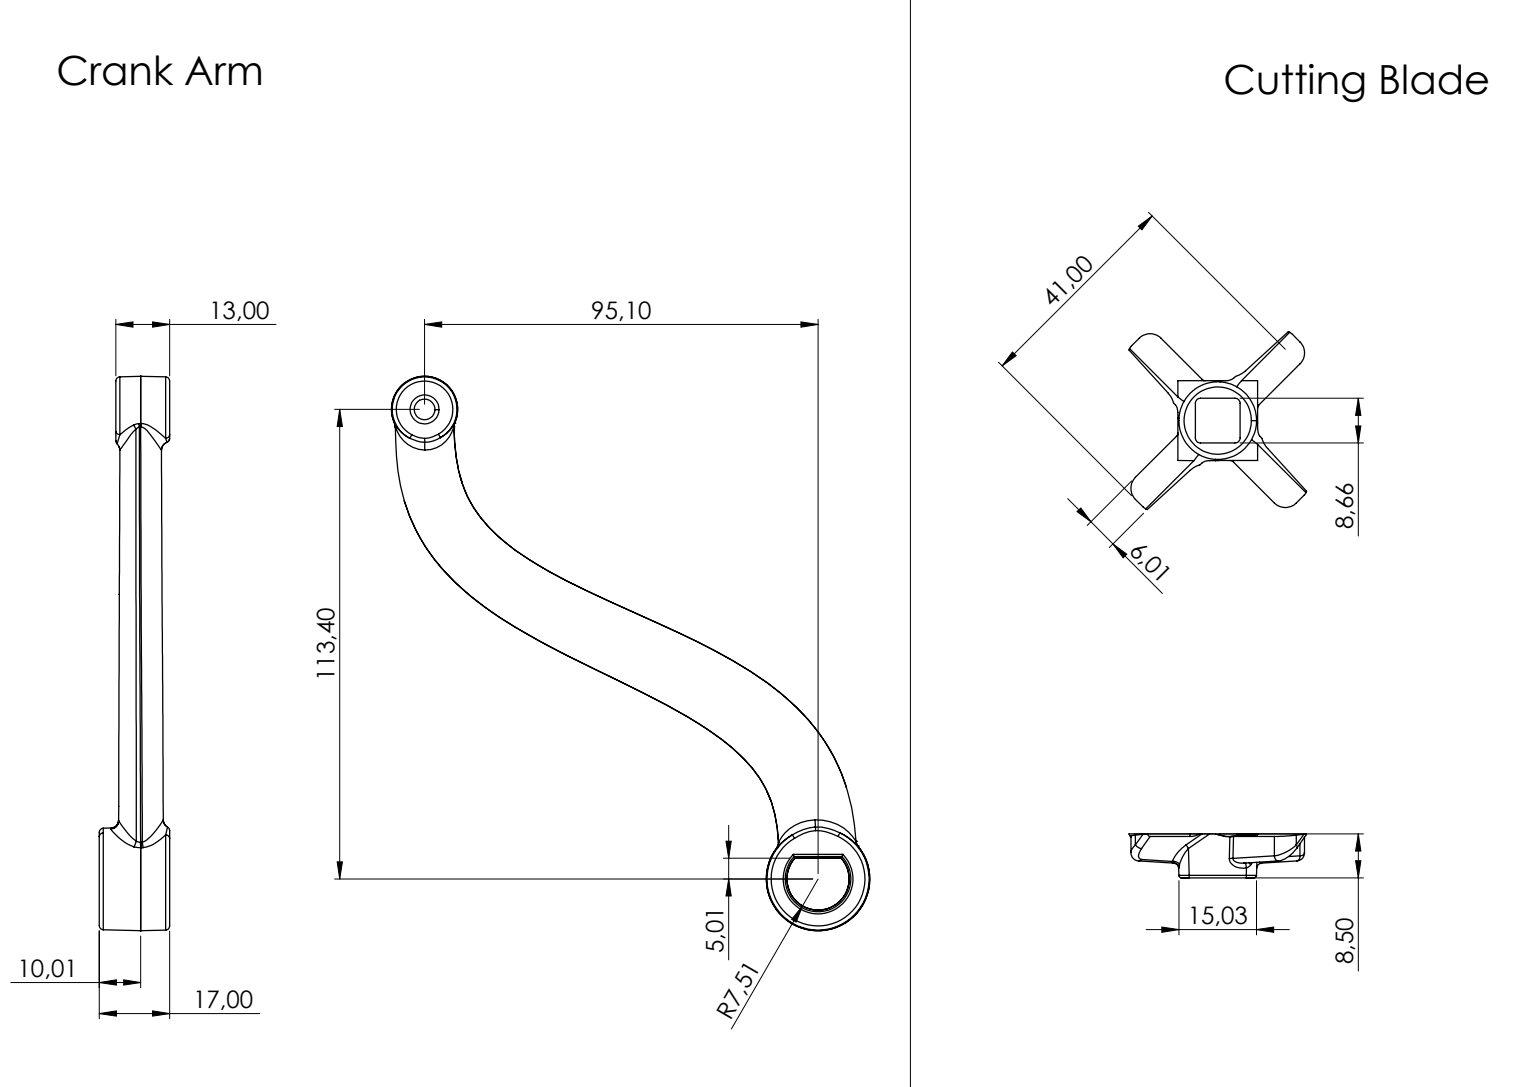
ISO-10303-21;
HEADER;
FILE_DESCRIPTION (('STEP AP214'),
    '1' );
FILE_NAME ('Cutting Blade.step',
    '2026-10-06T09:49:54',
    ( '' ),
    ( '' ),
    'SwSTEP 2.0',
    'SolidWorks 2020',
    '' );
FILE_SCHEMA (( 'AUTOMOTIVE_DESIGN' ));
ENDSEC;

DATA;
#16=CARTESIAN_POINT ( 'NONE',  ( 1.715361092244999996, 1516.743010792419909, 212.5670474586069929 ) ) ;
#21=B_SPLINE_CURVE_WITH_KNOTS ( 'NONE', 3,
 ( #95105, #62085, #88907, #54776, #87831, #29014 ),
 .UNSPECIFIED., .F., .F.,
 ( 4, 2, 4 ),
 ( 0.000000000000000000, 0.5000000000000000000, 1.000000000000000000 ),
 .UNSPECIFIED. ) ;
#54=CARTESIAN_POINT ( 'NONE',  ( -1.906561575282239904E-08, 1509.051704408389924, 204.1347675157070114 ) ) ;
#56=CARTESIAN_POINT ( 'NONE',  ( -6.391938843916317836, 1508.551704408389696, 216.1347674408802106 ) ) ;
#61=CARTESIAN_POINT ( 'NONE',  ( 2.477373605864999995, 1516.891731298979948, 206.2406231745169976 ) ) ;
#69=CARTESIAN_POINT ( 'NONE',  ( -16.59156838405375112, 1513.042027792487033, 221.1339923359998352 ) ) ;
#75=CARTESIAN_POINT ( 'NONE',  ( -5.770883602015000058, 1516.603620185149794, 211.4160555996369908 ) ) ;
#77=EDGE_CURVE ( 'NONE', #86690, #11573, #16701, .T. ) ;
#86=EDGE_CURVE ( 'NONE', #1893, #51148, #21, .T. ) ;
#111=CARTESIAN_POINT ( 'NONE',  ( 6.939219482805000005, 1516.783701990830195, 203.3409846960470020 ) ) ;
#112=CARTESIAN_POINT ( 'NONE',  ( 5.786847739675000213, 1517.104497701820037, 209.8595134730280165 ) ) ;
#115=CARTESIAN_POINT ( 'NONE',  ( 3.849857897463838885, 1511.509056589855390, 217.2694430494650248 ) ) ;
#143=AXIS2_PLACEMENT_3D ( 'NONE', #57309, #48343, #30414 ) ;
#150=CARTESIAN_POINT ( 'NONE',  ( -15.65821252386499829, 1513.518111364920060, 223.8216251916669819 ) ) ;
#156=CARTESIAN_POINT ( 'NONE',  ( -2.881222795715000284, 1516.891731298979948, 206.6444723262370076 ) ) ;
#179=CARTESIAN_POINT ( 'NONE',  ( -13.16128167722848552, 1513.520077403203913, 192.3341213175320092 ) ) ;
#180=EDGE_CURVE ( 'NONE', #17368, #18936, #5451, .T. ) ;
#186=DIRECTION ( 'NONE',  ( -1.000000000000000000, 0.000000000000000000, 0.000000000000000000 ) ) ;
#207=CARTESIAN_POINT ( 'NONE',  ( -5.006329619514999330, 1516.755758396839838, 202.5714564999769891 ) ) ;
#219=EDGE_CURVE ( 'NONE', #44996, #39203, #32843, .T. ) ;
#233=CARTESIAN_POINT ( 'NONE',  ( 7.300066962235000290, 1513.142795523620180, 201.9269575992269949 ) ) ;
#236=ORIENTED_EDGE ( 'NONE', *, *, #47228, .T. ) ;
#243=CARTESIAN_POINT ( 'NONE',  ( -7.886135186697788235, 1512.218159651028827, 212.0631589305448301 ) ) ;
#250=CARTESIAN_POINT ( 'NONE',  ( -4.043990345725000601, 1516.983612918759945, 206.6425990843970055 ) ) ;
#256=CARTESIAN_POINT ( 'NONE',  ( 7.213837368615000578, 1512.784460098860109, 215.9877155789269807 ) ) ;
#266=CARTESIAN_POINT ( 'NONE',  ( 7.720650135305000994, 1516.977993847330026, 214.9014730243169993 ) ) ;
#268=CARTESIAN_POINT ( 'NONE',  ( 6.161099242332739756, 1511.774605969369986, 217.7619246857520068 ) ) ;
#269=CARTESIAN_POINT ( 'NONE',  ( 7.260544162646080046, 1508.878901399440110, 215.8879859943839961 ) ) ;
#270=CARTESIAN_POINT ( 'NONE',  ( 3.268859396054999866, 1516.922519270759949, 211.5998327024669834 ) ) ;
#289=CARTESIAN_POINT ( 'NONE',  ( 2.482067860225000366, 1517.099836525840146, 203.3337487049469985 ) ) ;
#304=LINE ( 'NONE', #17034, #54663 ) ;
#309=CARTESIAN_POINT ( 'NONE',  ( -4.487249408019919450, 1509.038630944639863, 212.6094330731689865 ) ) ;
#315=DIRECTION ( 'NONE',  ( 0.2720708970484284062, 0.6839977328998089190, 0.6768489701308448847 ) ) ;
#316=CARTESIAN_POINT ( 'NONE',  ( -8.788316527315000570, 1511.741868877540128, 215.3741124244170067 ) ) ;
#323=VERTEX_POINT ( 'NONE', #26651 ) ;
#339=CARTESIAN_POINT ( 'NONE',  ( -5.441672317485815036, 1511.126521620285303, 201.4186169187619839 ) ) ;
#370=CARTESIAN_POINT ( 'NONE',  ( -1.703779643355000095, 1517.057265928030120, 213.1670284501570052 ) ) ;
#378=CARTESIAN_POINT ( 'NONE',  ( -3.264778817514999876, 1516.727068157269969, 204.1245957781970048 ) ) ;
#381=CARTESIAN_POINT ( 'NONE',  ( -1.569161292555000031, 1517.051704408389924, 216.8444262845069943 ) ) ;
#393=CARTESIAN_POINT ( 'NONE',  ( 0.7576635334400020350, 1516.855632454399938, 211.9899581013969794 ) ) ;
#398=CARTESIAN_POINT ( 'NONE',  ( -2.881325412095000260, 1517.003078582959688, 208.0029426616869728 ) ) ;
#414=CARTESIAN_POINT ( 'NONE',  ( -7.325541825264999751, 1516.710692850270107, 214.1269169785269924 ) ) ;
#417=CARTESIAN_POINT ( 'NONE',  ( -3.259729335964999919, 1517.119374999550018, 216.4589997383470177 ) ) ;
#444=CARTESIAN_POINT ( 'NONE',  ( -9.638115897704999213, 1520.551704408390151, 203.7504991310570119 ) ) ;
#449=CARTESIAN_POINT ( 'NONE',  ( -2.759740495412019712, 1516.551695078709827, 201.4123589199890034 ) ) ;
#455=ORIENTED_EDGE ( 'NONE', *, *, #105774, .T. ) ;
#493=CARTESIAN_POINT ( 'NONE',  ( 6.949703334655000120, 1517.130100026000036, 209.8609679372960102 ) ) ;
#502=CARTESIAN_POINT ( 'NONE',  ( -14.94819997777649867, 1513.870294663139930, 223.8775307694120045 ) ) ;
#510=CARTESIAN_POINT ( 'NONE',  ( -6.952166420425000659, 1517.213554313520035, 207.4130983078469797 ) ) ;
#525=CARTESIAN_POINT ( 'NONE',  ( -1.715361130375000043, 1516.743010792419909, 205.6766444437269854 ) ) ;
#543=LINE ( 'NONE', #53148, #67817 ) ;
#571=CARTESIAN_POINT ( 'NONE',  ( -3.254401441735000233, 1516.919782530640077, 213.1645757730269963 ) ) ;
#598=VERTEX_POINT ( 'NONE', #85321 ) ;
#605=DIRECTION ( 'NONE',  ( -1.000000000000000000, -6.997424008300000075E-18, -1.832339962680000039E-19 ) ) ;
#607=CARTESIAN_POINT ( 'NONE',  ( -5.385523200472070116, 1511.435001055929888, 200.4690698413500058 ) ) ;
#612=CARTESIAN_POINT ( 'NONE',  ( -3.461995196814999787, 1516.906233342200039, 206.2559344154570056 ) ) ;
#625=CARTESIAN_POINT ( 'NONE',  ( -1.700706814495000163, 1516.923170579120097, 211.4225755968969906 ) ) ;
#632=CARTESIAN_POINT ( 'NONE',  ( 3.052975896485000007, 1516.551704408390151, 217.1245693350269903 ) ) ;
#655=CARTESIAN_POINT ( 'NONE',  ( -4.618119704395000191, 1516.706638732659940, 202.1845071865270143 ) ) ;
#656=CARTESIAN_POINT ( 'NONE',  ( -6.556851034704999748, 1516.939568781210028, 209.1335575761840175 ) ) ;
#659=CARTESIAN_POINT ( 'NONE',  ( 4.264166330254295367, 1511.427938673519748, 217.4025041547218109 ) ) ;
#667=CARTESIAN_POINT ( 'NONE',  ( -0.4363688680027120181, 1517.051704408389924, 216.7663257121729998 ) ) ;
#671=VECTOR ( 'NONE', #63207, 1000.000000000000000 ) ;
#693=CARTESIAN_POINT ( 'NONE',  ( -15.60002308836500085, 1512.080583811389943, 221.9287863060669963 ) ) ;
#698=CARTESIAN_POINT ( 'NONE',  ( 7.708770007014999592, 1516.524310051880093, 206.8307984429870032 ) ) ;
#715=CARTESIAN_POINT ( 'NONE',  ( -2.385772222184999958, 1512.160709093490141, 201.5273412906769863 ) ) ;
#720=CARTESIAN_POINT ( 'NONE',  ( -7.500000019065006462, 1516.813460996586855, 209.5490843734590385 ) ) ;
#748=CARTESIAN_POINT ( 'NONE',  ( 4.031142351675000235, 1516.929569650079884, 204.1114229688670036 ) ) ;
#750=CARTESIAN_POINT ( 'NONE',  ( 15.09629032713499974, 1514.287526756679881, 193.8365223143670164 ) ) ;
#757=ORIENTED_EDGE ( 'NONE', *, *, #107789, .F. ) ;
#773=CARTESIAN_POINT ( 'NONE',  ( -4.027051443935000030, 1516.733363207009916, 211.6130343286269806 ) ) ;
#776=CARTESIAN_POINT ( 'NONE',  ( 7.248946776565000860, 1514.005261957179982, 201.2133402509770121 ) ) ;
#782=CARTESIAN_POINT ( 'NONE',  ( -8.664447134935000960, 1512.053281741910041, 215.6822705669570155 ) ) ;
#785=CARTESIAN_POINT ( 'NONE',  ( 7.717505752974999744, 1516.857914730730045, 216.8393517232070167 ) ) ;
#792=CARTESIAN_POINT ( 'NONE',  ( 3.446329775655000205, 1516.812046502680005, 206.2422037788969931 ) ) ;
#798=CARTESIAN_POINT ( 'NONE',  ( 7.665825164484999732, 1514.407352313670117, 214.8849219750870247 ) ) ;
#804=CARTESIAN_POINT ( 'NONE',  ( 7.487063056100070391, 1517.051702153270071, 209.5621714086410066 ) ) ;
#805=EDGE_CURVE ( 'NONE', #71147, #96332, #85826, .T. ) ;
#809=CARTESIAN_POINT ( 'NONE',  ( 0.7560907277860019482, 1516.770163853809890, 214.1221759657669850 ) ) ;
#814=CARTESIAN_POINT ( 'NONE',  ( 4.625359524845000792, 1517.025470194390209, 211.6020329869469947 ) ) ;
#824=TOROIDAL_SURFACE ( 'NONE', #91997, 6.500000000000000000, 1.000000000000000000 ) ;
#831=CARTESIAN_POINT ( 'NONE',  ( -4.039897316195000698, 1516.787536375099990, 204.1233307748069876 ) ) ;
#878=EDGE_CURVE ( 'NONE', #23166, #598, #93399, .T. ) ;
#892=ORIENTED_EDGE ( 'NONE', *, *, #53861, .T. ) ;
#899=DIRECTION ( 'NONE',  ( 0.9980966414074828874, 0.06164810140419229451, 0.001614312349211199796 ) ) ;
#915=CARTESIAN_POINT ( 'NONE',  ( -4.029572678834999699, 1516.858649670339901, 213.1633184439769764 ) ) ;
#918=EDGE_CURVE ( 'NONE', #68939, #6679, #17776, .T. ) ;
#923=CARTESIAN_POINT ( 'NONE',  ( 2.868433798504999910, 1517.020727862619879, 204.1095288638669842 ) ) ;
#926=CARTESIAN_POINT ( 'NONE',  ( -7.644479542047480258, 1517.051704408389924, 208.6854770967850072 ) ) ;
#938=CARTESIAN_POINT ( 'NONE',  ( 4.042729802795000715, 1516.919782530640077, 212.3762473738369749 ) ) ;
#943=CARTESIAN_POINT ( 'NONE',  ( 2.480427254505000345, 1516.872851364150165, 208.3639601402670110 ) ) ;
#960=CARTESIAN_POINT ( 'NONE',  ( 1.712644716155000024, 1516.636036526019780, 214.1174694231270053 ) ) ;
#963=CARTESIAN_POINT ( 'NONE',  ( -7.716878941104999612, 1516.833976295079992, 216.4517711926369827 ) ) ;
#990=EDGE_CURVE ( 'NONE', #18936, #89283, #17213, .T. ) ;
#997=CARTESIAN_POINT ( 'NONE',  ( -1.079555022276609932, 1516.642200982659915, 201.4099888424200060 ) ) ;
#1038=CARTESIAN_POINT ( 'NONE',  ( -7.601092437462869889, 1510.855104182140167, 214.7738715786570083 ) ) ;
#1045=CARTESIAN_POINT ( 'NONE',  ( -3.255809902135000211, 1516.837969789639828, 209.8792719553279937 ) ) ;
#1059=CARTESIAN_POINT ( 'NONE',  ( -0.7533003905399979772, 1516.992029636990083, 208.3816250717139837 ) ) ;
#1076=CARTESIAN_POINT ( 'NONE',  ( 2.477986732234999767, 1516.922519270759949, 205.8529865360470126 ) ) ;
#1123=CARTESIAN_POINT ( 'NONE',  ( -2.865911554774999814, 1516.906233342200039, 212.5838411289170153 ) ) ;
#1138=DIRECTION ( 'NONE',  ( -0.9147450530333530727, 0.03449475076686789321, 0.4025563316115395862 ) ) ;
#1154=EDGE_CURVE ( 'NONE', #30294, #42497, #37115, .T. ) ;
#1166=CARTESIAN_POINT ( 'NONE',  ( -6.563254928984999736, 1517.139039350860003, 206.6385234782069915 ) ) ;
#1173=CARTESIAN_POINT ( 'NONE',  ( 13.08147543293499915, 1513.492015765619954, 222.9104281842669764 ) ) ;
#1174=ORIENTED_EDGE ( 'NONE', *, *, #86900, .F. ) ;
#1179=CARTESIAN_POINT ( 'NONE',  ( -4.027697264044999947, 1516.766397346390022, 212.0005392193770035 ) ) ;
#1205=CARTESIAN_POINT ( 'NONE',  ( -4.037378294184999383, 1516.688761843659904, 202.5730239910470232 ) ) ;
#1206=CARTESIAN_POINT ( 'NONE',  ( 4.618583391875000110, 1516.939762005280045, 209.1087859301640322 ) ) ;
#1217=CARTESIAN_POINT ( 'NONE',  ( -0.4354997994421860308, 1517.051704408389924, 216.8053818660609977 ) ) ;
#1241=CARTESIAN_POINT ( 'NONE',  ( -15.56957305056499941, 1512.571022561239943, 222.6873122058669878 ) ) ;
#1245=CARTESIAN_POINT ( 'NONE',  ( -1.136004312195000088, 1516.815173273089840, 206.2562091229970065 ) ) ;
#1251=CARTESIAN_POINT ( 'NONE',  ( -10.25304834626500039, 1513.301704408390151, 214.4251468100669911 ) ) ;
#1262=CARTESIAN_POINT ( 'NONE',  ( -2.564633821555000193, 1511.308638870219966, 201.5496530815769916 ) ) ;
#1284=B_SPLINE_CURVE_WITH_KNOTS ( 'NONE', 3,
 ( #68712, #35081, #51899, #102816, #69263, #9338 ),
 .UNSPECIFIED., .F., .F.,
 ( 4, 2, 4 ),
 ( 1.219745810294720132E-06, 0.01184121947742510124, 0.02355703793478339941 ),
 .UNSPECIFIED. ) ;
#1293=FACE_OUTER_BOUND ( 'NONE', #104183, .T. ) ;
#1294=CARTESIAN_POINT ( 'NONE',  ( 2.480813884984999884, 1517.051603658920158, 204.1089070683270279 ) ) ;
#1296=CARTESIAN_POINT ( 'NONE',  ( 16.21240999383499570, 1514.452905717119847, 194.1945360481670093 ) ) ;
#1317=CARTESIAN_POINT ( 'NONE',  ( 6.950214933285000285, 1517.129577905929864, 211.9934263588270085 ) ) ;
#1320=CARTESIAN_POINT ( 'NONE',  ( 6.781132878754999815, 1512.686126173230150, 201.8548505242569888 ) ) ;
#1326=CARTESIAN_POINT ( 'NONE',  ( -7.084879081845000037, 1512.024017243139951, 216.0683601470269934 ) ) ;
#1327=CARTESIAN_POINT ( 'NONE',  ( 16.67556690833916022, 1513.118420042606658, 196.8779830456916216 ) ) ;
#1330=CARTESIAN_POINT ( 'NONE',  ( -6.554778571775000451, 1516.929962200689943, 216.8412383526069789 ) ) ;
#1337=EDGE_LOOP ( 'NONE', ( #26400, #72792, #8720, #28875, #102883, #62231 ) ) ;
#1338=CARTESIAN_POINT ( 'NONE',  ( -2.881222795715000284, 1516.891731298979948, 206.6444723262370076 ) ) ;
#1343=CARTESIAN_POINT ( 'NONE',  ( -7.203718089889590281, 1508.728103933889997, 202.3962606498199932 ) ) ;
#1353=AXIS2_PLACEMENT_3D ( 'NONE', #75150, #16294, #109298 ) ;
#1354=CARTESIAN_POINT ( 'NONE',  ( 7.719392382375000139, 1516.929962200689943, 215.6766245038770080 ) ) ;
#1358=CARTESIAN_POINT ( 'NONE',  ( -7.321193745875000047, 1516.534976163889951, 211.4135222436570132 ) ) ;
#1365=DIRECTION ( 'NONE',  ( -0.7384854939282339270, 4.128709092058512866E-17, 0.6742693640212139572 ) ) ;
#1374=CARTESIAN_POINT ( 'NONE',  ( -5.007588685045000432, 1516.804776704140068, 203.3466091393569855 ) ) ;
#1427=CARTESIAN_POINT ( 'NONE',  ( 7.522201442634911750, 1510.631883379783403, 203.2096215414982510 ) ) ;
#1448=CARTESIAN_POINT ( 'NONE',  ( 0.7564342142240020328, 1516.783665406140017, 213.7345173100169973 ) ) ;
#1449=CARTESIAN_POINT ( 'NONE',  ( 3.276907026574999993, 1511.440441732939917, 216.8388625892569905 ) ) ;
#1461=CARTESIAN_POINT ( 'NONE',  ( 2.288357407604999949, 1517.116049120239950, 203.3334095979369920 ) ) ;
#1479=CARTESIAN_POINT ( 'NONE',  ( -3.446329813785000251, 1516.812046502680005, 212.0014881234369852 ) ) ;
#1484=CARTESIAN_POINT ( 'NONE',  ( 3.255809864005000165, 1516.837969789639828, 208.3644199470059846 ) ) ;
#1494=B_SPLINE_CURVE_WITH_KNOTS ( 'NONE', 5,
 ( #71750, #95254, #20722, #61140, #62230, #54918 ),
 .UNSPECIFIED., .F., .F.,
 ( 6, 6 ),
 ( 0.000000000000000000, 1.000000000000000000 ),
 .UNSPECIFIED. ) ;
#1502=CARTESIAN_POINT ( 'NONE',  ( 3.262264650305000124, 1516.633288330999903, 215.6694029015669969 ) ) ;
#1514=CARTESIAN_POINT ( 'NONE',  ( 7.518184181947409783, 1510.874996213040049, 203.1087175251330166 ) ) ;
#1558=ADVANCED_FACE ( 'NONE', ( #55461 ), #67926, .T. ) ;
#1588=CARTESIAN_POINT ( 'NONE',  ( -7.713648872314999849, 1516.710624944440042, 209.8745175203999906 ) ) ;
#1606=CARTESIAN_POINT ( 'NONE',  ( -5.013429394184999666, 1517.123342927159911, 207.9998951881570122 ) ) ;
#1612=DIRECTION ( 'NONE',  ( -1.000000000000000000, 0.000000000000000000, 0.000000000000000000 ) ) ;
#1625=CARTESIAN_POINT ( 'NONE',  ( -6.949574985774999547, 1517.102359858469754, 205.8627441332170065 ) ) ;
#1628=CARTESIAN_POINT ( 'NONE',  ( -5.018135829431690453, 1516.818301249122669, 203.5289603568284065 ) ) ;
#1646=CARTESIAN_POINT ( 'NONE',  ( 6.946748518954999341, 1516.983995446890049, 214.1250666973070054 ) ) ;
#1673=CARTESIAN_POINT ( 'NONE',  ( 4.041472473744999405, 1516.858649670339901, 213.1514186109370144 ) ) ;
#1721=CARTESIAN_POINT ( 'NONE',  ( 2.282622912365000367, 1516.861367446839949, 206.8218623544969716 ) ) ;
#1735=CARTESIAN_POINT ( 'NONE',  ( 1.716392741775000008, 1516.788317650260069, 211.9856338259669997 ) ) ;
#1760=CARTESIAN_POINT ( 'NONE',  ( 5.513240533218949579, 1508.551563895499839, 201.9548267187850001 ) ) ;
#1764=CARTESIAN_POINT ( 'NONE',  ( -7.719392420504999741, 1516.929962200689943, 202.5670673984569703 ) ) ;
#1765=CARTESIAN_POINT ( 'NONE',  ( 0.01012488564660149991, 1516.989863902050047, 210.2497743036369968 ) ) ;
#1771=LINE ( 'NONE', #96358, #74990 ) ;
#1802=CARTESIAN_POINT ( 'NONE',  ( 11.25155670613500014, 1512.842772631639946, 225.3231501446670109 ) ) ;
#1806=CARTESIAN_POINT ( 'NONE',  ( -16.38335856736500062, 1512.258183966690012, 220.9924808180670084 ) ) ;
#1811=CARTESIAN_POINT ( 'NONE',  ( -5.012317106364999830, 1517.020727862619879, 206.2534121335969814 ) ) ;
#1816=DIRECTION ( 'NONE',  ( 0.000000000000000000, -1.000000000000000000, 3.531714064933559186E-16 ) ) ;
#1828=CARTESIAN_POINT ( 'NONE',  ( -2.229731647334999955, 1512.142919181319940, 201.5278066827870020 ) ) ;
#1831=CARTESIAN_POINT ( 'NONE',  ( 17.14950075666149587, 1517.051704408389924, 222.8506259189660170 ) ) ;
#1864=CARTESIAN_POINT ( 'NONE',  ( 7.324914918154999732, 1516.685667699390024, 204.5043554653269950 ) ) ;
#1886=CARTESIAN_POINT ( 'NONE',  ( -0.7355686809059980291, 1517.012231669750008, 212.3888856620870058 ) ) ;
#1893=VERTEX_POINT ( 'NONE', #110668 ) ;
#1894=VERTEX_POINT ( 'NONE', #27773 ) ;
#1900=CARTESIAN_POINT ( 'NONE',  ( 7.550503318189189628, 1510.480349263560129, 203.5706572562480119 ) ) ;
#1908=CARTESIAN_POINT ( 'NONE',  ( 5.771797426184999580, 1516.647618671360078, 206.2459958378869942 ) ) ;
#1911=AXIS2_PLACEMENT_3D ( 'NONE', #63244, #45873, #62132 ) ;
#1914=CARTESIAN_POINT ( 'NONE',  ( -6.766176630772359424, 1508.878902422570036, 201.8612697231370134 ) ) ;
#1920=CARTESIAN_POINT ( 'NONE',  ( -14.49568595290499928, 1514.921196705999819, 193.9190483465280010 ) ) ;
#1921=CARTESIAN_POINT ( 'NONE',  ( 17.05226155321927095, 1516.729020916208583, 222.6134475786040525 ) ) ;
#1925=CARTESIAN_POINT ( 'NONE',  ( 0.01289778877310149806, 1516.939723362869927, 214.1281058189269970 ) ) ;
#1927=CARTESIAN_POINT ( 'NONE',  ( 6.247704779676360509, 1510.876154134890157, 216.5661308656380015 ) ) ;
#1929=CARTESIAN_POINT ( 'NONE',  ( 2.493073829755000137, 1516.826109302209943, 211.9861720575370043 ) ) ;
#1938=PLANE ( 'NONE',  #73670 ) ;
#1946=CARTESIAN_POINT ( 'NONE',  ( 5.000083827734999709, 1516.858456333729919, 204.1129977322069919 ) ) ;
#1948=VECTOR ( 'NONE', #101539, 1000.000000000000114 ) ;
#1991=CARTESIAN_POINT ( 'NONE',  ( -5.004442077115000664, 1516.690345681169902, 201.4087281291169802 ) ) ;
#1995=CARTESIAN_POINT ( 'NONE',  ( 8.126234247455000670, 1514.923664147150021, 215.2485921136969864 ) ) ;
#2004=CARTESIAN_POINT ( 'NONE',  ( -8.463742342545000241, 1511.382391139620040, 213.9463409611770146 ) ) ;
#2018=ORIENTED_EDGE ( 'NONE', *, *, #878, .T. ) ;
#2023=CARTESIAN_POINT ( 'NONE',  ( 2.490245914424999985, 1516.691389976299888, 213.7302634767470124 ) ) ;
#2024=CARTESIAN_POINT ( 'NONE',  ( 4.036380747524999535, 1511.355055856609852, 217.1076883285369945 ) ) ;
#2025=AXIS2_PLACEMENT_3D ( 'NONE', #103889, #7617, #68656 ) ;
#2031=CARTESIAN_POINT ( 'NONE',  ( 5.000083827734999709, 1516.858456333729919, 204.1129977322069919 ) ) ;
#2046=CARTESIAN_POINT ( 'NONE',  ( 0.7574259850960020080, 1516.837969789639828, 212.3776558342370038 ) ) ;
#2051=CARTESIAN_POINT ( 'NONE',  ( 4.623892060624999800, 1517.066898074209803, 209.8584071487349831 ) ) ;
#2067=CARTESIAN_POINT ( 'NONE',  ( 2.487103419534999915, 1516.577434278289957, 215.6681487122470173 ) ) ;
#2078=CARTESIAN_POINT ( 'NONE',  ( 7.658720530103260593, 1511.445028088800200, 203.0218979614350019 ) ) ;
#2079=PRODUCT_DEFINITION_CONTEXT ( 'detailed design', #26278, 'design' ) ;
#2081=DIRECTION ( 'NONE',  ( 0.6742693640208961003, 0.000000000000000000, 0.7384854939285241393 ) ) ;
#2090=CARTESIAN_POINT ( 'NONE',  ( 6.520293444144174444, 1509.032998982614345, 201.8615402263750127 ) ) ;
#2105=EDGE_CURVE ( 'NONE', #33006, #74270, #109360, .T. ) ;
#2108=CARTESIAN_POINT ( 'NONE',  ( -1.951485868198830076, 1516.530904812869949, 201.4129032351939657 ) ) ;
#2156=ORIENTED_EDGE ( 'NONE', *, *, #106868, .F. ) ;
#2157=CARTESIAN_POINT ( 'NONE',  ( -1.122033430074999893, 1516.972341476009888, 209.8777854684929878 ) ) ;
#2161=VECTOR ( 'NONE', #110428, 1000.000000000000114 ) ;
#2174=CARTESIAN_POINT ( 'NONE',  ( 6.938478784765000462, 1516.719999691880048, 208.3679751968140010 ) ) ;
#2178=ORIENTED_EDGE ( 'NONE', *, *, #38568, .F. ) ;
#2184=CARTESIAN_POINT ( 'NONE',  ( 6.541070334811199594, 1517.051704644130041, 212.7912326336579838 ) ) ;
#2191=CARTESIAN_POINT ( 'NONE',  ( -7.336844680545000053, 1517.106845464700200, 205.6683011064770312 ) ) ;
#2210=CARTESIAN_POINT ( 'NONE',  ( -6.549762485114999144, 1516.729202374750002, 213.7405950387170037 ) ) ;
#2211=CARTESIAN_POINT ( 'NONE',  ( -4.329791528864999961, 1515.051704408389924, 212.4519801359869859 ) ) ;
#2228=CARTESIAN_POINT ( 'NONE',  ( 6.499999980935001531, 1516.051704408390151, 209.1218459511669892 ) ) ;
#2270=FACE_OUTER_BOUND ( 'NONE', #4358, .T. ) ;
#2285=CARTESIAN_POINT ( 'NONE',  ( -5.013274999515000552, 1517.068517094990057, 206.8347616620369820 ) ) ;
#2297=CARTESIAN_POINT ( 'NONE',  ( -3.445685115514999897, 1516.778761582560037, 211.6139765934069885 ) ) ;
#2307=CARTESIAN_POINT ( 'NONE',  ( 14.86633461655332233, 1514.624327954312776, 225.3233414037949842 ) ) ;
#2324=CARTESIAN_POINT ( 'NONE',  ( -1.130607502004999931, 1516.632821972880038, 202.5736453444569918 ) ) ;
#2325=CARTESIAN_POINT ( 'NONE',  ( -3.253301419385000504, 1516.790374942449944, 210.2573062871869922 ) ) ;
#2329=ORIENTED_EDGE ( 'NONE', *, *, #108317, .F. ) ;
#2346=CARTESIAN_POINT ( 'NONE',  ( -7.779264728704999854, 1514.199187793449937, 202.4059200890270063 ) ) ;
#2359=EDGE_CURVE ( 'NONE', #5115, #10547, #107935, .T. ) ;
#2371=CARTESIAN_POINT ( 'NONE',  ( -0.7576635715699989726, 1516.855632454399938, 206.2537338009369989 ) ) ;
#2373=DIRECTION ( 'NONE',  ( 0.000000000000000000, -1.000000000000000000, 6.123233995736769734E-17 ) ) ;
#2390=CARTESIAN_POINT ( 'NONE',  ( 5.857434645806802287, 1510.600498174433824, 216.6525474564166416 ) ) ;
#2404=EDGE_CURVE ( 'NONE', #19958, #1894, #81618, .T. ) ;
#2424=CARTESIAN_POINT ( 'NONE',  ( 7.323974606304999746, 1516.647924054489977, 205.0857262875869935 ) ) ;
#2446=CARTESIAN_POINT ( 'NONE',  ( 6.561995960394999550, 1517.083030555940013, 212.3803205491769859 ) ) ;
#2467=CARTESIAN_POINT ( 'NONE',  ( -7.338411997524999286, 1517.170512887980067, 206.6372682748769876 ) ) ;
#2473=CARTESIAN_POINT ( 'NONE',  ( -6.961854465055609786, 1508.551568319609714, 202.5699773954310103 ) ) ;
#2485=CARTESIAN_POINT ( 'NONE',  ( -6.552897405075000847, 1516.858146885269889, 215.6784973415170157 ) ) ;
#2489=CARTESIAN_POINT ( 'NONE',  ( -1.118903308544999975, 1517.003078582959688, 212.0031713441969998 ) ) ;
#2505=CARTESIAN_POINT ( 'NONE',  ( 4.612507273904999039, 1516.886345593249871, 204.1123678647870179 ) ) ;
#2521=CARTESIAN_POINT ( 'NONE',  ( -5.513435911474870110, 1508.551704408389924, 202.1089243664339961 ) ) ;
#2522=CIRCLE ( 'NONE', #40049, 5.000000000000000888 ) ;
#2545=DIRECTION ( 'NONE',  ( 0.000000000000000000, 1.000000000000000000, -6.123233995736769734E-17 ) ) ;
#2547=CARTESIAN_POINT ( 'NONE',  ( 3.259729297834999873, 1517.119374999550018, 201.7846921639870175 ) ) ;
#2562=CARTESIAN_POINT ( 'NONE',  ( -7.548380910495000151, 1510.399296111369949, 213.9269235281369959 ) ) ;
#2581=CARTESIAN_POINT ( 'NONE',  ( 0.01289778877310149806, 1516.939723362869927, 214.1281058189269970 ) ) ;
#2582=CARTESIAN_POINT ( 'NONE',  ( 2.933667421895000516, 1512.215430505229961, 217.0052628094269949 ) ) ;
#2587=CARTESIAN_POINT ( 'NONE',  ( 4.998515157294999511, 1516.787536375099990, 205.0819486540370065 ) ) ;
#2589=CARTESIAN_POINT ( 'NONE',  ( -3.415238448984999842, 1511.775527460079957, 205.7066075212470082 ) ) ;
#2590=CARTESIAN_POINT ( 'NONE',  ( 5.004475574535000248, 1517.026025493960105, 201.3999380438669959 ) ) ;
#2601=CARTESIAN_POINT ( 'NONE',  ( 4.043366220174999803, 1516.951766529250108, 211.9887038632370206 ) ) ;
#2607=CARTESIAN_POINT ( 'NONE',  ( 7.724874613184999461, 1517.139320148880188, 209.8621665372610039 ) ) ;
#2621=CARTESIAN_POINT ( 'NONE',  ( 0.01244693565920149993, 1516.939646076049939, 214.9034317483770167 ) ) ;
#2631=CARTESIAN_POINT ( 'NONE',  ( 7.899080318006880930, 1511.275365984429982, 203.5511717028010139 ) ) ;
#2639=DIRECTION ( 'NONE',  ( -0.6742693640212139572, -4.521919481779819710E-17, -0.7384854939282339270 ) ) ;
#2645=DIRECTION ( 'NONE',  ( -0.7071067811865492381, 0.000000000000000000, -0.7071067811865457964 ) ) ;
#2662=CARTESIAN_POINT ( 'NONE',  ( -2.000106894569579907, 1516.529320347400244, 201.4129447258819994 ) ) ;
#2706=CARTESIAN_POINT ( 'NONE',  ( 0.01012488564660149991, 1516.989863902050047, 210.2497743036369968 ) ) ;
#2708=B_SPLINE_CURVE_WITH_KNOTS ( 'NONE', 3,
 ( #29885, #55678, #22008, #65718, #23130, #6348, #29339, #63540, #97656, #20926, #49469, #60081, #25881, #23687, #57872, #109375, #68482, #179, #109911, #100404, #58416, #17468, #92002, #7447, #42158, #51118, #41045, #101480, #51669, #94197, #24231, #85805, #8538, #93634, #66287, #85242, #32652, #16369, #75223, #102583, #92542, #9103, #76310, #15276, #24768, #43270, #110460, #108807, #50567, #83589 ),
 .UNSPECIFIED., .F., .F.,
 ( 4, 2, 2, 1, 1, 2, 2, 2, 2, 1, 1, 1, 2, 2, 2, 2, 1, 1, 1, 2, 2, 2, 2, 1, 1, 1, 1, 2, 2, 2, 4 ),
 ( 0.000000000000000000, 0.1249999999987768118, 0.1874999999981652177, 0.2187499999978483323, 0.2343749999976874887, 0.2421874999976066367, 0.2499999999975258125, 0.3749999999967162934, 0.4374999999962853603, 0.4687499999960699770, 0.4843749999959355845, 0.4921874999958685826, 0.4960937499958351093, 0.4999999999958015806, 0.6249999999951432184, 0.6874999999948141483, 0.7187499999946499463, 0.7343749999945659024, 0.7421874999945267115, 0.7460937499945041740, 0.7499999999944817475, 0.8124999999947372098, 0.8437499999948295804, 0.8593749999948757656, 0.8671874999948987472, 0.8710937499949140683, 0.8730468749949186202, 0.8740234374949206186, 0.8749999999949225060, 0.9374999999974612530, 1.000000000000000000 ),
 .UNSPECIFIED. ) ;
#2712=EDGE_LOOP ( 'NONE', ( #76998, #67436, #41942, #17145, #20832, #42478, #88108, #19322, #74311 ) ) ;
#2720=VERTEX_POINT ( 'NONE', #85468 ) ;
#2722=CARTESIAN_POINT ( 'NONE',  ( 3.255809864005000165, 1516.837969789639828, 208.3644199470059846 ) ) ;
#2739=CARTESIAN_POINT ( 'NONE',  ( -2.493699806765000027, 1516.858326417339867, 206.6451124560869914 ) ) ;
#2749=CARTESIAN_POINT ( 'NONE',  ( -7.821732098484999618, 1513.613303996360173, 201.3872288444869980 ) ) ;
#2756=CARTESIAN_POINT ( 'NONE',  ( 3.456007385174999946, 1516.647534046129977, 215.6697273451470096 ) ) ;
#2758=ORIENTED_EDGE ( 'NONE', *, *, #78090, .T. ) ;
#2802=CARTESIAN_POINT ( 'NONE',  ( 7.599227146675000100, 1512.341036988540054, 206.8869224911269953 ) ) ;
#2820=CARTESIAN_POINT ( 'NONE',  ( -5.783578535681273003, 1516.788854543809975, 213.9010045776934419 ) ) ;
#2823=DIRECTION ( 'NONE',  ( -0.4770263929453174567, 0.7067418228236591604, -0.5224574779878943254 ) ) ;
#2825=CARTESIAN_POINT ( 'NONE',  ( 2.864326087304999824, 1516.826109302209943, 206.6287721023469999 ) ) ;
#2829=CARTESIAN_POINT ( 'NONE',  ( 15.20279577643499991, 1516.814170398969964, 225.0317485278669949 ) ) ;
#2836=CARTESIAN_POINT ( 'NONE',  ( 1.136004274065000041, 1516.815173273089840, 211.9874827793370287 ) ) ;
#2845=CARTESIAN_POINT ( 'NONE',  ( 11.97297233184965570, 1513.029502680773930, 225.6983645998317058 ) ) ;
#2847=ORIENTED_EDGE ( 'NONE', *, *, #49017, .T. ) ;
#2848=ORIENTED_EDGE ( 'NONE', *, *, #54124, .T. ) ;
#2856=CARTESIAN_POINT ( 'NONE',  ( 6.455447949027460552, 1508.551704612109916, 202.2941920603649919 ) ) ;
#2861=EDGE_CURVE ( 'NONE', #93671, #44996, #6366, .T. ) ;
#2864=VERTEX_POINT ( 'NONE', #72042 ) ;
#2865=CARTESIAN_POINT ( 'NONE',  ( 7.324914918154999732, 1516.685667699390024, 204.5043554653269950 ) ) ;
#2870=ORIENTED_EDGE ( 'NONE', *, *, #97880, .F. ) ;
#2891=CARTESIAN_POINT ( 'NONE',  ( -7.573276867445001059, 1513.355826799089755, 201.2778793177070042 ) ) ;
#2901=VERTEX_POINT ( 'NONE', #12649 ) ;
#2916=CARTESIAN_POINT ( 'NONE',  ( 2.863787855735000054, 1516.788317650260069, 207.4054531903269947 ) ) ;
#2935=CARTESIAN_POINT ( 'NONE',  ( 5.963459866581566793, 1510.663752950224307, 216.6350338863308309 ) ) ;
#2938=CARTESIAN_POINT ( 'NONE',  ( 17.10989499766859367, 1517.051704408389924, 222.9504516956734506 ) ) ;
#2956=ADVANCED_FACE ( 'NONE', ( #92651 ), #32751, .F. ) ;
#2972=CARTESIAN_POINT ( 'NONE',  ( 7.712490952985000980, 1516.666407245520077, 204.5049844236870058 ) ) ;
#2992=CARTESIAN_POINT ( 'NONE',  ( 6.561686423234999843, 1517.069378699710114, 212.5741351528070027 ) ) ;
#3003=CARTESIAN_POINT ( 'NONE',  ( -7.316722043595000002, 1511.382498894329956, 215.7022088808070066 ) ) ;
#3012=CARTESIAN_POINT ( 'NONE',  ( -4.811461170099283535, 1516.551188146009054, 218.2487618711105313 ) ) ;
#3014=CARTESIAN_POINT ( 'NONE',  ( 0.7350231981660010350, 1516.970035769810011, 206.8242163110469960 ) ) ;
#3025=CARTESIAN_POINT ( 'NONE',  ( 7.717505752974999744, 1516.857914730730045, 201.4043401791270185 ) ) ;
#3033=CARTESIAN_POINT ( 'NONE',  ( -3.259101837015000225, 1517.102359858469754, 216.0714209178769920 ) ) ;
#3037=CARTESIAN_POINT ( 'NONE',  ( 5.949235695344720298, 1511.655824793919919, 217.4114490419000276 ) ) ;
#3039=CARTESIAN_POINT ( 'NONE',  ( 2.492443650904999863, 1516.793978928989873, 212.3737347995770222 ) ) ;
#3040=CARTESIAN_POINT ( 'NONE',  ( 3.330134165755000097, 1515.051704408389924, 213.4516374609670208 ) ) ;
#3043=ORIENTED_EDGE ( 'NONE', *, *, #45218, .T. ) ;
#3055=ORIENTED_EDGE ( 'NONE', *, *, #108341, .F. ) ;
#3056=CARTESIAN_POINT ( 'NONE',  ( -2.877113108595000135, 1516.697242742309982, 204.1252037719370094 ) ) ;
#3069=AXIS2_PLACEMENT_3D ( 'NONE', #84795, #58524, #49027 ) ;
#3094=CARTESIAN_POINT ( 'NONE',  ( -12.61087486066499785, 1512.195694528090144, 194.0417079242670013 ) ) ;
#3097=CARTESIAN_POINT ( 'NONE',  ( -2.872700555325000238, 1516.559109716219837, 201.4121646638069763 ) ) ;
#3102=CARTESIAN_POINT ( 'NONE',  ( 7.575166919095000395, 1511.422242621320265, 206.4203055568870013 ) ) ;
#3106=ORIENTED_EDGE ( 'NONE', *, *, #105951, .T. ) ;
#3111=CARTESIAN_POINT ( 'NONE',  ( -7.848179713114999956, 1511.193640125469983, 213.6447370295169890 ) ) ;
#3132=CARTESIAN_POINT ( 'NONE',  ( -7.325541825264999751, 1516.710692850270107, 214.1269169785269924 ) ) ;
#3133=CARTESIAN_POINT ( 'NONE',  ( 4.813011385984999890, 1510.693074690949970, 216.6779200322870054 ) ) ;
#3138=CARTESIAN_POINT ( 'NONE',  ( -0.01322039564809850132, 1516.939819969850078, 205.0847949345169923 ) ) ;
#3141=CARTESIAN_POINT ( 'NONE',  ( 0.7403205670290020635, 1517.139320148880188, 201.3969713189170250 ) ) ;
#3153=CARTESIAN_POINT ( 'NONE',  ( -4.609996619675000851, 1516.769879638719885, 212.5810025483170023 ) ) ;
#3160=CARTESIAN_POINT ( 'NONE',  ( 0.7533003524100010395, 1516.992029636990083, 209.8620668306199946 ) ) ;
#3173=CARTESIAN_POINT ( 'NONE',  ( -5.777745433405000242, 1516.908489800550115, 215.6797558528670038 ) ) ;
#3179=CARTESIAN_POINT ( 'NONE',  ( 0.7403205670290020635, 1517.139320148880188, 201.3969713189170250 ) ) ;
#3188=CARTESIAN_POINT ( 'NONE',  ( 7.946349138541700441, 1511.532396045849964, 203.1959877047910084 ) ) ;
#3201=DIRECTION ( 'NONE',  ( 0.02616798426500965835, 0.9993150019883683122, -0.02616798426500970692 ) ) ;
#3202=CARTESIAN_POINT ( 'NONE',  ( 4.987078416414999715, 1508.551704408389924, 212.6094384009469707 ) ) ;
#3246=CARTESIAN_POINT ( 'NONE',  ( -7.500000019064998469, 1516.801704408389924, 209.1218459511669892 ) ) ;
#3258=CARTESIAN_POINT ( 'NONE',  ( 1.137296650804999976, 1516.908147884120126, 210.8236964273370120 ) ) ;
#3266=CARTESIAN_POINT ( 'NONE',  ( 5.778999773775000293, 1516.955859323880077, 201.7887757972170277 ) ) ;
#3272=CARTESIAN_POINT ( 'NONE',  ( 1.715109447055000125, 1516.963431999339946, 209.8570730874349977 ) ) ;
#3289=CARTESIAN_POINT ( 'NONE',  ( -2.299656354225000143, 1516.843453247299749, 206.6453952679669896 ) ) ;
#3290=VERTEX_POINT ( 'NONE', #37586 ) ;
#3306=DIRECTION ( 'NONE',  ( -1.000000000000000000, 0.000000000000000000, 0.000000000000000000 ) ) ;
#3308=CARTESIAN_POINT ( 'NONE',  ( 2.874588922665000545, 1516.606339319019980, 215.6687976528169770 ) ) ;
#3331=CYLINDRICAL_SURFACE ( 'NONE', #1911, 0.4999999999999909517 ) ;
#3350=ORIENTED_EDGE ( 'NONE', *, *, #99298, .F. ) ;
#3376=CARTESIAN_POINT ( 'NONE',  ( -0.01323705180209850014, 1516.939658295650133, 206.6356258303270010 ) ) ;
#3386=CARTESIAN_POINT ( 'NONE',  ( 8.753854055680109880, 1516.720891557477444, 213.2732902691849972 ) ) ;
#3397=CARTESIAN_POINT ( 'NONE',  ( 14.31751620109325174, 1514.209381233404883, 225.6439688837686504 ) ) ;
#3407=FACE_BOUND ( 'NONE', #58671, .T. ) ;
#3416=CARTESIAN_POINT ( 'NONE',  ( -3.264778817514999876, 1516.727068157269969, 204.1245957781970048 ) ) ;
#3436=CARTESIAN_POINT ( 'NONE',  ( -6.742834623714999864, 1512.383155430620036, 200.7463434866369880 ) ) ;
#3452=CARTESIAN_POINT ( 'NONE',  ( 14.12475443283500098, 1513.169116394660023, 224.4178625549669732 ) ) ;
#3461=CARTESIAN_POINT ( 'NONE',  ( 1.117840086735000016, 1516.949031626070109, 207.4047068479870006 ) ) ;
#3495=DIRECTION ( 'NONE',  ( -0.5224574779883525144, -0.7067418228232951183, 0.4770263929453549823 ) ) ;
#3502=EDGE_CURVE ( 'NONE', #33889, #21042, #75482, .T. ) ;
#3519=CARTESIAN_POINT ( 'NONE',  ( -2.490245952555000031, 1516.691389976299888, 204.5134284255869943 ) ) ;
#3541=CARTESIAN_POINT ( 'NONE',  ( 2.879956924955000108, 1516.827328999679821, 212.3743765858270081 ) ) ;
#3550=ORIENTED_EDGE ( 'NONE', *, *, #91361, .T. ) ;
#3564=CARTESIAN_POINT ( 'NONE',  ( 3.445201488374999954, 1516.743010792419909, 207.4064848398570291 ) ) ;
#3576=CYLINDRICAL_SURFACE ( 'NONE', #58477, 0.9999999999999522604 ) ;
#3583=CARTESIAN_POINT ( 'NONE',  ( -6.940473372275000052, 1516.833525648419936, 215.6778681647369922 ) ) ;
#3585=CARTESIAN_POINT ( 'NONE',  ( 6.048292005814400518, 1511.681069547209972, 217.7611486164249754 ) ) ;
#3587=CARTESIAN_POINT ( 'NONE',  ( -4.996642198295000448, 1516.697242742309982, 211.9989590406970024 ) ) ;
#3588=CARTESIAN_POINT ( 'NONE',  ( 3.915803383833039941, 1515.051704408389924, 213.4516362061017674 ) ) ;
#3605=CARTESIAN_POINT ( 'NONE',  ( -7.723480117524999855, 1517.086065052259983, 205.0863097070169943 ) ) ;
#3629=VECTOR ( 'NONE', #88330, 1000.000000000000227 ) ;
#3634=( BOUNDED_CURVE ( )  B_SPLINE_CURVE ( 3, ( #36275, #78848, #61504, #11632 ),
 .UNSPECIFIED., .F., .F. ) 
 B_SPLINE_CURVE_WITH_KNOTS ( ( 4, 4 ),
 ( 5.498282993746389735, 7.068394191937580118 ),
 .UNSPECIFIED. ) 
 CURVE ( )  GEOMETRIC_REPRESENTATION_ITEM ( )  RATIONAL_B_SPLINE_CURVE ( ( 1.000000000000000000, 0.8048993128220308657, 0.8048993128220308657, 1.000000000000000000 ) ) 
 REPRESENTATION_ITEM ( '' )  );
#3645=CARTESIAN_POINT ( 'NONE',  ( -14.49215846226499949, 1514.088841912139969, 192.6059998857670053 ) ) ;
#3650=CARTESIAN_POINT ( 'NONE',  ( 1.710012720495000194, 1517.232977404109988, 201.3945188173769907 ) ) ;
#3664=CARTESIAN_POINT ( 'NONE',  ( -7.556166249915000854, 1510.696675236759802, 213.5834717662970093 ) ) ;
#3667=AXIS2_PLACEMENT_3D ( 'NONE', #4462, #79519, #2823 ) ;
#3675=CARTESIAN_POINT ( 'NONE',  ( 15.90990255763500016, 1512.830284628050094, 198.1616908427670296 ) ) ;
#3685=CARTESIAN_POINT ( 'NONE',  ( 3.263521904354999670, 1516.676340709600026, 214.8942497445370066 ) ) ;
#3686=CARTESIAN_POINT ( 'NONE',  ( 3.165841356415000085, 1511.802450769970164, 217.0590624235869939 ) ) ;
#3691=CARTESIAN_POINT ( 'NONE',  ( -2.878693287274999957, 1516.766397346390022, 205.0941487061870134 ) ) ;
#3694=B_SPLINE_SURFACE_WITH_KNOTS ( 'NONE', 5, 5, ( 
 ( #309, #110587, #33873, #74800, #42284, #15953 ),
 ( #17600, #76434, #75890, #50686, #51800, #68609 ),
 ( #85939, #9242, #59652, #66412, #108943, #58000 ),
 ( #68064, #17038, #7027, #24898, #100529, #60203 ),
 ( #102177, #110040, #93760, #23808, #102712, #59105 ),
 ( #92134, #51235, #15409, #83732, #41184, #84283 ) ),
 .UNSPECIFIED., .F., .F., .F.,
 ( 6, 6 ),
 ( 6, 6 ),
 ( 4.250940516431700011, 7.082035122218299783 ),
 ( -9.670478295891639110E-06, 0.5000000000000000000 ),
 .UNSPECIFIED. ) ;
#3698=ORIENTED_EDGE ( 'NONE', *, *, #45621, .F. ) ;
#3704=CARTESIAN_POINT ( 'NONE',  ( 6.560742225334999844, 1517.028034847769959, 213.1554992345569701 ) ) ;
#3710=CARTESIAN_POINT ( 'NONE',  ( -1.709766532154999963, 1516.959716008189844, 209.1345041580460133 ) ) ;
#3719=CARTESIAN_POINT ( 'NONE',  ( 7.499999980935000643, 1516.801704408389924, 209.1218459511669892 ) ) ;
#3725=CARTESIAN_POINT ( 'NONE',  ( 2.488360629304999794, 1516.616791731099966, 214.8929950451170043 ) ) ;
#3729=VERTEX_POINT ( 'NONE', #70805 ) ;
#3730=CARTESIAN_POINT ( 'NONE',  ( -0.01126495432349849946, 1516.939530130779985, 202.1773791897269916 ) ) ;
#3735=CARTESIAN_POINT ( 'NONE',  ( 8.788267567532809466, 1511.742575854359984, 202.8686686809350022 ) ) ;
#3758=CARTESIAN_POINT ( 'NONE',  ( -7.495712400002839004, 1517.016242308364099, 208.8285887136074450 ) ) ;
#3764=CARTESIAN_POINT ( 'NONE',  ( -0.7983437007204670088, 1516.708834472140097, 201.4082439830900171 ) ) ;
#3769=CARTESIAN_POINT ( 'NONE',  ( 12.22498599127479935, 1512.125809830880144, 223.8828819965079902 ) ) ;
#3814=CARTESIAN_POINT ( 'NONE',  ( -5.770820179264999794, 1516.591755933730155, 210.8331571987770019 ) ) ;
#3822=EDGE_CURVE ( 'NONE', #89306, #3290, #97423, .T. ) ;
#3823=CARTESIAN_POINT ( 'NONE',  ( 3.259729297834999873, 1517.119374999550018, 201.7846921639870175 ) ) ;
#3838=AXIS2_PLACEMENT_3D ( 'NONE', #66963, #14317, #56898 ) ;
#3844=CARTESIAN_POINT ( 'NONE',  ( -1.136004312195000088, 1516.815173273089840, 206.2562091229970065 ) ) ;
#3852=CARTESIAN_POINT ( 'NONE',  ( 6.372167600494999640, 1511.069621805459974, 216.5183910133270047 ) ) ;
#3860=CARTESIAN_POINT ( 'NONE',  ( -4.612507312034999529, 1516.886345593249871, 214.1313240375470173 ) ) ;
#3862=ORIENTED_EDGE ( 'NONE', *, *, #70755, .F. ) ;
#3879=DIRECTION ( 'NONE',  ( 0.7063774289747313251, 0.04540766091858271930, -0.7063774289747313251 ) ) ;
#3881=CARTESIAN_POINT ( 'NONE',  ( -5.513435705061030312, 1509.038615938849944, 201.6090957135359929 ) ) ;
#3890=CARTESIAN_POINT ( 'NONE',  ( -4.554962026871971048, 1508.731359868796062, 212.6094325583298712 ) ) ;
#3928=CARTESIAN_POINT ( 'NONE',  ( -0.7579263249019989601, 1516.927039499179955, 207.4176752179770347 ) ) ;
#3949=CARTESIAN_POINT ( 'NONE',  ( 14.77683004841523307, 1514.552098284236536, 225.3854720466699462 ) ) ;
#3967=CARTESIAN_POINT ( 'NONE',  ( 1.121383591734999907, 1517.104192383289956, 204.4960559556369901 ) ) ;
#3987=CARTESIAN_POINT ( 'NONE',  ( -6.658917469454999960, 1512.371207877090001, 200.8892782097470047 ) ) ;
#4000=CARTESIAN_POINT ( 'NONE',  ( 13.86270800413499948, 1513.875858217480072, 225.8871191791669730 ) ) ;
#4008=CARTESIAN_POINT ( 'NONE',  ( -2.494758036134999912, 1516.937508036699910, 207.4208181092269854 ) ) ;
#4019=CYLINDRICAL_SURFACE ( 'NONE', #68164, 0.9999999999999985567 ) ;
#4026=CARTESIAN_POINT ( 'NONE',  ( 6.288919081391354027, 1510.947107034761302, 216.5507387054137496 ) ) ;
#4063=CARTESIAN_POINT ( 'NONE',  ( 4.028630584655000568, 1516.812923327049930, 205.6617440802170051 ) ) ;
#4070=ORIENTED_EDGE ( 'NONE', *, *, #85135, .F. ) ;
#4091=ORIENTED_EDGE ( 'NONE', *, *, #25305, .T. ) ;
#4092=CARTESIAN_POINT ( 'NONE',  ( -6.715925881185000001, 1514.199187793469946, 216.9011106608170110 ) ) ;
#4093=CARTESIAN_POINT ( 'NONE',  ( 16.20149547506775534, 1514.624327907797579, 194.2555113716582582 ) ) ;
#4104=CARTESIAN_POINT ( 'NONE',  ( 7.321193707744999557, 1516.534976163889951, 206.8301696586770220 ) ) ;
#4121=CARTESIAN_POINT ( 'NONE',  ( 0.7538707352880020807, 1516.719999691880048, 216.0603247549969979 ) ) ;
#4123=DIRECTION ( 'NONE',  ( 0.8236474686107853049, -0.5669078173018522460, 0.01484500364079644613 ) ) ;
#4125=CARTESIAN_POINT ( 'NONE',  ( 6.561995960394999550, 1517.083030555940013, 212.3803205491769859 ) ) ;
#4143=CARTESIAN_POINT ( 'NONE',  ( -6.559798094425000059, 1516.987478262539980, 204.5068286042669854 ) ) ;
#4165=CARTESIAN_POINT ( 'NONE',  ( 8.389588760568322812, 1511.399594748087793, 204.5238464867746302 ) ) ;
#4170=ADVANCED_FACE ( 'NONE', ( #109599 ), #49705, .T. ) ;
#4175=CARTESIAN_POINT ( 'NONE',  ( -12.07722023366500075, 1511.957228877180114, 194.2728863314669923 ) ) ;
#4177=CARTESIAN_POINT ( 'NONE',  ( 2.872208710164999790, 1517.145312756229941, 201.7840522196070197 ) ) ;
#4181=CARTESIAN_POINT ( 'NONE',  ( 7.684243075114999932, 1511.930588878439949, 206.3551010095970071 ) ) ;
#4188=CARTESIAN_POINT ( 'NONE',  ( -4.487249791936469556, 1509.038615938009798, 212.6094384014929801 ) ) ;
#4189=CARTESIAN_POINT ( 'NONE',  ( -4.616861546623686863, 1516.666407247929328, 201.4093550276068072 ) ) ;
#4206=VERTEX_POINT ( 'NONE', #57562 ) ;
#4214=CARTESIAN_POINT ( 'NONE',  ( -5.775236830874999505, 1516.804776704140068, 214.1294346171470124 ) ) ;
#4221=CARTESIAN_POINT ( 'NONE',  ( -1.713317447804999949, 1516.660388280709867, 204.5138242629670060 ) ) ;
#4234=CARTESIAN_POINT ( 'NONE',  ( -6.935457963315000640, 1516.627618683580067, 212.5772239474869991 ) ) ;
#4239=CARTESIAN_POINT ( 'NONE',  ( -7.714148301377419692, 1516.729697371079965, 209.8385372711610160 ) ) ;
#4240=EDGE_CURVE ( 'NONE', #49508, #63015, #65316, .T. ) ;
#4241=CARTESIAN_POINT ( 'NONE',  ( 5.786847739675000213, 1517.104497701820037, 209.8595134730280165 ) ) ;
#4257=CARTESIAN_POINT ( 'NONE',  ( 3.261635932824999973, 1516.613881697390070, 216.0569793506570022 ) ) ;
#4262=CARTESIAN_POINT ( 'NONE',  ( 7.716878902974999122, 1516.833976295079992, 201.7919207096969672 ) ) ;
#4263=CARTESIAN_POINT ( 'NONE',  ( -14.84895963876499891, 1511.957228877180114, 221.1990661657670216 ) ) ;
#4265=CARTESIAN_POINT ( 'NONE',  ( -15.91746622356501462, 1512.594959757389915, 220.0895646873669875 ) ) ;
#4288=EDGE_CURVE ( 'NONE', #37685, #65412, #87722, .T. ) ;
#4300=CARTESIAN_POINT ( 'NONE',  ( 0.04106552329005089957, 1516.946282269519997, 201.4020272027410101 ) ) ;
#4302=ORIENTED_EDGE ( 'NONE', *, *, #103432, .F. ) ;
#4304=CARTESIAN_POINT ( 'NONE',  ( 13.70533112961760125, 1512.850289816029772, 224.4308539454270033 ) ) ;
#4306=ORIENTED_EDGE ( 'NONE', *, *, #42966, .T. ) ;
#4345=CARTESIAN_POINT ( 'NONE',  ( 3.462948796544999652, 1516.956048353049937, 211.4063724288770061 ) ) ;
#4354=CARTESIAN_POINT ( 'NONE',  ( 2.291514297774999598, 1517.194972660189933, 201.3955140066269962 ) ) ;
#4358=EDGE_LOOP ( 'NONE', ( #50228, #35588, #67697, #74405 ) ) ;
#4370=CARTESIAN_POINT ( 'NONE',  ( 0.7559394982620020187, 1516.972341476009888, 210.2438793621770117 ) ) ;
#4375=CARTESIAN_POINT ( 'NONE',  ( 7.717016619025000246, 1511.440441732939917, 205.8449389055269876 ) ) ;
#4377=CARTESIAN_POINT ( 'NONE',  ( 4.995994787574999485, 1516.665179208830068, 206.6322283937570035 ) ) ;
#4378=ORIENTED_EDGE ( 'NONE', *, *, #31531, .F. ) ;
#4379=LINE ( 'NONE', #98415, #97351 ) ;
#4396=CARTESIAN_POINT ( 'NONE',  ( -6.939219520934999608, 1516.783701990830195, 214.9027072062869763 ) ) ;
#4397=ORIENTED_EDGE ( 'NONE', *, *, #51664, .F. ) ;
#4398=CARTESIAN_POINT ( 'NONE',  ( 7.708877363402839578, 1516.528409826940106, 206.8600011716279994 ) ) ;
#4428=CARTESIAN_POINT ( 'NONE',  ( -4.487249791936469556, 1509.038615938009798, 212.6094384014929801 ) ) ;
#4440=CARTESIAN_POINT ( 'NONE',  ( 3.487585849186794817, 1508.611350403810775, 213.8000011204408963 ) ) ;
#4453=CARTESIAN_POINT ( 'NONE',  ( -7.507423057800870048, 1508.880864719049896, 215.2619752906269923 ) ) ;
#4462=CARTESIAN_POINT ( 'NONE',  ( -5.242935297045000276, 1514.496907775670024, 217.7778693727470056 ) ) ;
#4464=CARTESIAN_POINT ( 'NONE',  ( 4.026614479655000522, 1516.699825673279975, 207.4075116849170115 ) ) ;
#4485=CARTESIAN_POINT ( 'NONE',  ( 14.16490606602967084, 1514.105081316843780, 225.7087563701193460 ) ) ;
#4493=CARTESIAN_POINT ( 'NONE',  ( 4.369728359379250193, 1508.879004046169939, 205.0024669094390219 ) ) ;
#4501=CARTESIAN_POINT ( 'NONE',  ( 4.612507273904999039, 1516.886345593249871, 204.1123678647870179 ) ) ;
#4507=ORIENTED_EDGE ( 'NONE', *, *, #75832, .F. ) ;
#4512=CARTESIAN_POINT ( 'NONE',  ( -14.35493914170010044, 1513.426431439620046, 193.9549492499340033 ) ) ;
#4523=CARTESIAN_POINT ( 'NONE',  ( -7.466890204824999877, 1513.600111798330090, 202.4729951676269764 ) ) ;
#4537=CARTESIAN_POINT ( 'NONE',  ( 11.87063484783499945, 1512.258183966700017, 225.5052044994669700 ) ) ;
#4543=CARTESIAN_POINT ( 'NONE',  ( 2.282622912365000367, 1516.861367446839949, 206.8218623544969716 ) ) ;
#4584=CARTESIAN_POINT ( 'NONE',  ( 3.487592431604999987, 1508.551704408389924, 204.1347675156769981 ) ) ;
#4591=CARTESIAN_POINT ( 'NONE',  ( -3.385932610363147077, 1511.683921178999071, 201.1181467729594203 ) ) ;
#4598=CARTESIAN_POINT ( 'NONE',  ( -4.041472511874999896, 1516.858649670339901, 205.0922732913970208 ) ) ;
#4612=CARTESIAN_POINT ( 'NONE',  ( -4.612671377915000370, 1516.783665406140017, 209.8782801844560026 ) ) ;
#4627=CARTESIAN_POINT ( 'NONE',  ( -6.390054486374999954, 1513.333000339850059, 216.6179291409569885 ) ) ;
#4637=CARTESIAN_POINT ( 'NONE',  ( 7.708770007014999592, 1516.524310051880093, 206.8307984429870032 ) ) ;
#4642=ORIENTED_EDGE ( 'NONE', *, *, #48019, .F. ) ;
#4648=CARTESIAN_POINT ( 'NONE',  ( -5.910253173700709795, 1511.600194708689969, 200.4926261112069881 ) ) ;
#4654=CARTESIAN_POINT ( 'NONE',  ( 5.005700201405000271, 1516.732530461250008, 216.0598116305469887 ) ) ;
#4658=CARTESIAN_POINT ( 'NONE',  ( 2.419940912470191829, 1516.533504771425442, 216.8308567494544832 ) ) ;
#4659=CARTESIAN_POINT ( 'NONE',  ( 3.266349474065000091, 1516.797038924770050, 213.1501537103870021 ) ) ;
#4667=EDGE_CURVE ( 'NONE', #106739, #71879, #51778, .T. ) ;
#4677=CARTESIAN_POINT ( 'NONE',  ( 6.547881374914999775, 1516.647534046129977, 205.6658385469270058 ) ) ;
#4700=CARTESIAN_POINT ( 'NONE',  ( 7.924501696547047835, 1511.889619706852500, 206.0091653069858069 ) ) ;
#4706=CARTESIAN_POINT ( 'NONE',  ( -7.513187957268617545, 1510.663752939659162, 215.0853058208080313 ) ) ;
#4709=CARTESIAN_POINT ( 'NONE',  ( -11.59188839696499862, 1512.902436350919970, 192.6803903701670038 ) ) ;
#4712=CARTESIAN_POINT ( 'NONE',  ( -1.708721022705000037, 1516.531533746980131, 201.8006767011069940 ) ) ;
#4746=CARTESIAN_POINT ( 'NONE',  ( -5.001338666445000136, 1516.911981270829983, 214.9058546054269812 ) ) ;
#4754=CARTESIAN_POINT ( 'NONE',  ( 0.7360974386200019870, 1517.045004075700035, 205.0794574309270217 ) ) ;
#4767=CARTESIAN_POINT ( 'NONE',  ( -7.323034312095000331, 1516.609912606490070, 212.5765947784269940 ) ) ;
#4772=CARTESIAN_POINT ( 'NONE',  ( 4.625789976465000564, 1517.104192383289956, 210.2432295619669844 ) ) ;
#4785=CARTESIAN_POINT ( 'NONE',  ( -2.484577695354999616, 1517.170512887980067, 216.4602579296269766 ) ) ;
#4790=CARTESIAN_POINT ( 'NONE',  ( -3.261007169695000041, 1516.596789218710001, 201.7991362452670216 ) ) ;
#4797=CARTESIAN_POINT ( 'NONE',  ( 8.488400859335269999, 1511.451532973539770, 203.7397716954870077 ) ) ;
#4811=FACE_OUTER_BOUND ( 'NONE', #61858, .T. ) ;
#4824=CARTESIAN_POINT ( 'NONE',  ( 0.02465969127001850156, 1516.941612417570013, 201.4021494659330074 ) ) ;
#4829=CARTESIAN_POINT ( 'NONE',  ( 13.03156809012940087, 1512.406412987999829, 224.3505518485380037 ) ) ;
#4873=CARTESIAN_POINT ( 'NONE',  ( 7.339749335215000059, 1517.224900789629828, 210.8312305431869902 ) ) ;
#4875=CARTESIAN_POINT ( 'NONE',  ( 3.461360093275000160, 1516.874084700499907, 212.3753080308970311 ) ) ;
#4883=CARTESIAN_POINT ( 'NONE',  ( -3.261007169695000041, 1516.596789218710001, 201.7991362452670216 ) ) ;
#4884=DIRECTION ( 'NONE',  ( 0.6742693640212154005, 0.000000000000000000, 0.7384854939282328168 ) ) ;
#4898=CARTESIAN_POINT ( 'NONE',  ( -5.775625115495000017, 1516.745833913490060, 209.8771724060850090 ) ) ;
#4904=CARTESIAN_POINT ( 'NONE',  ( 7.548872300095000654, 1510.418062979259958, 203.9404357814470075 ) ) ;
#4906=( BOUNDED_CURVE ( )  B_SPLINE_CURVE ( 3, ( #98180, #56187, #20910, #55115 ),
 .UNSPECIFIED., .F., .F. ) 
 B_SPLINE_CURVE_WITH_KNOTS ( ( 4, 4 ),
 ( 4.424142070125560267, 5.579787944456629845 ),
 .UNSPECIFIED. ) 
 CURVE ( )  GEOMETRIC_REPRESENTATION_ITEM ( )  RATIONAL_B_SPLINE_CURVE ( ( 1.000000000000000000, 0.8917691661789544089, 0.8917691661789544089, 1.000000000000000000 ) ) 
 REPRESENTATION_ITEM ( '' )  );
#4907=CARTESIAN_POINT ( 'NONE',  ( -4.625359562974999506, 1517.025470194390209, 206.6416589153869836 ) ) ;
#4922=CARTESIAN_POINT ( 'NONE',  ( 5.006329581384999727, 1516.755758396839838, 215.6722354023569892 ) ) ;
#4924=CARTESIAN_POINT ( 'NONE',  ( 7.710967333700570414, 1516.608222572569957, 207.8710650191239893 ) ) ;
#4925=CARTESIAN_POINT ( 'NONE',  ( -7.889297536996000559, 1517.051704408390378, 206.4074150262267722 ) ) ;
#4933=CARTESIAN_POINT ( 'NONE',  ( 2.234923440975000286, 1512.341036988540054, 216.7210731169070073 ) ) ;
#4946=VECTOR ( 'NONE', #52550, 1000.000000000000114 ) ;
#4951=CARTESIAN_POINT ( 'NONE',  ( -4.538868782924999401, 1511.336728379370243, 201.0216414995070124 ) ) ;
#4967=DIRECTION ( 'NONE',  ( 0.02616798426500960631, -0.9993150019883682011, -0.02616798426500960631 ) ) ;
#4995=CARTESIAN_POINT ( 'NONE',  ( -7.727327152855000492, 1517.232977404109988, 207.4118332116069894 ) ) ;
#5011=CARTESIAN_POINT ( 'NONE',  ( 7.565983030562289713, 1517.051704408389924, 209.5600921240870207 ) ) ;
#5036=CARTESIAN_POINT ( 'NONE',  ( -6.557909920764999789, 1516.908489800550115, 203.3441005368270282 ) ) ;
#5043=CARTESIAN_POINT ( 'NONE',  ( 4.554961988741982992, 1508.731359868795835, 205.6342593440040503 ) ) ;
#5045=CARTESIAN_POINT ( 'NONE',  ( -14.75568483658040009, 1513.870294662259994, 194.1736459919410152 ) ) ;
#5057=CARTESIAN_POINT ( 'NONE',  ( -7.743766119884999632, 1514.370494773840164, 202.8627129457869955 ) ) ;
#5070=CARTESIAN_POINT ( 'NONE',  ( 14.37690900153499918, 1514.216506490359961, 225.6932579665669891 ) ) ;
#5110=CIRCLE ( 'NONE', #99897, 1.000000000000059064 ) ;
#5115=VERTEX_POINT ( 'NONE', #95839 ) ;
#5118=DIRECTION ( 'NONE',  ( -0.8236474686107847498, 0.5669078173018529121, -0.01484500364079613562 ) ) ;
#5127=CARTESIAN_POINT ( 'NONE',  ( -2.957486053519140956, 1512.146863357693292, 201.2343373090091347 ) ) ;
#5136=CARTESIAN_POINT ( 'NONE',  ( 2.285487581364999965, 1517.001127920769704, 205.0775242521070254 ) ) ;
#5151=CARTESIAN_POINT ( 'NONE',  ( 2.881325373965000214, 1517.003078582959688, 210.2407492406470055 ) ) ;
#5164=CARTESIAN_POINT ( 'NONE',  ( -5.706397885535000825, 1514.325389163589989, 216.7730352073269842 ) ) ;
#5165=CARTESIAN_POINT ( 'NONE',  ( 16.31974134803240872, 1514.485057798524167, 194.4298416830750682 ) ) ;
#5171=CARTESIAN_POINT ( 'NONE',  ( -3.487592469391230132, 1509.038615938009798, 204.6345961782960217 ) ) ;
#5174=CARTESIAN_POINT ( 'NONE',  ( -2.258825589925000266, 1511.942942747529969, 201.5330432499970073 ) ) ;
#5180=CARTESIAN_POINT ( 'NONE',  ( 3.255809864005000165, 1516.837969789639828, 208.3644199470059846 ) ) ;
#5191=CARTESIAN_POINT ( 'NONE',  ( -5.652025646554889704, 1510.855104182140167, 201.5207535327680262 ) ) ;
#5193=CARTESIAN_POINT ( 'NONE',  ( -6.178095865712184498, 1510.835436358435118, 201.6599032209836082 ) ) ;
#5199=VECTOR ( 'NONE', #47929, 1000.000000000000000 ) ;
#5200=CARTESIAN_POINT ( 'NONE',  ( -5.778999811904999895, 1516.955859323880077, 216.4549161051170074 ) ) ;
#5206=CARTESIAN_POINT ( 'NONE',  ( -5.772727946874999461, 1516.691414181030041, 212.5791125756269935 ) ) ;
#5218=B_SPLINE_CURVE_WITH_KNOTS ( 'NONE', 5,
 ( #98225, #73606, #22587, #29913, #39979, #56237 ),
 .UNSPECIFIED., .F., .F.,
 ( 6, 6 ),
 ( 4.250950522270000143, 7.082025451739999866 ),
 .UNSPECIFIED. ) ;
#5225=CARTESIAN_POINT ( 'NONE',  ( -1.714334285315000095, 1516.699825673279975, 205.0952314524469955 ) ) ;
#5254=( BOUNDED_CURVE ( )  B_SPLINE_CURVE ( 3, ( #58994, #16391, #50586, #84716 ),
 .UNSPECIFIED., .F., .T. ) 
 B_SPLINE_CURVE_WITH_KNOTS ( ( 4, 4 ),
 ( 0.5395807524025459934, 1.539014399144550405 ),
 .UNSPECIFIED. ) 
 CURVE ( )  GEOMETRIC_REPRESENTATION_ITEM ( )  RATIONAL_B_SPLINE_CURVE ( ( 1.000000000000000000, 0.9184788592068002799, 0.9184788592068002799, 1.000000000000000000 ) ) 
 REPRESENTATION_ITEM ( '' )  );
#5261=CARTESIAN_POINT ( 'NONE',  ( -7.550503362009299835, 1510.480349264700180, 214.6730346447039892 ) ) ;
#5264=CARTESIAN_POINT ( 'NONE',  ( -11.75640701316500092, 1511.791180387469922, 193.9413991097669907 ) ) ;
#5266=CARTESIAN_POINT ( 'NONE',  ( -6.942973667334999988, 1516.833844030519913, 201.7931697622170191 ) ) ;
#5269=CARTESIAN_POINT ( 'NONE',  ( 15.90990255763500016, 1512.830284628050094, 198.1616908427670296 ) ) ;
#5293=CARTESIAN_POINT ( 'NONE',  ( 7.380526832584999752, 1511.503799556579906, 202.6426608137470282 ) ) ;
#5303=CARTESIAN_POINT ( 'NONE',  ( 0.7538707352880020807, 1516.719999691880048, 216.0603247549969979 ) ) ;
#5311=CARTESIAN_POINT ( 'NONE',  ( 4.997573787194999895, 1516.742629295279812, 205.6633194342169872 ) ) ;
#5313=CARTESIAN_POINT ( 'NONE',  ( 4.037050997585000189, 1516.939819969850078, 209.1086255745840106 ) ) ;
#5317=CARTESIAN_POINT ( 'NONE',  ( 6.527830543224999893, 1512.220794350770120, 216.8989209840169963 ) ) ;
#5325=CARTESIAN_POINT ( 'NONE',  ( 5.785582913545000316, 1516.981965530290154, 213.1542438721070027 ) ) ;
#5330=CARTESIAN_POINT ( 'NONE',  ( -7.708877905894440552, 1516.528429087750055, 211.1705659669590034 ) ) ;
#5331=CARTESIAN_POINT ( 'NONE',  ( 4.045182479925000685, 1517.057265928030120, 210.8256255754569963 ) ) ;
#5343=CARTESIAN_POINT ( 'NONE',  ( 7.550503318189189628, 1510.480349263560129, 203.5706572562480119 ) ) ;
#5346=CARTESIAN_POINT ( 'NONE',  ( -1.125509888415000104, 1517.203017563489766, 216.4609531728469847 ) ) ;
#5351=CARTESIAN_POINT ( 'NONE',  ( -6.942344729965000738, 1516.810037859429940, 201.4055938791270250 ) ) ;
#5353=VERTEX_POINT ( 'NONE', #67760 ) ;
#5358=CARTESIAN_POINT ( 'NONE',  ( 7.551708674585110082, 1510.523965798400013, 203.3918062713489974 ) ) ;
#5375=AXIS2_PLACEMENT_3D ( 'NONE', #34462, #94922, #43974 ) ;
#5380=CARTESIAN_POINT ( 'NONE',  ( -13.72878287234173555, 1517.051704408389924, 226.2713469440930112 ) ) ;
#5386=CARTESIAN_POINT ( 'NONE',  ( -0.4165852338731970139, 1516.813354641049955, 201.4055070984510110 ) ) ;
#5390=CARTESIAN_POINT ( 'NONE',  ( 14.92122229814569856, 1514.080593477150160, 223.9397791912049911 ) ) ;
#5410=ADVANCED_FACE ( 'NONE', ( #101873 ), #50955, .F. ) ;
#5431=CARTESIAN_POINT ( 'NONE',  ( 2.494757998004999866, 1516.937508036699910, 210.8228737931069929 ) ) ;
#5434=CARTESIAN_POINT ( 'NONE',  ( -7.323034312095000331, 1516.609912606490070, 212.5765947784269940 ) ) ;
#5440=CARTESIAN_POINT ( 'NONE',  ( 5.778372563615000068, 1516.932669162149978, 202.1763558832970205 ) ) ;
#5451=LINE ( 'NONE', #23883, #107492 ) ;
#5452=CARTESIAN_POINT ( 'NONE',  ( -3.669386717783980068, 1517.051704642929963, 215.6629163041010031 ) ) ;
#5455=CARTESIAN_POINT ( 'NONE',  ( 2.493697040924999886, 1516.977201124959947, 210.2401991861970032 ) ) ;
#5460=CARTESIAN_POINT ( 'NONE',  ( 8.558300736974999268, 1511.397837225850026, 204.0148718853070022 ) ) ;
#5461=CARTESIAN_POINT ( 'NONE',  ( 5.770820141135000192, 1516.591755933730155, 207.4105347035570048 ) ) ;
#5473=CARTESIAN_POINT ( 'NONE',  ( 7.627638999635267147, 1513.425324099864838, 215.5670651928058703 ) ) ;
#5477=CARTESIAN_POINT ( 'NONE',  ( 4.987078416394999714, 1508.551704408389924, 209.1218459511669892 ) ) ;
#5479=CARTESIAN_POINT ( 'NONE',  ( -7.715625241105000143, 1516.786099423779888, 215.6766101314970001 ) ) ;
#5481=CARTESIAN_POINT ( 'NONE',  ( 7.709070221419720426, 1516.535774777470124, 206.6432696383980101 ) ) ;
#5494=B_SPLINE_SURFACE_WITH_KNOTS ( 'NONE', 5, 5, ( 
 ( #3735, #88267, #86601, #12101, #44063, #2078, #36758, #45737, #35646 ),
 ( #46295, #80422, #18829, #37867, #3188, #11560, #78201, #37316, #27252 ),
 ( #61434, #97205, #53024, #103382, #61990, #54139, #10449, #1514, #44622 ),
 ( #71511, #53585, #105630, #28915, #78763, #104511, #105067, #96106, #19381 ),
 ( #26687, #36208, #27806, #87731, #2631, #11009, #45180, #73122, #5358 ),
 ( #99399, #4797, #22124, #65286, #5917, #107819, #99953, #89907, #38942 ) ),
 .UNSPECIFIED., .F., .F., .F.,
 ( 6, 6 ),
 ( 6, 3, 6 ),
 ( 4.238752792101340816, 5.659133035208659734 ),
 ( 0.000000000000000000, 0.5000000000000000000, 1.002061266618659907 ),
 .UNSPECIFIED. ) ;
#5507=AXIS2_PLACEMENT_3D ( 'NONE', #74613, #107651, #66229 ) ;
#5525=ORIENTED_EDGE ( 'NONE', *, *, #219, .F. ) ;
#5526=EDGE_CURVE ( 'NONE', #51148, #42643, #78925, .T. ) ;
#5529=FACE_OUTER_BOUND ( 'NONE', #43506, .T. ) ;
#5545=CARTESIAN_POINT ( 'NONE',  ( -7.512750272569109988, 1509.038617475950105, 214.6350457578409987 ) ) ;
#5560=CARTESIAN_POINT ( 'NONE',  ( 2.477975315464999717, 1516.839862955080207, 207.9852983471170091 ) ) ;
#5588=ORIENTED_EDGE ( 'NONE', *, *, #102639, .F. ) ;
#5594=ORIENTED_EDGE ( 'NONE', *, *, #22009, .T. ) ;
#5598=CARTESIAN_POINT ( 'NONE',  ( 2.866857893004999713, 1516.951766529250108, 205.0784797119270024 ) ) ;
#5603=ORIENTED_EDGE ( 'NONE', *, *, #74145, .F. ) ;
#5606=CYLINDRICAL_SURFACE ( 'NONE', #96725, 2.999999999999995115 ) ;
#5607=CARTESIAN_POINT ( 'NONE',  ( -13.18795888012849993, 1512.495155157840145, 193.8533315336999863 ) ) ;
#5623=CARTESIAN_POINT ( 'NONE',  ( -5.614653854145000622, 1512.956339156650074, 214.7364997862470091 ) ) ;
#5633=CARTESIAN_POINT ( 'NONE',  ( 14.45097768893499968, 1514.857962383129916, 224.3693530530669875 ) ) ;
#5647=VECTOR ( 'NONE', #2639, 1000.000000000000114 ) ;
#5687=PLANE ( 'NONE',  #110541 ) ;
#5688=SURFACE_SIDE_STYLE ('',( #90215 ) ) ;
#5702=CARTESIAN_POINT ( 'NONE',  ( -2.879642191334999879, 1516.812046502680005, 205.6755161564470313 ) ) ;
#5716=CARTESIAN_POINT ( 'NONE',  ( 7.339749335215000059, 1517.224900789629828, 210.8312305431869902 ) ) ;
#5730=CARTESIAN_POINT ( 'NONE',  ( -5.986375141904999531, 1514.050458741980037, 216.7582919984769774 ) ) ;
#5744=CARTESIAN_POINT ( 'NONE',  ( 7.716878902974999122, 1516.833976295079992, 201.7919207096969672 ) ) ;
#5745=CARTESIAN_POINT ( 'NONE',  ( 0.7402208603880020554, 1516.992029636990083, 208.3685455796920110 ) ) ;
#5759=CARTESIAN_POINT ( 'NONE',  ( -5.912224502460420084, 1510.631883423287263, 201.5996445015462371 ) ) ;
#5764=CARTESIAN_POINT ( 'NONE',  ( 2.291676273424999799, 1516.534976163889951, 216.4430396779769978 ) ) ;
#5769=CARTESIAN_POINT ( 'NONE',  ( 1.135185044044999980, 1516.778853242349896, 212.5689744308569971 ) ) ;
#5790=CARTESIAN_POINT ( 'NONE',  ( -6.948321743994999800, 1517.049325831759916, 205.0875650164470017 ) ) ;
#5818=CARTESIAN_POINT ( 'NONE',  ( 7.508706873624496403, 1508.884207225577484, 203.6084103738515978 ) ) ;
#5831=CARTESIAN_POINT ( 'NONE',  ( 1.125509850285000280, 1517.203017563489766, 201.7827387294869936 ) ) ;
#5835=CARTESIAN_POINT ( 'NONE',  ( 15.19327421213499996, 1512.300546902530186, 196.2658363013669884 ) ) ;
#5847=CARTESIAN_POINT ( 'NONE',  ( -7.618904794935000169, 1511.873873588870083, 211.7469127400270281 ) ) ;
#5860=ORIENTED_EDGE ( 'NONE', *, *, #36766, .F. ) ;
#5865=CARTESIAN_POINT ( 'NONE',  ( -6.553524415734999664, 1516.882690742909972, 216.0660777183969969 ) ) ;
#5871=CARTESIAN_POINT ( 'NONE',  ( 7.710610402995000001, 1516.594591938570147, 205.6677260153969939 ) ) ;
#5873=CARTESIAN_POINT ( 'NONE',  ( -3.255809902135000211, 1516.837969789639828, 209.8792719553279937 ) ) ;
#5884=CARTESIAN_POINT ( 'NONE',  ( -5.774609660074999873, 1516.777260590120022, 213.7418541773069762 ) ) ;
#5888=CARTESIAN_POINT ( 'NONE',  ( -7.714725160980429486, 1516.751726750540229, 209.7571990288649886 ) ) ;
#5889=CARTESIAN_POINT ( 'NONE',  ( 4.626591867355000609, 1517.096587378560116, 210.8266407735670214 ) ) ;
#5904=CARTESIAN_POINT ( 'NONE',  ( 6.555393117025000826, 1516.809497469189864, 216.4498952504870033 ) ) ;
#5909=CARTESIAN_POINT ( 'NONE',  ( 4.615644804385000022, 1517.009964551830080, 202.1744681489270192 ) ) ;
#5917=CARTESIAN_POINT ( 'NONE',  ( 7.866724121416869941, 1511.219705715099963, 203.6977230978289981 ) ) ;
#5946=CARTESIAN_POINT ( 'NONE',  ( 14.56186259785490122, 1513.645442088340133, 224.1908963721469945 ) ) ;
#5956=CARTESIAN_POINT ( 'NONE',  ( 13.82860585633196848, 1517.051704408389924, 192.0119494921260639 ) ) ;
#5982=CARTESIAN_POINT ( 'NONE',  ( -4.995994825704999975, 1516.665179208830068, 211.6114635085770033 ) ) ;
#5985=CARTESIAN_POINT ( 'NONE',  ( 6.949265646015000186, 1517.089216728169959, 212.5747629931370000 ) ) ;
#5991=CARTESIAN_POINT ( 'NONE',  ( 6.552897366944999469, 1516.858146885269889, 202.5651945608169910 ) ) ;
#6006=CARTESIAN_POINT ( 'NONE',  ( 1.136814033864999907, 1516.854133554269993, 211.4058994415870245 ) ) ;
#6011=CARTESIAN_POINT ( 'NONE',  ( 7.556074062054999985, 1510.693074690949970, 204.3088345461070219 ) ) ;
#6012=CARTESIAN_POINT ( 'NONE',  ( 2.282622912365000367, 1516.861367446839949, 206.8218623544969716 ) ) ;
#6030=CARTESIAN_POINT ( 'NONE',  ( -7.328676208015000526, 1516.833844030519913, 216.0648195994369871 ) ) ;
#6034=CARTESIAN_POINT ( 'NONE',  ( -7.722580352398438208, 1517.051704408390378, 206.9393828551336583 ) ) ;
#6061=CARTESIAN_POINT ( 'NONE',  ( -3.991161821394999976, 1511.207707629420156, 201.3372867307170111 ) ) ;
#6063=CARTESIAN_POINT ( 'NONE',  ( -5.556349349672759175, 1511.457792576462907, 200.4111309786675577 ) ) ;
#6085=DIRECTION ( 'NONE',  ( 1.000000000000000000, 0.000000000000000000, 0.000000000000000000 ) ) ;
#6095=CARTESIAN_POINT ( 'NONE',  ( -7.395102162025949610, 1511.068351247050032, 215.4971964518929894 ) ) ;
#6100=CARTESIAN_POINT ( 'NONE',  ( 3.447128460625000113, 1516.778853242349896, 207.9866608880570027 ) ) ;
#6124=CARTESIAN_POINT ( 'NONE',  ( 4.364199090702369332, 1509.032029411810072, 205.0059829744700153 ) ) ;
#6133=CARTESIAN_POINT ( 'NONE',  ( -6.947377821305000367, 1517.009964551830080, 204.5062011277169916 ) ) ;
#6136=CARTESIAN_POINT ( 'NONE',  ( 15.05672294932299948, 1512.222316757829958, 196.4963374934199862 ) ) ;
#6142=CARTESIAN_POINT ( 'NONE',  ( -12.89209534591269879, 1512.335564144490036, 193.9409293534239964 ) ) ;
#6157=EDGE_LOOP ( 'NONE', ( #35933, #103858, #3055, #67312 ) ) ;
#6219=( BOUNDED_CURVE ( )  B_SPLINE_CURVE ( 3, ( #76193, #110340, #33612, #67809 ),
 .UNSPECIFIED., .F., .F. ) 
 B_SPLINE_CURVE_WITH_KNOTS ( ( 4, 4 ),
 ( 0.5395807523979880838, 1.539014399141934941 ),
 .UNSPECIFIED. ) 
 CURVE ( )  GEOMETRIC_REPRESENTATION_ITEM ( )  RATIONAL_B_SPLINE_CURVE ( ( 1.000000000000000000, 0.9184788592064899726, 0.9184788592064899726, 1.000000000000000000 ) ) 
 REPRESENTATION_ITEM ( '' )  );
#6226=CARTESIAN_POINT ( 'NONE',  ( -2.994327866758245804, 1512.053565093312500, 201.2273685530865919 ) ) ;
#6233=CARTESIAN_POINT ( 'NONE',  ( 4.610938211375000151, 1516.815231249920089, 205.0813186281270077 ) ) ;
#6251=CARTESIAN_POINT ( 'NONE',  ( 4.626591867355000609, 1517.096587378560116, 210.8266407735670214 ) ) ;
#6280=ORIENTED_EDGE ( 'NONE', *, *, #25623, .T. ) ;
#6281=CARTESIAN_POINT ( 'NONE',  ( 3.259101798884999734, 1517.102359858469754, 202.1722709844570147 ) ) ;
#6282=CARTESIAN_POINT ( 'NONE',  ( -0.01012492377659850000, 1516.989863902050047, 207.9939175986969815 ) ) ;
#6294=CARTESIAN_POINT ( 'NONE',  ( -6.092700172539130321, 1510.714321716110135, 201.6274141883939990 ) ) ;
#6297=CARTESIAN_POINT ( 'NONE',  ( -6.054581406427221424, 1510.727597940411670, 201.6275102438071372 ) ) ;
#6302=CARTESIAN_POINT ( 'NONE',  ( 1.128757561074999805, 1516.608208975040043, 216.8328129478670121 ) ) ;
#6308=CARTESIAN_POINT ( 'NONE',  ( -0.7360974767499980365, 1517.045004075700035, 213.1642344714070134 ) ) ;
#6316=CARTESIAN_POINT ( 'NONE',  ( -3.330134203884999700, 1515.051704408389924, 204.7920544413669859 ) ) ;
#6325=CARTESIAN_POINT ( 'NONE',  ( -1.135460355084999762, 1516.790374942449944, 205.8685445508469911 ) ) ;
#6348=CARTESIAN_POINT ( 'NONE',  ( -11.80664835635214516, 1512.979863700403257, 192.6170353444451564 ) ) ;
#6355=CARTESIAN_POINT ( 'NONE',  ( 7.512750207965000371, 1509.038615934239942, 203.6084103740869864 ) ) ;
#6366=( BOUNDED_CURVE ( )  B_SPLINE_CURVE ( 3, ( #28347, #71501, #28904, #29436 ),
 .UNSPECIFIED., .F., .F. ) 
 B_SPLINE_CURVE_WITH_KNOTS ( ( 4, 4 ),
 ( 1.971460695176299183, 2.757092281751130525 ),
 .UNSPECIFIED. ) 
 CURVE ( )  GEOMETRIC_REPRESENTATION_ITEM ( )  RATIONAL_B_SPLINE_CURVE ( ( 1.000000000000000000, 0.9492232417517829646, 0.9492232417517829646, 1.000000000000000000 ) ) 
 REPRESENTATION_ITEM ( '' )  );
#6373=CARTESIAN_POINT ( 'NONE',  ( -0.01126495432349849946, 1516.939530130779985, 202.1773791897269916 ) ) ;
#6374=CARTESIAN_POINT ( 'NONE',  ( -8.704319915738482294, 1511.459876705991064, 214.6724670380187945 ) ) ;
#6376=CARTESIAN_POINT ( 'NONE',  ( 15.16677552193500134, 1513.509764667529907, 194.6542904276670072 ) ) ;
#6381=ORIENTED_EDGE ( 'NONE', *, *, #92600, .F. ) ;
#6402=CARTESIAN_POINT ( 'NONE',  ( 8.297002879045001222, 1511.752511073100095, 203.0778258940270007 ) ) ;
#6411=CARTESIAN_POINT ( 'NONE',  ( 2.292940169014999974, 1516.565291103010168, 215.6678853655270132 ) ) ;
#6417=CARTESIAN_POINT ( 'NONE',  ( 6.445219222570445439, 1513.425324099854834, 201.4942069324724514 ) ) ;
#6421=CARTESIAN_POINT ( 'NONE',  ( 4.028630584655000568, 1516.812923327049930, 205.6617440802170051 ) ) ;
#6423=CARTESIAN_POINT ( 'NONE',  ( 7.719640903004999721, 1516.939452820819952, 209.1117431028050078 ) ) ;
#6426=CARTESIAN_POINT ( 'NONE',  ( 6.658917431355000360, 1512.371207877119787, 217.3544136925769976 ) ) ;
#6435=CARTESIAN_POINT ( 'NONE',  ( 7.334328272665000092, 1517.005755693489846, 214.1256940922069987 ) ) ;
#6440=CARTESIAN_POINT ( 'NONE',  ( -7.709297277558810890, 1516.544444245480008, 210.8523772776020166 ) ) ;
#6441=CARTESIAN_POINT ( 'NONE',  ( -0.7352271553329990939, 1516.963431999339946, 210.8369554172870153 ) ) ;
#6454=CARTESIAN_POINT ( 'NONE',  ( 2.292307230374999616, 1516.548716157039962, 216.0554627912370051 ) ) ;
#6459=CARTESIAN_POINT ( 'NONE',  ( 7.715625202974999652, 1516.786099423779888, 202.5670817708370066 ) ) ;
#6460=CARTESIAN_POINT ( 'NONE',  ( -16.76527324706500011, 1513.875858217480072, 222.9845539743670031 ) ) ;
#6461=CARTESIAN_POINT ( 'NONE',  ( 5.513435558014999849, 1509.038615934239942, 216.6345961781970288 ) ) ;
#6532=CARTESIAN_POINT ( 'NONE',  ( 7.725990161824999980, 1517.181921232829836, 211.6070516194370157 ) ) ;
#6536=CARTESIAN_POINT ( 'NONE',  ( 1.135185044044999980, 1516.778853242349896, 212.5689744308569971 ) ) ;
#6545=CARTESIAN_POINT ( 'NONE',  ( -6.556022232634999725, 1516.833525648419936, 202.1813725979570222 ) ) ;
#6560=CARTESIAN_POINT ( 'NONE',  ( -6.546001388695000145, 1516.557392317769882, 210.8318505190270002 ) ) ;
#6566=CARTESIAN_POINT ( 'NONE',  ( 7.321169230994999388, 1516.531533746980131, 207.4131249475269954 ) ) ;
#6573=ORIENTED_EDGE ( 'NONE', *, *, #60296, .T. ) ;
#6585=CARTESIAN_POINT ( 'NONE',  ( -2.483949978725000118, 1517.156142772249950, 216.0726795003369887 ) ) ;
#6587=CARTESIAN_POINT ( 'NONE',  ( 7.718696897759629749, 1516.903402714960066, 209.0140334714870107 ) ) ;
#6612=CARTESIAN_POINT ( 'NONE',  ( -3.853756162035000266, 1510.775363762149937, 201.5636160667770014 ) ) ;
#6616=CARTESIAN_POINT ( 'NONE',  ( -14.11150871393421724, 1517.034034075904401, 226.0802419627609368 ) ) ;
#6640=LINE ( 'NONE', #91743, #85039 ) ;
#6649=CARTESIAN_POINT ( 'NONE',  ( -8.298113379911610465, 1511.753545947210114, 215.1666516095260135 ) ) ;
#6654=CARTESIAN_POINT ( 'NONE',  ( -7.337297350114999617, 1517.135701590510052, 208.3821536943570152 ) ) ;
#6667=EDGE_CURVE ( 'NONE', #51820, #65412, #80948, .T. ) ;
#6679=VERTEX_POINT ( 'NONE', #110000 ) ;
#6687=CARTESIAN_POINT ( 'NONE',  ( -3.802992233161490265, 1508.880967439349888, 204.6292016850710240 ) ) ;
#6689=CARTESIAN_POINT ( 'NONE',  ( 5.772727908745000747, 1516.691414181030041, 205.6645793267070133 ) ) ;
#6693=CARTESIAN_POINT ( 'NONE',  ( 15.13723819610809862, 1513.497693042470019, 194.6975888916769861 ) ) ;
#6698=CARTESIAN_POINT ( 'NONE',  ( -14.21962194668809865, 1513.293387711960122, 193.9060419221420091 ) ) ;
#6745=FACE_OUTER_BOUND ( 'NONE', #93919, .T. ) ;
#6770=CARTESIAN_POINT ( 'NONE',  ( -4.982688954091917921, 1511.399508273119864, 200.6046720606312306 ) ) ;
#6776=CARTESIAN_POINT ( 'NONE',  ( -2.879956963085000154, 1516.827328999679821, 205.8693153165069702 ) ) ;
#6780=ORIENTED_EDGE ( 'NONE', *, *, #73025, .F. ) ;
#6788=CARTESIAN_POINT ( 'NONE',  ( -16.01537990865516292, 1514.821748405528524, 224.2191644384507754 ) ) ;
#6792=CARTESIAN_POINT ( 'NONE',  ( -1.117840124865000062, 1516.949031626070109, 210.8389850543470061 ) ) ;
#6813=CARTESIAN_POINT ( 'NONE',  ( -3.487586626227472841, 1508.731359868795380, 204.5668839433602386 ) ) ;
#6820=CARTESIAN_POINT ( 'NONE',  ( -0.01126495432349849946, 1516.939530130779985, 202.1773791897269916 ) ) ;
#6821=CARTESIAN_POINT ( 'NONE',  ( 7.713648834184999359, 1516.710624944440042, 208.3691743819339877 ) ) ;
#6843=CARTESIAN_POINT ( 'NONE',  ( 1.220352910582999995, 1516.613788747029275, 216.8329590593428975 ) ) ;
#6844=CARTESIAN_POINT ( 'NONE',  ( 1.715361092244999996, 1516.743010792419909, 212.5670474586069929 ) ) ;
#6862=CARTESIAN_POINT ( 'NONE',  ( 6.547556931335000385, 1516.633288330999903, 205.8595812817970057 ) ) ;
#6869=ADVANCED_FACE ( 'NONE', ( #93185 ), #60826, .F. ) ;
#6903=ORIENTED_EDGE ( 'NONE', *, *, #97405, .F. ) ;
#6906=CARTESIAN_POINT ( 'NONE',  ( -7.550614507920475837, 1510.484595328588057, 214.6890571836817969 ) ) ;
#6910=CARTESIAN_POINT ( 'NONE',  ( -15.20279857216500119, 1514.921193539169963, 193.2119409213669883 ) ) ;
#6913=EDGE_CURVE ( 'NONE', #72650, #43618, #16563, .T. ) ;
#6916=CARTESIAN_POINT ( 'NONE',  ( -2.873329398885000163, 1516.572193931679976, 201.7997408644770019 ) ) ;
#6919=CARTESIAN_POINT ( 'NONE',  ( 16.88678280943500098, 1513.362623229679912, 196.1895945485670154 ) ) ;
#6943=CARTESIAN_POINT ( 'NONE',  ( 8.207084954655000431, 1512.038636172079805, 202.7922115676269925 ) ) ;
#6952=CARTESIAN_POINT ( 'NONE',  ( 6.943602653455000606, 1516.858069504249897, 216.0629462479770098 ) ) ;
#6953=CARTESIAN_POINT ( 'NONE',  ( -7.943222529415674416, 1511.827399570821171, 212.3015523490330452 ) ) ;
#6962=CARTESIAN_POINT ( 'NONE',  ( -3.461360131404999763, 1516.874084700499907, 205.8683838714370040 ) ) ;
#6964=CARTESIAN_POINT ( 'NONE',  ( 4.618583391875000110, 1516.939762005280045, 209.1087859301640322 ) ) ;
#6978=CARTESIAN_POINT ( 'NONE',  ( -6.549762485114999144, 1516.729202374750002, 213.7405950387170037 ) ) ;
#6982=CARTESIAN_POINT ( 'NONE',  ( 7.167019213315450443, 1508.551563895499839, 214.6350865034499691 ) ) ;
#6983=CARTESIAN_POINT ( 'NONE',  ( 1.718203463455000080, 1516.898441858519845, 210.8221056461869978 ) ) ;
#7002=CARTESIAN_POINT ( 'NONE',  ( -2.873958889724999910, 1516.588006113850042, 202.1873174023370154 ) ) ;
#7006=EDGE_CURVE ( 'NONE', #21616, #44160, #62344, .T. ) ;
#7027=CARTESIAN_POINT ( 'NONE',  ( -4.159863671365049420, 1508.728286123109910, 213.5483371690740171 ) ) ;
#7084=CARTESIAN_POINT ( 'NONE',  ( -1.701729858475000023, 1516.969638403840008, 212.0041719496170174 ) ) ;
#7087=CARTESIAN_POINT ( 'NONE',  ( -7.710285875814999912, 1516.582197289609894, 212.3822242253069987 ) ) ;
#7094=CARTESIAN_POINT ( 'NONE',  ( 2.290256263724999908, 1517.170721208160103, 202.1706708033170230 ) ) ;
#7104=ORIENTED_EDGE ( 'NONE', *, *, #62690, .F. ) ;
#7105=ORIENTED_EDGE ( 'NONE', *, *, #75513, .F. ) ;
#7112=CARTESIAN_POINT ( 'NONE',  ( -2.282622950494999969, 1516.861367446839949, 211.4218295478370067 ) ) ;
#7117=CARTESIAN_POINT ( 'NONE',  ( 1.700706776364999895, 1516.923170579120097, 206.8211163054370161 ) ) ;
#7119=DIRECTION ( 'NONE',  ( 0.000000000000000000, -1.000000000000000000, 6.123233995736769734E-17 ) ) ;
#7134=CARTESIAN_POINT ( 'NONE',  ( -6.937338783705000012, 1516.706638732659940, 213.7399656364970042 ) ) ;
#7137=CARTESIAN_POINT ( 'NONE',  ( 6.555393117025000826, 1516.809497469189864, 216.4498952504870033 ) ) ;
#7215=CARTESIAN_POINT ( 'NONE',  ( -7.726684725664999753, 1517.208444099459939, 207.9957078235169945 ) ) ;
#7227=CARTESIAN_POINT ( 'NONE',  ( 7.526515472008799890, 1517.051704408389924, 209.5611024095850041 ) ) ;
#7235=EDGE_LOOP ( 'NONE', ( #2156, #21366, #70373, #71162, #9440, #30933, #91937, #29011, #55062 ) ) ;
#7247=CARTESIAN_POINT ( 'NONE',  ( 7.710610402995000001, 1516.594591938570147, 205.6677260153969939 ) ) ;
#7309=B_SPLINE_CURVE_WITH_KNOTS ( 'NONE', 3,
 ( #58479, #17535, #243, #67998, #76373, #34371, #75826, #68545, #109977, #16431, #24833, #85872, #6953, #110522, #41110, #75287, #92606, #85303, #25389, #109433, #9173, #102644, #50623, #33254, #51736, #84756, #25944, #60140, #43338, #33804, #77486, #93695, #32159, #66346, #102110, #100462, #59582, #23745, #32710, #50082, #16975, #101000, #51174, #24296, #84211, #7507, #8053, #59038, #67445 ),
 .UNSPECIFIED., .F., .F.,
 ( 4, 2, 1, 2, 2, 2, 1, 1, 2, 2, 2, 2, 1, 1, 1, 2, 2, 2, 2, 1, 1, 1, 2, 2, 2, 1, 1, 2, 2, 4 ),
 ( 0.000000000000000000, 0.06249999999961332320, 0.09374999999955876961, 0.1093749999996599526, 0.1249999999997611078, 0.1875000000001662837, 0.2187500000003581302, 0.2343750000004542200, 0.2421875000005638823, 0.2500000000006735723, 0.3750000000012407853, 0.4375000000015574209, 0.4687500000017156832, 0.4843750000018106627, 0.4921875000018929858, 0.4960937500019232393, 0.5000000000019535484, 0.6250000000019894086, 0.6875000000019952928, 0.7187500000020067281, 0.7343750000020016211, 0.7421875000020143887, 0.7460937500020170532, 0.7500000000020197177, 0.8125000000015978330, 0.8437500000013867796, 0.8593750000012922996, 0.8671875000012422285, 0.8750000000011921575, 1.000000000000000000 ),
 .UNSPECIFIED. ) ;
#7339=CARTESIAN_POINT ( 'NONE',  ( -0.01327257453019850021, 1516.940252185109784, 206.2479269295770052 ) ) ;
#7349=CARTESIAN_POINT ( 'NONE',  ( -16.09179319795009633, 1514.742486295231856, 224.1276633295240117 ) ) ;
#7353=CARTESIAN_POINT ( 'NONE',  ( 4.044321679994999919, 1517.001127920769704, 211.4073335515969916 ) ) ;
#7381=CARTESIAN_POINT ( 'NONE',  ( -5.004442077115000664, 1516.690345681169902, 201.4087281291169802 ) ) ;
#7382=CARTESIAN_POINT ( 'NONE',  ( -2.297629659184999618, 1516.970035769810011, 208.3868227339359862 ) ) ;
#7386=CARTESIAN_POINT ( 'NONE',  ( 4.076676381798102433, 1511.455724275399234, 217.3418713267658973 ) ) ;
#7402=CARTESIAN_POINT ( 'NONE',  ( 0.7533001353030019942, 1516.714320817460020, 216.4479181143769893 ) ) ;
#7407=CARTESIAN_POINT ( 'NONE',  ( -1.704794841465000044, 1517.096587378560116, 213.7484378375869767 ) ) ;
#7410=CARTESIAN_POINT ( 'NONE',  ( 4.119379022663339995, 1508.879004046169939, 213.4915743296109838 ) ) ;
#7424=CARTESIAN_POINT ( 'NONE',  ( 0.7356989345870019736, 1517.020847257979995, 205.6609797614169963 ) ) ;
#7447=CARTESIAN_POINT ( 'NONE',  ( -13.59245260875518113, 1513.749539319655923, 192.3712733982298744 ) ) ;
#7471=CARTESIAN_POINT ( 'NONE',  ( 6.551643386774999023, 1516.807958722750072, 203.3403553877570005 ) ) ;
#7474=CARTESIAN_POINT ( 'NONE',  ( 16.85261132413500107, 1513.023086264660151, 195.9232021551670186 ) ) ;
#7506=CARTESIAN_POINT ( 'NONE',  ( 4.036119644515000715, 1516.647924054489977, 216.4458205765370167 ) ) ;
#7507=CARTESIAN_POINT ( 'NONE',  ( -8.520858377768730563, 1511.400001115551277, 214.1155622411217507 ) ) ;
#7513=EDGE_CURVE ( 'NONE', #11042, #20112, #71758, .T. ) ;
#7515=CARTESIAN_POINT ( 'NONE',  ( 2.477986732234999767, 1516.922519270759949, 205.8529865360470126 ) ) ;
#7522=CARTESIAN_POINT ( 'NONE',  ( 7.645478567275000081, 1514.134513140269974, 215.1770428866170164 ) ) ;
#7531=CARTESIAN_POINT ( 'NONE',  ( 0.7564342142240020328, 1516.783665406140017, 213.7345173100169973 ) ) ;
#7534=FACE_OUTER_BOUND ( 'NONE', #24165, .T. ) ;
#7535=CARTESIAN_POINT ( 'NONE',  ( 7.321627509198920691, 1508.611138448520023, 214.6350682835270050 ) ) ;
#7536=CARTESIAN_POINT ( 'NONE',  ( -2.476733514145000203, 1516.858326417339867, 211.6155457388669845 ) ) ;
#7550=CARTESIAN_POINT ( 'NONE',  ( 11.74136607283499956, 1511.863761374039996, 224.9732485802669828 ) ) ;
#7551=CARTESIAN_POINT ( 'NONE',  ( -2.485205687335000135, 1517.181921232829836, 216.8478361320569832 ) ) ;
#7555=VERTEX_POINT ( 'NONE', #50920 ) ;
#7556=CARTESIAN_POINT ( 'NONE',  ( 5.001338628314999646, 1516.911981270829983, 203.3378372969070256 ) ) ;
#7567=DIRECTION ( 'NONE',  ( -0.7063774289747313251, 0.04540766091858282338, 0.7063774289747313251 ) ) ;
#7593=CARTESIAN_POINT ( 'NONE',  ( 3.669386717837979983, 1517.051704638620095, 202.5807756278150009 ) ) ;
#7617=DIRECTION ( 'NONE',  ( 0.000000000000000000, -1.000000000000000000, 6.123233995736769734E-17 ) ) ;
#7627=CARTESIAN_POINT ( 'NONE',  ( 8.002723364794999128, 1516.551704408390151, 206.0688700356170102 ) ) ;
#7629=CARTESIAN_POINT ( 'NONE',  ( -2.477986770365000257, 1516.922519270759949, 212.3907053662870226 ) ) ;
#7631=CARTESIAN_POINT ( 'NONE',  ( 5.441672368615000366, 1511.126521646420088, 216.8250749888169935 ) ) ;
#7638=CARTESIAN_POINT ( 'NONE',  ( -5.781490582474999584, 1516.807958722750072, 202.5702025453269925 ) ) ;
#7639=ADVANCED_FACE ( 'NONE', ( #65132 ), #57934, .T. ) ;
#7654=CARTESIAN_POINT ( 'NONE',  ( -1.118104767724999782, 1516.965971551240045, 211.4215139361070044 ) ) ;
#7659=CARTESIAN_POINT ( 'NONE',  ( -7.339107240745000205, 1517.203017563489766, 207.9963360818169917 ) ) ;
#7676=CARTESIAN_POINT ( 'NONE',  ( 0.01289778877310149806, 1516.939723362869927, 214.1281058189269970 ) ) ;
#7679=CARTESIAN_POINT ( 'NONE',  ( -7.716252091104999877, 1516.810037859429940, 216.0641906620670056 ) ) ;
#7695=CARTESIAN_POINT ( 'NONE',  ( -14.77048072796499945, 1514.151220560310094, 224.0952811371670066 ) ) ;
#7756=CARTESIAN_POINT ( 'NONE',  ( -4.037051035714999792, 1516.939819969850078, 209.1350663277499962 ) ) ;
#7757=DIRECTION ( 'NONE',  ( -0.02616798426433289068, 0.9993150019884036173, 0.02616798426433289068 ) ) ;
#7764=CARTESIAN_POINT ( 'NONE',  ( -15.22870591643729909, 1512.406412987999829, 222.1534140603669698 ) ) ;
#7782=DIRECTION ( 'NONE',  ( -1.000000000000000000, 0.000000000000000000, 0.000000000000000000 ) ) ;
#7789=CARTESIAN_POINT ( 'NONE',  ( -0.7568987378019988999, 1516.805675336850072, 205.0906771642370074 ) ) ;
#7792=CARTESIAN_POINT ( 'NONE',  ( 14.77306016951930090, 1514.147575501539905, 194.1509863539160108 ) ) ;
#7815=CARTESIAN_POINT ( 'NONE',  ( 15.20279842864010078, 1514.921193439799936, 225.0317510863630162 ) ) ;
#7838=CARTESIAN_POINT ( 'NONE',  ( -7.710610441124999603, 1516.594591938570147, 212.5759658869370128 ) ) ;
#7842=ORIENTED_EDGE ( 'NONE', *, *, #22655, .T. ) ;
#7848=ORIENTED_EDGE ( 'NONE', *, *, #51201, .T. ) ;
#7880=CARTESIAN_POINT ( 'NONE',  ( -2.492443689034999910, 1516.793978928989873, 205.8699571027569846 ) ) ;
#7889=CARTESIAN_POINT ( 'NONE',  ( -16.68633777358233061, 1513.912053498707792, 222.9853921125541376 ) ) ;
#7893=CARTESIAN_POINT ( 'NONE',  ( 2.299983577604999940, 1516.861367446839949, 211.4044688825970013 ) ) ;
#7908=ORIENTED_EDGE ( 'NONE', *, *, #77071, .F. ) ;
#7919=CARTESIAN_POINT ( 'NONE',  ( -0.08509234499448949107, 1516.966051576868949, 216.6298010462417665 ) ) ;
#7925=CARTESIAN_POINT ( 'NONE',  ( -3.454119954834999895, 1516.594591938570147, 201.4112355291069889 ) ) ;
#7926=CARTESIAN_POINT ( 'NONE',  ( -4.623892098755000291, 1517.066898074209803, 208.3852847535989952 ) ) ;
#7951=CARTESIAN_POINT ( 'NONE',  ( -1.121950782074999875, 1517.123342927159911, 214.1352753262870010 ) ) ;
#7956=CARTESIAN_POINT ( 'NONE',  ( 4.333361510917200121, 1508.551704406479985, 213.7899733016769801 ) ) ;
#7957=ORIENTED_EDGE ( 'NONE', *, *, #100216, .F. ) ;
#7970=CARTESIAN_POINT ( 'NONE',  ( -2.492443689034999910, 1516.793978928989873, 205.8699571027569846 ) ) ;
#8018=CARTESIAN_POINT ( 'NONE',  ( -6.556651409415000131, 1516.858146885269889, 202.5689485651570010 ) ) ;
#8039=PLANE ( 'NONE',  #33939 ) ;
#8044=CARTESIAN_POINT ( 'NONE',  ( 6.017564063794999640, 1514.771170611759999, 201.2298835190769921 ) ) ;
#8052=CARTESIAN_POINT ( 'NONE',  ( 2.291047489114999891, 1516.524310051880093, 216.8306159772470210 ) ) ;
#8053=CARTESIAN_POINT ( 'NONE',  ( -8.566427451443020757, 1511.406470015435389, 214.2518601733771675 ) ) ;
#8059=CARTESIAN_POINT ( 'NONE',  ( -2.299014068865000038, 1516.811292230880099, 206.2578025137869986 ) ) ;
#8065=CARTESIAN_POINT ( 'NONE',  ( 7.943523441464999557, 1514.557408760809949, 215.5609834051570033 ) ) ;
#8073=CARTESIAN_POINT ( 'NONE',  ( 4.621897824414999967, 1516.858533673840157, 213.7337256555570093 ) ) ;
#8076=CARTESIAN_POINT ( 'NONE',  ( 5.984345938447710012, 1508.551704613440052, 216.1343701986449730 ) ) ;
#8077=CARTESIAN_POINT ( 'NONE',  ( -4.027051443935000030, 1516.733363207009916, 211.6130343286269806 ) ) ;
#8092=CARTESIAN_POINT ( 'NONE',  ( 2.485217193935000068, 1516.534320418310244, 216.8308781079170160 ) ) ;
#8097=CARTESIAN_POINT ( 'NONE',  ( -5.006329619514999330, 1516.755758396839838, 202.5714564999769891 ) ) ;
#8117=FACE_OUTER_BOUND ( 'NONE', #53866, .T. ) ;
#8172=CARTESIAN_POINT ( 'NONE',  ( 7.721907888235000073, 1517.026025493960105, 214.1263215447669950 ) ) ;
#8179=CARTESIAN_POINT ( 'NONE',  ( -1.130002532395000037, 1516.621991115350056, 202.1860446705670142 ) ) ;
#8193=CARTESIAN_POINT ( 'NONE',  ( -7.708745685915000756, 1516.523379810429788, 210.8299382363969983 ) ) ;
#8197=CARTESIAN_POINT ( 'NONE',  ( -1.133653179125000188, 1516.978425811520083, 208.3843950493249793 ) ) ;
#8214=CARTESIAN_POINT ( 'NONE',  ( -6.937965698444999774, 1516.732530461250008, 214.1275461716370216 ) ) ;
#8217=CARTESIAN_POINT ( 'NONE',  ( -4.034908597844999889, 1517.068717944079935, 216.4577469658269990 ) ) ;
#8219=CARTESIAN_POINT ( 'NONE',  ( 7.720548113794640344, 1516.974097803170025, 209.2608539945439929 ) ) ;
#8263=DIRECTION ( 'NONE',  ( 0.000000000000000000, -1.000000000000000000, 6.123233995736769734E-17 ) ) ;
#8282=DIRECTION ( 'NONE',  ( 0.000000000000000000, -1.000000000000000000, 6.123233995736769734E-17 ) ) ;
#8294=CARTESIAN_POINT ( 'NONE',  ( -7.663889450468710507, 1510.954290761809943, 214.5915452069070000 ) ) ;
#8299=EDGE_CURVE ( 'NONE', #100973, #100009, #29763, .T. ) ;
#8301=CARTESIAN_POINT ( 'NONE',  ( 0.7402208603880020554, 1516.992029636990083, 208.3685455796920110 ) ) ;
#8307=ORIENTED_EDGE ( 'NONE', *, *, #96093, .T. ) ;
#8310=CARTESIAN_POINT ( 'NONE',  ( -15.29008555799489955, 1513.004579589639889, 223.0186118662149966 ) ) ;
#8330=CARTESIAN_POINT ( 'NONE',  ( -4.492644309999670682, 1508.880967335730247, 205.3188433609270191 ) ) ;
#8332=CARTESIAN_POINT ( 'NONE',  ( 0.7355686427760019797, 1517.012231669750008, 205.8548062402470009 ) ) ;
#8383=CARTESIAN_POINT ( 'NONE',  ( -4.609996619675000851, 1516.769879638719885, 212.5810025483170023 ) ) ;
#8394=CARTESIAN_POINT ( 'NONE',  ( 15.84449002363500014, 1515.383078152259941, 223.0212718033670001 ) ) ;
#8425=CARTESIAN_POINT ( 'NONE',  ( -7.337793750624999944, 1517.145312756229941, 206.2496372219370073 ) ) ;
#8432=VERTEX_POINT ( 'NONE', #23716 ) ;
#8435=CARTESIAN_POINT ( 'NONE',  ( -16.43125158753896287, 1512.939392324912433, 220.7790245402972289 ) ) ;
#8439=CARTESIAN_POINT ( 'NONE',  ( -4.608021707265000266, 1516.660388280709867, 210.8351633799069873 ) ) ;
#8468=CARTESIAN_POINT ( 'NONE',  ( -6.944231786295000042, 1516.882690742909972, 202.5683215544970039 ) ) ;
#8469=CARTESIAN_POINT ( 'NONE',  ( 0.007128837152181529378, 1517.006509894990131, 209.8686634857439799 ) ) ;
#8488=ADVANCED_FACE ( 'NONE', ( #87512 ), #26474, .T. ) ;
#8491=CARTESIAN_POINT ( 'NONE',  ( 16.82650268237432201, 1517.015067831505576, 223.4080418569560322 ) ) ;
#8497=CARTESIAN_POINT ( 'NONE',  ( 4.491288139582719552, 1508.884219106000046, 212.6094330128009915 ) ) ;
#8513=CARTESIAN_POINT ( 'NONE',  ( 4.609064303374999838, 1516.723920667490120, 206.2441009858569885 ) ) ;
#8528=ORIENTED_EDGE ( 'NONE', *, *, #27617, .T. ) ;
#8533=CARTESIAN_POINT ( 'NONE',  ( 3.487592431261229642, 1509.038615938009798, 213.6090957240379851 ) ) ;
#8538=CARTESIAN_POINT ( 'NONE',  ( -14.32480461217465262, 1514.214463197139139, 192.6030336675313777 ) ) ;
#8539=LINE ( 'NONE', #78525, #109372 ) ;
#8556=CARTESIAN_POINT ( 'NONE',  ( -5.513222351421919853, 1508.611138448520023, 216.4434734794269843 ) ) ;
#8565=CARTESIAN_POINT ( 'NONE',  ( -3.456007423304999993, 1516.647534046129977, 202.5739645571870255 ) ) ;
#8566=VECTOR ( 'NONE', #97905, 1000.000000000000114 ) ;
#8584=EDGE_CURVE ( 'NONE', #11042, #10258, #20278, .T. ) ;
#8592=CARTESIAN_POINT ( 'NONE',  ( 7.211759810944999849, 1511.702066573629963, 202.3497083402869805 ) ) ;
#8599=AXIS2_PLACEMENT_3D ( 'NONE', #38062, #20144, #106367 ) ;
#8600=CARTESIAN_POINT ( 'NONE',  ( -2.290886304614999869, 1517.184383877180153, 216.4605998004670084 ) ) ;
#8605=CARTESIAN_POINT ( 'NONE',  ( 1.701027822874999984, 1516.937508036699910, 206.6270879340970055 ) ) ;
#8610=CARTESIAN_POINT ( 'NONE',  ( 7.458171671575000161, 1513.513616978040091, 215.6792808263570009 ) ) ;
#8620=CARTESIAN_POINT ( 'NONE',  ( -6.550389470255000290, 1516.755758396839838, 214.1281755516169767 ) ) ;
#8625=CARTESIAN_POINT ( 'NONE',  ( 6.769623004886519801, 1509.032014039220030, 216.3879256010220047 ) ) ;
#8626=CARTESIAN_POINT ( 'NONE',  ( -5.770883602015000058, 1516.603620185149794, 211.4160555996369908 ) ) ;
#8638=CARTESIAN_POINT ( 'NONE',  ( 10.96771871713499813, 1512.594959757389915, 225.0393121556670053 ) ) ;
#8645=CARTESIAN_POINT ( 'NONE',  ( 3.257220602695000355, 1517.040132827679827, 203.3350082531769942 ) ) ;
#8667=PLANE ( 'NONE',  #94587 ) ;
#8680=EDGE_CURVE ( 'NONE', #17382, #54193, #56412, .T. ) ;
#8703=AXIS2_PLACEMENT_3D ( 'NONE', #5623, #31913, #90714 ) ;
#8704=CARTESIAN_POINT ( 'NONE',  ( 7.540337753453409064, 1510.559702729411583, 203.3485307114503655 ) ) ;
#8720=ORIENTED_EDGE ( 'NONE', *, *, #81624, .F. ) ;
#8725=CARTESIAN_POINT ( 'NONE',  ( -3.449149233875000053, 1516.947419719950176, 213.7456339395970133 ) ) ;
#8731=CARTESIAN_POINT ( 'NONE',  ( -5.008848238024999233, 1516.858456333729919, 204.1217621043670079 ) ) ;
#8743=CARTESIAN_POINT ( 'NONE',  ( -4.802229637768189896, 1508.551704408389924, 204.6920723467030143 ) ) ;
#8744=CARTESIAN_POINT ( 'NONE',  ( -5.771149113014999443, 1516.616791731099966, 211.6102065995370083 ) ) ;
#8749=CARTESIAN_POINT ( 'NONE',  ( 6.944466742375000834, 1516.939530130779985, 209.1105810159089913 ) ) ;
#8750=VERTEX_POINT ( 'NONE', #32552 ) ;
#8766=CARTESIAN_POINT ( 'NONE',  ( 4.620008207075000151, 1516.777260590120022, 214.8964555921769772 ) ) ;
#8769=CARTESIAN_POINT ( 'NONE',  ( -5.003848160104999998, 1517.005755693489846, 216.4561742428970206 ) ) ;
#8843=CARTESIAN_POINT ( 'NONE',  ( -8.248023465271721477, 1511.495156305270029, 214.8261723429600067 ) ) ;
#8849=ORIENTED_EDGE ( 'NONE', *, *, #2404, .F. ) ;
#8850=CARTESIAN_POINT ( 'NONE',  ( -2.297629659184999618, 1516.970035769810011, 208.3868227339359862 ) ) ;
#8859=CARTESIAN_POINT ( 'NONE',  ( -14.90569725764700060, 1513.941944659479987, 223.9356467521019738 ) ) ;
#8860=CARTESIAN_POINT ( 'NONE',  ( 4.616899834755000320, 1517.050041317280147, 201.3993091674070115 ) ) ;
#8883=CARTESIAN_POINT ( 'NONE',  ( 1.702754371344999962, 1517.014196759610059, 205.6580786742169948 ) ) ;
#8886=CARTESIAN_POINT ( 'NONE',  ( 15.21196346850829961, 1512.378201925219855, 196.1437262287770125 ) ) ;
#8890=VECTOR ( 'NONE', #109631, 1000.000000000000000 ) ;
#8940=CARTESIAN_POINT ( 'NONE',  ( -2.285487619494999567, 1517.001127920769704, 213.1661676502270097 ) ) ;
#8979=CARTESIAN_POINT ( 'NONE',  ( 15.90990255763500016, 1512.830284628050094, 198.1616908427670296 ) ) ;
#8987=CARTESIAN_POINT ( 'NONE',  ( 0.7355686427760019797, 1517.012231669750008, 205.8548062402470009 ) ) ;
#8996=CARTESIAN_POINT ( 'NONE',  ( -16.78772373697407971, 1513.520094851864087, 222.2831617812080935 ) ) ;
#9000=CARTESIAN_POINT ( 'NONE',  ( -3.445407572115000150, 1516.764084769670262, 211.4198948937369948 ) ) ;
#9024=CARTESIAN_POINT ( 'NONE',  ( -4.487249791936469556, 1509.038615938009798, 212.6094384014929801 ) ) ;
#9025=FACE_OUTER_BOUND ( 'NONE', #69526, .T. ) ;
#9031=CARTESIAN_POINT ( 'NONE',  ( 0.7376675027960020170, 1517.104497701820037, 203.3349981924270082 ) ) ;
#9032=CARTESIAN_POINT ( 'NONE',  ( -0.7468175536419978666, 1517.006509894990131, 209.1289748073840258 ) ) ;
#9036=CARTESIAN_POINT ( 'NONE',  ( 3.029820084536003488, 1511.989325512496180, 217.0244469535358576 ) ) ;
#9052=AXIS2_PLACEMENT_3D ( 'NONE', #105947, #29226, #97530 ) ;
#9074=CARTESIAN_POINT ( 'NONE',  ( -14.97406874466500071, 1513.863307887919973, 223.8916988856670116 ) ) ;
#9080=CARTESIAN_POINT ( 'NONE',  ( 4.608417506514999928, 1516.691389976299888, 206.6316000176769876 ) ) ;
#9097=CARTESIAN_POINT ( 'NONE',  ( -2.412416396784999861, 1511.982868782460173, 201.5319981951469970 ) ) ;
#9103=CARTESIAN_POINT ( 'NONE',  ( -14.78589604906941624, 1514.559375976630236, 192.8644648269931281 ) ) ;
#9134=CIRCLE ( 'NONE', #25248, 1.000000000039237946 ) ;
#9135=CARTESIAN_POINT ( 'NONE',  ( -0.7553264739829980146, 1516.745833913490060, 203.3462208547369983 ) ) ;
#9137=CARTESIAN_POINT ( 'NONE',  ( 15.36767543323500007, 1514.414736986979960, 193.7450394534670295 ) ) ;
#9154=VECTOR ( 'NONE', #86328, 1000.000000000000114 ) ;
#9160=CARTESIAN_POINT ( 'NONE',  ( -4.608146819384999482, 1516.677239312369920, 211.4179708211670174 ) ) ;
#9163=CARTESIAN_POINT ( 'NONE',  ( 6.166911752485000342, 1513.656171171930055, 201.5360455003170159 ) ) ;
#9172=CARTESIAN_POINT ( 'NONE',  ( -4.034908597844999889, 1517.068717944079935, 216.4577469658269990 ) ) ;
#9173=CARTESIAN_POINT ( 'NONE',  ( -8.100270648889271285, 1511.553914495710615, 212.8212201628993228 ) ) ;
#9181=CARTESIAN_POINT ( 'NONE',  ( -4.043366258305000294, 1516.951766529250108, 206.2549880390970145 ) ) ;
#9188=CARTESIAN_POINT ( 'NONE',  ( 7.181020144905000180, 1512.881909847370025, 216.0859015499169971 ) ) ;
#9199=CARTESIAN_POINT ( 'NONE',  ( -4.032397940005000514, 1516.981965530290154, 214.9074288837770155 ) ) ;
#9203=CARTESIAN_POINT ( 'NONE',  ( -7.722171335595510833, 1517.036116044630262, 208.7506064649060136 ) ) ;
#9204=CARTESIAN_POINT ( 'NONE',  ( 5.788436334164999586, 1517.116049120239950, 211.4102033778369787 ) ) ;
#9217=CIRCLE ( 'NONE', #98637, 7.500000000000000000 ) ;
#9223=CARTESIAN_POINT ( 'NONE',  ( 0.7376675027960020170, 1517.104497701820037, 203.3349981924270082 ) ) ;
#9242=CARTESIAN_POINT ( 'NONE',  ( -4.369728397509249795, 1508.879004046169939, 213.2412249928949848 ) ) ;
#9282=LINE ( 'NONE', #43994, #26918 ) ;
#9296=CARTESIAN_POINT ( 'NONE',  ( 4.040527303974999818, 1516.815231249920089, 213.7327841816070020 ) ) ;
#9301=CARTESIAN_POINT ( 'NONE',  ( -7.333070173014999860, 1516.955859323880077, 203.3428461583270064 ) ) ;
#9306=CARTESIAN_POINT ( 'NONE',  ( 7.861206899714999530, 1512.631076693560090, 221.9328003382670147 ) ) ;
#9311=CARTESIAN_POINT ( 'NONE',  ( 8.002723364794999128, 1516.551704408390151, 206.0688700356170102 ) ) ;
#9318=CARTESIAN_POINT ( 'NONE',  ( -7.322105105754999954, 1516.572193931679976, 211.9951753309869957 ) ) ;
#9324=CARTESIAN_POINT ( 'NONE',  ( -5.013429394184999666, 1517.123342927159911, 207.9998951881570122 ) ) ;
#9338=CARTESIAN_POINT ( 'NONE',  ( 0.4346943641293429805, 1517.051704428850144, 201.3992661435559910 ) ) ;
#9340=CARTESIAN_POINT ( 'NONE',  ( 1.713317409674999903, 1516.660388280709867, 213.7298676393670291 ) ) ;
#9343=CARTESIAN_POINT ( 'NONE',  ( 0.7526715501680020237, 1516.710624944440042, 216.8354948044169817 ) ) ;
#9345=CARTESIAN_POINT ( 'NONE',  ( -1.128757599205000073, 1516.608208975040043, 201.4108789544669946 ) ) ;
#9376=CARTESIAN_POINT ( 'NONE',  ( -2.725458657727350076, 1516.549587951120202, 201.4124141148399758 ) ) ;
#9383=VERTEX_POINT ( 'NONE', #25650 ) ;
#9420=CARTESIAN_POINT ( 'NONE',  ( -2.480427292634999947, 1516.872851364150165, 209.8797317620669673 ) ) ;
#9435=CARTESIAN_POINT ( 'NONE',  ( -2.491655763544999846, 1516.977504706749869, 208.3867361609839861 ) ) ;
#9440=ORIENTED_EDGE ( 'NONE', *, *, #54124, .F. ) ;
#9451=CARTESIAN_POINT ( 'NONE',  ( -3.267291643295000103, 1516.842852731759876, 205.6749038603869906 ) ) ;
#9452=ORIENTED_EDGE ( 'NONE', *, *, #17385, .F. ) ;
#9454=CARTESIAN_POINT ( 'NONE',  ( -6.541070373676360461, 1517.051704644259871, 205.4524592699869743 ) ) ;
#9460=CARTESIAN_POINT ( 'NONE',  ( -15.01814846036320006, 1514.214451730469818, 194.3960741685959874 ) ) ;
#9495=CARTESIAN_POINT ( 'NONE',  ( 4.622842844184999578, 1516.901952101700090, 213.1523604828169880 ) ) ;
#9507=ORIENTED_EDGE ( 'NONE', *, *, #110602, .F. ) ;
#9532=CARTESIAN_POINT ( 'NONE',  ( -6.951883559441813354, 1516.584123404785487, 211.9369655874735940 ) ) ;
#9535=CARTESIAN_POINT ( 'NONE',  ( -13.29425504400375857, 1516.551188142741921, 225.9939214950833559 ) ) ;
#9536=CARTESIAN_POINT ( 'NONE',  ( -0.7578858299649979813, 1516.872851364150165, 206.6414186775969881 ) ) ;
#9548=CARTESIAN_POINT ( 'NONE',  ( 4.624099291334999862, 1516.962555622980062, 212.3771868965270073 ) ) ;
#9570=CARTESIAN_POINT ( 'NONE',  ( 6.081399314780780330, 1508.610505977490220, 201.8017946903299844 ) ) ;
#9575=CARTESIAN_POINT ( 'NONE',  ( 1.124289655455000148, 1517.184063036290127, 202.5579304082170040 ) ) ;
#9576=CARTESIAN_POINT ( 'NONE',  ( -2.480427292634999947, 1516.872851364150165, 209.8797317620669673 ) ) ;
#9579=CARTESIAN_POINT ( 'NONE',  ( 4.597999444932870716, 1511.399594748111213, 217.5114347307018363 ) ) ;
#9614=CARTESIAN_POINT ( 'NONE',  ( -15.82925655696500122, 1512.053076656670100, 221.8543121690670148 ) ) ;
#9619=CARTESIAN_POINT ( 'NONE',  ( -2.493699806765000027, 1516.858326417339867, 206.6451124560869914 ) ) ;
#9647=CARTESIAN_POINT ( 'NONE',  ( -14.45097772706500017, 1514.857962383129916, 193.8743388492669908 ) ) ;
#9648=ADVANCED_FACE ( 'NONE', ( #53664 ), #46916, .T. ) ;
#9673=CARTESIAN_POINT ( 'NONE',  ( -6.557909920764999789, 1516.908489800550115, 203.3441005368270282 ) ) ;
#9688=CARTESIAN_POINT ( 'NONE',  ( -3.487592468881668406, 1508.603735221695615, 213.8522301334431290 ) ) ;
#9698=CARTESIAN_POINT ( 'NONE',  ( 2.880592928985000079, 1516.859514182039902, 211.9868180862470126 ) ) ;
#9702=CARTESIAN_POINT ( 'NONE',  ( 6.382129819174999774, 1514.500328598809801, 201.2525669677770281 ) ) ;
#9709=CARTESIAN_POINT ( 'NONE',  ( -7.380526870715000243, 1511.503799556579906, 215.6010310885870069 ) ) ;
#9710=CARTESIAN_POINT ( 'NONE',  ( 16.60142420124314455, 1513.050501378471836, 197.0834984225024016 ) ) ;
#9711=LINE ( 'NONE', #60138, #52833 ) ;
#9712=CARTESIAN_POINT ( 'NONE',  ( 5.004442038985000174, 1516.690345681169902, 216.8349637732169697 ) ) ;
#9720=CARTESIAN_POINT ( 'NONE',  ( -2.880592967115000125, 1516.859514182039902, 206.2568738160869941 ) ) ;
#9726=CARTESIAN_POINT ( 'NONE',  ( -6.648420388365120282, 1508.610128767860033, 202.0257353737460164 ) ) ;
#9731=CARTESIAN_POINT ( 'NONE',  ( -6.067071732141870122, 1511.169205552290123, 201.5628721129530163 ) ) ;
#9738=CARTESIAN_POINT ( 'NONE',  ( -5.776491133374999976, 1516.858301627840092, 214.9045953718370185 ) ) ;
#9742=CARTESIAN_POINT ( 'NONE',  ( -3.251888867474999945, 1516.793978928989873, 211.6142896211370044 ) ) ;
#9750=CARTESIAN_POINT ( 'NONE',  ( -7.549016801754999229, 1510.423579818969984, 213.5498276941069946 ) ) ;
#9760=CARTESIAN_POINT ( 'NONE',  ( -2.294209667535000108, 1516.603620185149794, 203.3509623682169831 ) ) ;
#9788=CARTESIAN_POINT ( 'NONE',  ( -6.126746181595000174, 1514.923664147150021, 217.2480802176870043 ) ) ;
#9843=CARTESIAN_POINT ( 'NONE',  ( 5.784638319815000429, 1516.939574742129935, 213.7356083271170064 ) ) ;
#9844=CARTESIAN_POINT ( 'NONE',  ( 4.542415389984999941, 1511.388520542559945, 217.4923749357569989 ) ) ;
#9848=CARTESIAN_POINT ( 'NONE',  ( -1.131796848745000084, 1516.659138130710289, 203.3488676535569937 ) ) ;
#9862=CARTESIAN_POINT ( 'NONE',  ( 3.268235720634999897, 1516.890356958860139, 211.9874346545169885 ) ) ;
#9868=CARTESIAN_POINT ( 'NONE',  ( 0.7374508827770021036, 1516.978425811520083, 207.9881927911069965 ) ) ;
#9875=CARTESIAN_POINT ( 'NONE',  ( 7.012921545474999796, 1509.051704408389924, 209.1218459511669892 ) ) ;
#9880=CARTESIAN_POINT ( 'NONE',  ( 4.429742651635811157, 1508.551704408389924, 213.9240872047329844 ) ) ;
#9883=CARTESIAN_POINT ( 'NONE',  ( -5.776491133374999976, 1516.858301627840092, 214.9045953718370185 ) ) ;
#9901=LINE ( 'NONE', #22957, #48489 ) ;
#9906=CARTESIAN_POINT ( 'NONE',  ( 6.742044244646490547, 1509.032357808383040, 202.0097227829280655 ) ) ;
#9949=ORIENTED_EDGE ( 'NONE', *, *, #91847, .F. ) ;
#9969=CARTESIAN_POINT ( 'NONE',  ( -2.286472924554999953, 1516.883361325900069, 209.8798303522490016 ) ) ;
#9978=CARTESIAN_POINT ( 'NONE',  ( -14.77306020744990001, 1514.147575501819802, 224.0927055486180279 ) ) ;
#9980=CARTESIAN_POINT ( 'NONE',  ( 7.329930013194999816, 1516.881930554049859, 201.4037113026670056 ) ) ;
#9986=CARTESIAN_POINT ( 'NONE',  ( 5.772978278544999675, 1516.659138130710289, 207.9900491214870044 ) ) ;
#10002=CARTESIAN_POINT ( 'NONE',  ( -0.7572979743539989261, 1516.829948096479939, 205.6721984920870057 ) ) ;
#10022=CARTESIAN_POINT ( 'NONE',  ( -3.449149233875000053, 1516.947419719950176, 213.7456339395970133 ) ) ;
#10042=CARTESIAN_POINT ( 'NONE',  ( -6.520294809802511971, 1509.032998946479893, 201.8615409552149913 ) ) ;
#10049=CARTESIAN_POINT ( 'NONE',  ( 4.040527303974999818, 1516.815231249920089, 213.7327841816070020 ) ) ;
#10088=CARTESIAN_POINT ( 'NONE',  ( -7.075104946580074383, 1516.558315471130072, 211.6107311714952175 ) ) ;
#10093=CARTESIAN_POINT ( 'NONE',  ( -2.493699806765000027, 1516.858326417339867, 206.6451124560869914 ) ) ;
#10107=CARTESIAN_POINT ( 'NONE',  ( -1.701729858475000023, 1516.969638403840008, 212.0041719496170174 ) ) ;
#10126=EDGE_LOOP ( 'NONE', ( #95739, #97752, #42264, #66882, #51027, #20805, #34361 ) ) ;
#10136=CARTESIAN_POINT ( 'NONE',  ( -6.943602691585000208, 1516.858069504249897, 202.1807456543569685 ) ) ;
#10137=CARTESIAN_POINT ( 'NONE',  ( -3.460866208815000178, 1517.020847257979995, 208.3861469975149987 ) ) ;
#10175=CARTESIAN_POINT ( 'NONE',  ( -15.24995208726499918, 1513.868118914750085, 224.0843299309669874 ) ) ;
#10179=CARTESIAN_POINT ( 'NONE',  ( 2.282915183265000092, 1516.876240617270014, 206.6278256496669883 ) ) ;
#10197=CARTESIAN_POINT ( 'NONE',  ( -2.966690011115000303, 1511.639769324940062, 201.4286129170669710 ) ) ;
#10220=CARTESIAN_POINT ( 'NONE',  ( -7.167019251197560337, 1508.551563895499839, 214.6350865074379897 ) ) ;
#10230=CARTESIAN_POINT ( 'NONE',  ( 2.480187016714999970, 1517.025470194390209, 204.4964864072570094 ) ) ;
#10242=ORIENTED_EDGE ( 'NONE', *, *, #91847, .T. ) ;
#10251=CARTESIAN_POINT ( 'NONE',  ( 1.135460316954999938, 1516.790374942449944, 212.3751473514870156 ) ) ;
#10254=CARTESIAN_POINT ( 'NONE',  ( 6.910053031764999965, 1514.330398624150121, 201.0829441462669820 ) ) ;
#10258=VERTEX_POINT ( 'NONE', #65639 ) ;
#10260=CARTESIAN_POINT ( 'NONE',  ( -8.207084992775001808, 1512.038636172079805, 215.4514803347070142 ) ) ;
#10271=CARTESIAN_POINT ( 'NONE',  ( -3.461995196814999787, 1516.906233342200039, 206.2559344154570056 ) ) ;
#10287=CARTESIAN_POINT ( 'NONE',  ( -0.7376675409259989546, 1517.104497701820037, 214.9086937099069985 ) ) ;
#10289=CARTESIAN_POINT ( 'NONE',  ( 6.067071694012949656, 1511.169205552290123, 216.6808197893799957 ) ) ;
#10292=CARTESIAN_POINT ( 'NONE',  ( 7.337793712495000342, 1517.145312756229941, 211.9940546803969994 ) ) ;
#10312=CARTESIAN_POINT ( 'NONE',  ( -0.7553264739829980146, 1516.745833913490060, 203.3462208547369983 ) ) ;
#10322=CARTESIAN_POINT ( 'NONE',  ( -7.709487050242899819, 1516.551695078709827, 211.8815864275139802 ) ) ;
#10360=CARTESIAN_POINT ( 'NONE',  ( -5.399591253687431092, 1511.369014876797792, 201.1386261298281397 ) ) ;
#10369=CARTESIAN_POINT ( 'NONE',  ( -7.656028705865000283, 1510.967342883699985, 213.6171158279370275 ) ) ;
#10374=SHAPE_REPRESENTATION_RELATIONSHIP ( 'NONE' , 'NONE' ,  #60858, #51910 ) ;
#10391=CARTESIAN_POINT ( 'NONE',  ( -4.611879723454999969, 1516.858533673840157, 213.7437437946470027 ) ) ;
#10392=CARTESIAN_POINT ( 'NONE',  ( 2.541812758945000361, 1512.177707669779920, 216.7470359957769972 ) ) ;
#10399=CARTESIAN_POINT ( 'NONE',  ( -0.7553264739829980146, 1516.745833913490060, 203.3462208547369983 ) ) ;
#10405=B_SPLINE_SURFACE_WITH_KNOTS ( 'NONE', 5, 5, ( 
 ( #93733, #17012, #16470, #104236, #10738, #109471, #67482, #8638, #44911 ),
 ( #44345, #101586, #79058, #36476, #7550, #24872, #70673, #78488, #1802 ),
 ( #61709, #57971, #92106, #41704, #32749, #4537, #71218, #81767, #88546 ),
 ( #64459, #105342, #46554, #29181, #47095, #89080, #12915, #47639, #19667 ),
 ( #81222, #72846, #80133, #98022, #12368, #72307, #80689, #96949, #63907 ),
 ( #3452, #29722, #46001, #13449, #56040, #20215, #37580, #21843, #4000 ),
 ( #54414, #38671, #55501, #30268, #28631, #98575, #106980, #62836, #5070 ),
 ( #53872, #90167, #11831, #38126, #63372, #39219, #106438, #104788, #28074 ),
 ( #105902, #62262, #96391, #71783, #21294, #89627, #88011, #11293, #97487 ) ),
 .UNSPECIFIED., .F., .F., .F.,
 ( 6, 3, 6 ),
 ( 6, 3, 6 ),
 ( 9.902195898209999569, 12.38020728900000123, 16.40090783169999966 ),
 ( 0.000000000000000000, 0.5000000000000000000, 1.000000000000000000 ),
 .UNSPECIFIED. ) ;
#10406=CARTESIAN_POINT ( 'NONE',  ( 1.126138108584999964, 1517.208444099459939, 201.3951612445669923 ) ) ;
#10416=CARTESIAN_POINT ( 'NONE',  ( -3.252530653725000054, 1516.827328999679821, 212.0018028951869837 ) ) ;
#10422=CARTESIAN_POINT ( 'NONE',  ( 3.261652286895000419, 1516.939580991450157, 209.1085619926769823 ) ) ;
#10438=CARTESIAN_POINT ( 'NONE',  ( -0.7386049428049979992, 1517.122674412569950, 215.6839400395269877 ) ) ;
#10443=CARTESIAN_POINT ( 'NONE',  ( 6.942354273414999888, 1516.905946377369901, 201.4030824261969883 ) ) ;
#10449=CARTESIAN_POINT ( 'NONE',  ( 7.580297983975060383, 1511.034527886640262, 203.1778469106609748 ) ) ;
#10481=CARTESIAN_POINT ( 'NONE',  ( -2.204892687444989896, 1516.527839230000154, 201.4129835103060202 ) ) ;
#10488=EDGE_LOOP ( 'NONE', ( #19052, #32248, #15479, #68975 ) ) ;
#10515=CARTESIAN_POINT ( 'NONE',  ( -6.942344730043687129, 1516.810037862407626, 201.4055939276168488 ) ) ;
#10524=CARTESIAN_POINT ( 'NONE',  ( 7.724874613184999461, 1517.139320148880188, 209.8621665372610039 ) ) ;
#10542=CARTESIAN_POINT ( 'NONE',  ( 2.477975315464999717, 1516.839862955080207, 207.9852983471170091 ) ) ;
#10547=VERTEX_POINT ( 'NONE', #98396 ) ;
#10561=CARTESIAN_POINT ( 'NONE',  ( 5.772403774305000290, 1516.676340709600026, 205.8583240277470168 ) ) ;
#10583=CARTESIAN_POINT ( 'NONE',  ( 6.559168636745000391, 1516.960844870249957, 214.1244393295569921 ) ) ;
#10599=ORIENTED_EDGE ( 'NONE', *, *, #990, .F. ) ;
#10640=VECTOR ( 'NONE', #64870, 1000.000000000000114 ) ;
#10654=CARTESIAN_POINT ( 'NONE',  ( -6.064575543111884848, 1516.744957452581048, 213.5348771919006197 ) ) ;
#10658=CARTESIAN_POINT ( 'NONE',  ( -13.49160170200362963, 1516.729020965288555, 226.1741075741266229 ) ) ;
#10659=CARTESIAN_POINT ( 'NONE',  ( -4.044321718124999521, 1517.001127920769704, 206.8363583507369867 ) ) ;
#10667=CYLINDRICAL_SURFACE ( 'NONE', #83170, 2.999999999999995115 ) ;
#10668=EDGE_LOOP ( 'NONE', ( #12851, #34431, #25475, #92898 ) ) ;
#10673=CARTESIAN_POINT ( 'NONE',  ( 1.715704490974999885, 1516.757508073510053, 212.3732403323669757 ) ) ;
#10680=DIRECTION ( 'NONE',  ( 0.06162841671618445039, -0.9961946980917499861, 0.06162841671618458916 ) ) ;
#10699=CARTESIAN_POINT ( 'NONE',  ( -0.01171164408179850049, 1516.939568781210028, 202.5649949355269825 ) ) ;
#10700=CARTESIAN_POINT ( 'NONE',  ( 7.727327114725000001, 1517.232977404109988, 210.8318586907270173 ) ) ;
#10723=CARTESIAN_POINT ( 'NONE',  ( -7.458171709695000651, 1513.513616978009850, 202.5644110759569969 ) ) ;
#10733=EDGE_LOOP ( 'NONE', ( #10242, #27059, #45551 ) ) ;
#10738=CARTESIAN_POINT ( 'NONE',  ( 11.40944910053500116, 1511.843510977570077, 224.6458867293669925 ) ) ;
#10746=AXIS2_PLACEMENT_3D ( 'NONE', #21610, #64774, #91594 ) ;
#10747=CARTESIAN_POINT ( 'NONE',  ( -3.268859434184999913, 1516.922519270759949, 206.6438591998669949 ) ) ;
#10765=CARTESIAN_POINT ( 'NONE',  ( -3.276907064705000039, 1511.440441732949921, 201.4048293130770162 ) ) ;
#10799=CARTESIAN_POINT ( 'NONE',  ( -4.040527342105000308, 1516.815231249920089, 204.5109077207270047 ) ) ;
#10820=CARTESIAN_POINT ( 'NONE',  ( -6.934528567894999718, 1516.588006113850042, 211.9958048218269937 ) ) ;
#10830=CARTESIAN_POINT ( 'NONE',  ( -7.475494293344999264, 1511.623805160490065, 215.5182564808370103 ) ) ;
#10831=CARTESIAN_POINT ( 'NONE',  ( 16.72494116235394301, 1513.190421814297224, 196.6872607197416585 ) ) ;
#10842=CARTESIAN_POINT ( 'NONE',  ( -3.462948834675000143, 1516.956048353049937, 206.8373194734570006 ) ) ;
#10848=CARTESIAN_POINT ( 'NONE',  ( -6.551934178310329315, 1508.551568321310015, 202.1599716710999814 ) ) ;
#10859=CARTESIAN_POINT ( 'NONE',  ( 1.569161254424999985, 1517.051704408389924, 201.3992656178269840 ) ) ;
#10860=CARTESIAN_POINT ( 'NONE',  ( 2.294209629405000062, 1516.603620185149794, 214.8927295341169952 ) ) ;
#10862=CARTESIAN_POINT ( 'NONE',  ( 5.835879592667029492, 1511.569910118449798, 217.3960280942959855 ) ) ;
#10865=CARTESIAN_POINT ( 'NONE',  ( -6.934528567894999718, 1516.588006113850042, 211.9958048218269937 ) ) ;
#10883=CARTESIAN_POINT ( 'NONE',  ( -0.01244697378919850002, 1516.939646076049939, 203.3402601539570185 ) ) ;
#10904=CARTESIAN_POINT ( 'NONE',  ( -4.414895773965000103, 1511.801704408389924, 205.7066075212470082 ) ) ;
#10908=DIRECTION ( 'NONE',  ( -0.7063774289747313251, 0.04540766091858282338, 0.7063774289747313251 ) ) ;
#10921=CARTESIAN_POINT ( 'NONE',  ( -1.906499846882070084E-08, 1516.051704408390151, 209.1218459511669892 ) ) ;
#10923=CARTESIAN_POINT ( 'NONE',  ( -6.942344729965000738, 1516.810037859429940, 201.4055938791270250 ) ) ;
#10932=ORIENTED_EDGE ( 'NONE', *, *, #79903, .F. ) ;
#10957=CARTESIAN_POINT ( 'NONE',  ( -1.123101616545000070, 1517.157901477309906, 214.9105372957470195 ) ) ;
#10958=CARTESIAN_POINT ( 'NONE',  ( 2.822464090084999988, 1512.205735116489905, 216.8958673752769926 ) ) ;
#10959=STYLED_ITEM ( 'NONE', ( #20967 ), #51910 ) ;
#10964=CARTESIAN_POINT ( 'NONE',  ( 4.610938211375000151, 1516.815231249920089, 205.0813186281270077 ) ) ;
#10967=CARTESIAN_POINT ( 'NONE',  ( 6.942354273414999888, 1516.905946377369901, 201.4030824261969883 ) ) ;
#10977=CARTESIAN_POINT ( 'NONE',  ( -1.701729858475000023, 1516.969638403840008, 212.0041719496170174 ) ) ;
#10982=CARTESIAN_POINT ( 'NONE',  ( -4.037051035714999792, 1516.939819969850078, 209.1350663277499962 ) ) ;
#10996=CARTESIAN_POINT ( 'NONE',  ( 4.802229599638190294, 1508.551704408389924, 213.5516195556409969 ) ) ;
#10998=CARTESIAN_POINT ( 'NONE',  ( -2.870951705914999597, 1517.111322026010157, 215.6844817927369888 ) ) ;
#11009=CARTESIAN_POINT ( 'NONE',  ( 7.679927584005029395, 1511.009256124219974, 203.5019279399089953 ) ) ;
#11025=EDGE_CURVE ( 'NONE', #78418, #48402, #79305, .T. ) ;
#11040=CARTESIAN_POINT ( 'NONE',  ( -2.265367662664029780, 1516.528448466100144, 201.4129675568979962 ) ) ;
#11042=VERTEX_POINT ( 'NONE', #9311 ) ;
#11068=ADVANCED_FACE ( 'NONE', ( #31062 ), #15880, .F. ) ;
#11085=MANIFOLD_SOLID_BREP ( 'Stock-MAS-682-1', #43092 ) ;
#11091=CARTESIAN_POINT ( 'NONE',  ( 0.7533003524100010395, 1516.992029636990083, 209.8620668306199946 ) ) ;
#11100=CYLINDRICAL_SURFACE ( 'NONE', #96162, 1.000000000000003775 ) ;
#11107=EDGE_CURVE ( 'NONE', #37652, #51148, #80323, .T. ) ;
#11111=CARTESIAN_POINT ( 'NONE',  ( 2.284053471355000031, 1516.854133554269993, 207.9850318982369970 ) ) ;
#11128=CARTESIAN_POINT ( 'NONE',  ( -7.338411997524999286, 1517.170512887980067, 206.6372682748769876 ) ) ;
#11145=CARTESIAN_POINT ( 'NONE',  ( -2.289624470354999719, 1517.154223579619838, 215.6854418399169901 ) ) ;
#11152=CARTESIAN_POINT ( 'NONE',  ( 4.277761459085749784, 1517.051704409989952, 201.7957048000489806 ) ) ;
#11192=EDGE_CURVE ( 'NONE', #46100, #107968, #15043, .T. ) ;
#11208=EDGE_CURVE ( 'NONE', #93671, #66885, #57056, .T. ) ;
#11219=CARTESIAN_POINT ( 'NONE',  ( 7.321193707744999557, 1516.534976163889951, 206.8301696586770220 ) ) ;
#11223=CARTESIAN_POINT ( 'NONE',  ( 12.20279393231724363, 1516.551704399888649, 226.2743875082219347 ) ) ;
#11232=CARTESIAN_POINT ( 'NONE',  ( 5.012317068235000228, 1517.020727862619879, 211.9902797687369969 ) ) ;
#11251=EDGE_CURVE ( 'NONE', #8432, #2864, #72211, .T. ) ;
#11260=CARTESIAN_POINT ( 'NONE',  ( 0.7369041709050019318, 1517.080322339569875, 204.1102945640870132 ) ) ;
#11269=DIRECTION ( 'NONE',  ( 0.7071067811865474617, -6.092092863024105611E-16, -0.7071067811865474617 ) ) ;
#11280=CARTESIAN_POINT ( 'NONE',  ( -6.338109935804999928, 1511.735270473989885, 201.5240551590069913 ) ) ;
#11288=ORIENTED_EDGE ( 'NONE', *, *, #54848, .F. ) ;
#11293=CARTESIAN_POINT ( 'NONE',  ( 15.27973127913499951, 1514.812393650459853, 224.9548174513670062 ) ) ;
#11302=CARTESIAN_POINT ( 'NONE',  ( -2.300729664794999962, 1516.923170579120097, 207.4211391557370234 ) ) ;
#11319=CARTESIAN_POINT ( 'NONE',  ( 5.567211196089225211, 1510.484595323987833, 216.6724604399022951 ) ) ;
#11356=CARTESIAN_POINT ( 'NONE',  ( -3.459156616214999591, 1516.769879638719885, 204.5118493505569859 ) ) ;
#11375=CARTESIAN_POINT ( 'NONE',  ( 7.336844642415000450, 1517.106845464700200, 212.5753907958570039 ) ) ;
#11385=CARTESIAN_POINT ( 'NONE',  ( -8.080850468484999993, 1512.335510084620182, 215.7195519849769880 ) ) ;
#11398=CARTESIAN_POINT ( 'NONE',  ( 2.282301578035000222, 1516.836638729160086, 207.4044134838369757 ) ) ;
#11404=CARTESIAN_POINT ( 'NONE',  ( -6.141356664424689527, 1509.034509698630018, 201.6091305267439964 ) ) ;
#11410=CARTESIAN_POINT ( 'NONE',  ( -6.099948008796559407, 1511.445028088800200, 201.4631254019980133 ) ) ;
#11412=CARTESIAN_POINT ( 'NONE',  ( 17.17760792425680094, 1517.051704368240053, 222.7507317666290305 ) ) ;
#11416=CARTESIAN_POINT ( 'NONE',  ( -2.289624470354999719, 1517.154223579619838, 215.6854418399169901 ) ) ;
#11418=CARTESIAN_POINT ( 'NONE',  ( 5.854887922672690870, 1510.764648358900104, 216.6679770094980313 ) ) ;
#11420=CARTESIAN_POINT ( 'NONE',  ( -6.547556969464999987, 1516.633288330999903, 212.3841106205370011 ) ) ;
#11436=CARTESIAN_POINT ( 'NONE',  ( -1.131796848745000084, 1516.659138130710289, 203.3488676535569937 ) ) ;
#11474=CARTESIAN_POINT ( 'NONE',  ( -14.32022880866499825, 1513.136578080079744, 193.2786756054669866 ) ) ;
#11481=CARTESIAN_POINT ( 'NONE',  ( 7.777794710095000674, 1511.980236064749988, 206.2293425532969877 ) ) ;
#11487=EDGE_LOOP ( 'NONE', ( #69112, #57440, #9452, #1174 ) ) ;
#11489=CARTESIAN_POINT ( 'NONE',  ( 8.537822598675001373, 1517.051704408389924, 212.5465662711270056 ) ) ;
#11507=ORIENTED_EDGE ( 'NONE', *, *, #89820, .T. ) ;
#11511=CARTESIAN_POINT ( 'NONE',  ( -4.612507312034999529, 1516.886345593249871, 214.1313240375470173 ) ) ;
#11512=CARTESIAN_POINT ( 'NONE',  ( 3.927225866655000619, 1511.005930286180046, 216.7576803329270092 ) ) ;
#11518=CARTESIAN_POINT ( 'NONE',  ( -7.334957394705000411, 1517.030858226499959, 204.5055736355369902 ) ) ;
#11521=CARTESIAN_POINT ( 'NONE',  ( 1.710012720495000194, 1517.232977404109988, 201.3945188173769907 ) ) ;
#11531=CARTESIAN_POINT ( 'NONE',  ( 2.879642153204999833, 1516.812046502680005, 212.5681757458869754 ) ) ;
#11537=CARTESIAN_POINT ( 'NONE',  ( -6.938478822895000064, 1516.719999691880048, 209.8757167055200057 ) ) ;
#11542=ORIENTED_EDGE ( 'NONE', *, *, #32444, .T. ) ;
#11550=CARTESIAN_POINT ( 'NONE',  ( -2.289624470354999719, 1517.154223579619838, 215.6854418399169901 ) ) ;
#11558=CARTESIAN_POINT ( 'NONE',  ( -15.78436440076501768, 1512.151624459629829, 220.2511651824670196 ) ) ;
#11560=CARTESIAN_POINT ( 'NONE',  ( 7.670153655591260389, 1511.304111283970087, 203.1182573986329771 ) ) ;
#11573=VERTEX_POINT ( 'NONE', #33459 ) ;
#11574=FACE_OUTER_BOUND ( 'NONE', #55271, .T. ) ;
#11589=CARTESIAN_POINT ( 'NONE',  ( -0.8697201140136210373, 1516.690597168679915, 201.4087215436879887 ) ) ;
#11595=ORIENTED_EDGE ( 'NONE', *, *, #106261, .T. ) ;
#11605=CARTESIAN_POINT ( 'NONE',  ( 12.18971934853500194, 1512.123542805230272, 223.8476153537669973 ) ) ;
#11628=ORIENTED_EDGE ( 'NONE', *, *, #63222, .T. ) ;
#11631=CARTESIAN_POINT ( 'NONE',  ( 6.951517132375000685, 1517.194816588360027, 210.2467400204669730 ) ) ;
#11632=CARTESIAN_POINT ( 'NONE',  ( 5.513435553965000402, 1508.551704408389924, 202.1089243864769855 ) ) ;
#11639=CARTESIAN_POINT ( 'NONE',  ( 3.453544825624999870, 1517.106845464700200, 201.7850012896870169 ) ) ;
#11645=CARTESIAN_POINT ( 'NONE',  ( 0.7402208603880020554, 1516.992029636990083, 208.3685455796920110 ) ) ;
#11662=CARTESIAN_POINT ( 'NONE',  ( -0.01327257453019850021, 1516.940252185109784, 206.2479269295770052 ) ) ;
#11678=CARTESIAN_POINT ( 'NONE',  ( -2.483322492024999661, 1517.139039350860003, 215.6851008610869940 ) ) ;
#11700=DIRECTION ( 'NONE',  ( -1.224646799147353207E-16, -6.123233995736769734E-17, -1.000000000000000000 ) ) ;
#11750=CARTESIAN_POINT ( 'NONE',  ( 2.864043418315000089, 1516.811292230880099, 206.8228319013669818 ) ) ;
#11771=CARTESIAN_POINT ( 'NONE',  ( 14.75869785433269676, 1514.537600265056653, 225.3978362136949158 ) ) ;
#11792=CARTESIAN_POINT ( 'NONE',  ( -6.946748557085000719, 1516.983995446890049, 204.1186252050270014 ) ) ;
#11796=CARTESIAN_POINT ( 'NONE',  ( 5.258165198517999350, 1511.418041552836030, 217.7311153980011795 ) ) ;
#11810=DIRECTION ( 'NONE',  ( -0.9996573249755517088, -0.02617694830808747070, 0.000000000000000000 ) ) ;
#11815=CARTESIAN_POINT ( 'NONE',  ( -6.372167638684999247, 1511.069621805459974, 201.7253008889670127 ) ) ;
#11826=ADVANCED_FACE ( 'NONE', ( #46746 ), #107019, .T. ) ;
#11831=CARTESIAN_POINT ( 'NONE',  ( 14.96248396073499976, 1513.868118914750085, 224.3717980193670201 ) ) ;
#11840=CARTESIAN_POINT ( 'NONE',  ( -6.951175166914999259, 1517.170721208160103, 206.8315896683770063 ) ) ;
#11859=CARTESIAN_POINT ( 'NONE',  ( 6.164039417708820245, 1510.821818217313648, 216.5878453126418037 ) ) ;
#11870=CARTESIAN_POINT ( 'NONE',  ( 7.550503318189189628, 1510.480349263560129, 203.5706572562480119 ) ) ;
#11896=CARTESIAN_POINT ( 'NONE',  ( 4.611879685325000366, 1516.858533673840157, 204.4999481076869756 ) ) ;
#11915=CARTESIAN_POINT ( 'NONE',  ( -4.996642198295000448, 1516.697242742309982, 211.9989590406970024 ) ) ;
#11923=FACE_OUTER_BOUND ( 'NONE', #72413, .T. ) ;
#11935=CARTESIAN_POINT ( 'NONE',  ( -1.718203501584999904, 1516.898441858519845, 207.4215862561470090 ) ) ;
#11941=CARTESIAN_POINT ( 'NONE',  ( -5.984315745076109749, 1508.551704607450120, 202.1093160777899982 ) ) ;
#11947=CARTESIAN_POINT ( 'NONE',  ( -5.987023825353920969, 1511.685461860059831, 200.6544365511240073 ) ) ;
#11953=CARTESIAN_POINT ( 'NONE',  ( -5.778372601744999670, 1516.932669162149978, 216.0673360190369863 ) ) ;
#11955=CARTESIAN_POINT ( 'NONE',  ( 5.943999021440889763, 1511.034527886640262, 216.7021439542070027 ) ) ;
#11957=CARTESIAN_POINT ( 'NONE',  ( -1.119439127814999990, 1517.026534522949987, 212.3908711059869745 ) ) ;
#11978=CARTESIAN_POINT ( 'NONE',  ( 3.254401403604999743, 1516.919782530640077, 205.0791161293069820 ) ) ;
#11986=CARTESIAN_POINT ( 'NONE',  ( -6.126746181595000174, 1514.923664147150021, 217.2480802176870043 ) ) ;
#12015=CARTESIAN_POINT ( 'NONE',  ( -14.10835369926500071, 1513.596256836700150, 192.4716710403669993 ) ) ;
#12018=CARTESIAN_POINT ( 'NONE',  ( -2.291047527245000381, 1516.524310051880093, 201.4130759250869858 ) ) ;
#12028=VERTEX_POINT ( 'NONE', #33477 ) ;
#12044=EDGE_LOOP ( 'NONE', ( #94679, #3550, #38083, #12324 ) ) ;
#12052=CARTESIAN_POINT ( 'NONE',  ( 3.456007385174999946, 1516.647534046129977, 215.6697273451470096 ) ) ;
#12053=CARTESIAN_POINT ( 'NONE',  ( 3.367054129315000033, 1511.558654537720031, 216.9757299529570105 ) ) ;
#12058=CARTESIAN_POINT ( 'NONE',  ( 3.255340926295000159, 1516.962555622980062, 204.4977466407669908 ) ) ;
#12060=CYLINDRICAL_SURFACE ( 'NONE', #105685, 1.000000000000003775 ) ;
#12069=CARTESIAN_POINT ( 'NONE',  ( -2.284526496774999860, 1516.956048353049937, 212.5847947667770086 ) ) ;
#12075=CARTESIAN_POINT ( 'NONE',  ( 1.715109447055000125, 1516.963431999339946, 209.8570730874349977 ) ) ;
#12088=CARTESIAN_POINT ( 'NONE',  ( 6.556022194504999234, 1516.833525648419936, 216.0623193043769845 ) ) ;
#12094=CARTESIAN_POINT ( 'NONE',  ( 1.708747624254999931, 1517.213554313520035, 202.1696795498070003 ) ) ;
#12095=CARTESIAN_POINT ( 'NONE',  ( -15.08013804596499874, 1512.195694528090144, 221.7327207927669974 ) ) ;
#12098=EDGE_CURVE ( 'NONE', #3729, #107968, #43018, .T. ) ;
#12101=CARTESIAN_POINT ( 'NONE',  ( 8.297057133861780898, 1511.753217516670247, 203.0771327291550108 ) ) ;
#12129=CARTESIAN_POINT ( 'NONE',  ( -0.5179933185710690058, 1516.784603496090085, 201.4062599077630011 ) ) ;
#12134=CARTESIAN_POINT ( 'NONE',  ( 14.69525441947700095, 1513.799047785610128, 224.1094165707140178 ) ) ;
#12173=CARTESIAN_POINT ( 'NONE',  ( -7.710967015764999211, 1516.608208975040043, 210.2506035313070072 ) ) ;
#12181=CARTESIAN_POINT ( 'NONE',  ( -1.708721022705000037, 1516.531533746980131, 201.8006767011069940 ) ) ;
#12190=VERTEX_POINT ( 'NONE', #99168 ) ;
#12202=CARTESIAN_POINT ( 'NONE',  ( -4.624736897314999595, 1516.994127245590107, 206.2540423059970180 ) ) ;
#12219=CARTESIAN_POINT ( 'NONE',  ( 4.038637462725000127, 1516.734985836460055, 214.8955147850770118 ) ) ;
#12228=CARTESIAN_POINT ( 'NONE',  ( 3.669386717837979983, 1517.051704638620095, 202.5807756278150009 ) ) ;
#12276=CARTESIAN_POINT ( 'NONE',  ( -3.330134203884999700, 1515.051704408389924, 204.7920544413669859 ) ) ;
#12287=CARTESIAN_POINT ( 'NONE',  ( -5.789394700334999477, 1517.164987839469859, 207.4150481461570052 ) ) ;
#12312=CARTESIAN_POINT ( 'NONE',  ( 11.80657790919278582, 1512.979858876890376, 225.6266235005796830 ) ) ;
#12324=ORIENTED_EDGE ( 'NONE', *, *, #66245, .F. ) ;
#12328=CARTESIAN_POINT ( 'NONE',  ( 1.704794803334999997, 1517.096587378560116, 204.4952540647470016 ) ) ;
#12331=CARTESIAN_POINT ( 'NONE',  ( 5.513435553965000402, 1508.551704408389924, 202.1089243864769855 ) ) ;
#12350=CARTESIAN_POINT ( 'NONE',  ( -6.867779409725000228, 1512.132770473870096, 201.9588434351270223 ) ) ;
#12368=CARTESIAN_POINT ( 'NONE',  ( 13.51662153773500030, 1512.620989416249813, 225.5656590752669786 ) ) ;
#12377=CARTESIAN_POINT ( 'NONE',  ( 2.476170596904999854, 1516.819260244609950, 207.4047612206870213 ) ) ;
#12397=CARTESIAN_POINT ( 'NONE',  ( 6.178095833435953033, 1510.835436364192674, 216.5837886796534804 ) ) ;
#12433=CARTESIAN_POINT ( 'NONE',  ( 2.479246847704999812, 1516.983612918759945, 205.0778556245070092 ) ) ;
#12438=CARTESIAN_POINT ( 'NONE',  ( 7.947250527635000950, 1514.433282224309778, 206.1243428727769924 ) ) ;
#12443=ORIENTED_EDGE ( 'NONE', *, *, #40559, .F. ) ;
#12445=ORIENTED_EDGE ( 'NONE', *, *, #43609, .T. ) ;
#12454=AXIS2_PLACEMENT_3D ( 'NONE', #1251, #44361, #1816 ) ;
#12467=ORIENTED_EDGE ( 'NONE', *, *, #72735, .T. ) ;
#12468=ORIENTED_EDGE ( 'NONE', *, *, #91161, .T. ) ;
#12470=CARTESIAN_POINT ( 'NONE',  ( -5.919280326385000457, 1513.965983108850196, 216.7636238285669776 ) ) ;
#12471=CARTESIAN_POINT ( 'NONE',  ( 16.78598026525966702, 1513.543684533296073, 195.9142244523475824 ) ) ;
#12478=CARTESIAN_POINT ( 'NONE',  ( -4.805077596034999843, 1510.399296111369949, 201.5734650597370035 ) ) ;
#12483=CARTESIAN_POINT ( 'NONE',  ( -3.463767296015000330, 1517.014196759610059, 207.4190915607570105 ) ) ;
#12495=CARTESIAN_POINT ( 'NONE',  ( -5.822794808474560213, 1511.432897564909808, 201.1850910160889896 ) ) ;
#12504=CARTESIAN_POINT ( 'NONE',  ( 4.036119644515000715, 1516.647924054489977, 216.4458205765370167 ) ) ;
#12507=CARTESIAN_POINT ( 'NONE',  ( 5.382074236615409291, 1511.451532973539770, 217.6102468295670178 ) ) ;
#12509=CARTESIAN_POINT ( 'NONE',  ( 0.01327253640020150012, 1516.940252185109784, 211.9957649727570015 ) ) ;
#12527=CARTESIAN_POINT ( 'NONE',  ( 3.447264348965000558, 1516.858765657450249, 205.6607986404769974 ) ) ;
#12554=CARTESIAN_POINT ( 'NONE',  ( 8.071166603322222244, 1511.586661999316902, 205.5159583346354282 ) ) ;
#12565=CARTESIAN_POINT ( 'NONE',  ( -11.25155674426499885, 1512.842772631639946, 192.9205417576670243 ) ) ;
#12570=CARTESIAN_POINT ( 'NONE',  ( 6.941727252324999320, 1516.882217593000178, 201.7906628411569727 ) ) ;
#12574=CARTESIAN_POINT ( 'NONE',  ( 6.252266454184999489, 1511.741868877540128, 217.9101624594169948 ) ) ;
#12587=AXIS2_PLACEMENT_3D ( 'NONE', #53165, #88407, #97350 ) ;
#12592=FILL_AREA_STYLE_COLOUR ( '', #71822 ) ;
#12606=CARTESIAN_POINT ( 'NONE',  ( -2.482067898354999969, 1517.099836525840146, 214.9099431973869798 ) ) ;
#12609=ORIENTED_EDGE ( 'NONE', *, *, #76897, .T. ) ;
#12613=CARTESIAN_POINT ( 'NONE',  ( -0.7564342523539989704, 1516.783665406140017, 204.5091745923169810 ) ) ;
#12629=CARTESIAN_POINT ( 'NONE',  ( -2.477986770365000257, 1516.922519270759949, 212.3907053662870226 ) ) ;
#12634=CARTESIAN_POINT ( 'NONE',  ( -7.718230792536809659, 1516.885624574970052, 209.2907034861239879 ) ) ;
#12635=CARTESIAN_POINT ( 'NONE',  ( -6.550870182235000172, 1516.727502608469877, 209.8762341530540141 ) ) ;
#12638=CARTESIAN_POINT ( 'NONE',  ( -5.513435911474870110, 1508.551704408389924, 202.1089243664339961 ) ) ;
#12648=CARTESIAN_POINT ( 'NONE',  ( 0.01073129396420149928, 1516.939491476980038, 216.4539099096770087 ) ) ;
#12649=CARTESIAN_POINT ( 'NONE',  ( -8.537822636805000087, 1517.051704408389924, 205.6971256312070011 ) ) ;
#12653=CARTESIAN_POINT ( 'NONE',  ( -7.330554171554999776, 1516.857992118400034, 201.7925428541169879 ) ) ;
#12684=CARTESIAN_POINT ( 'NONE',  ( 0.1086926021523879904, 1516.965532036659852, 201.4015232171759919 ) ) ;
#12688=CARTESIAN_POINT ( 'NONE',  ( 13.23930717780280020, 1512.526687531779999, 224.3998820107140091 ) ) ;
#12705=VECTOR ( 'NONE', #49096, 999.9999999999998863 ) ;
#12731=CARTESIAN_POINT ( 'NONE',  ( 5.788436334164999586, 1517.116049120239950, 211.4102033778369787 ) ) ;
#12739=CARTESIAN_POINT ( 'NONE',  ( -0.7533001734329990429, 1516.714320817460020, 201.7957737879569891 ) ) ;
#12744=VECTOR ( 'NONE', #107545, 1000.000000000000000 ) ;
#12750=ORIENTED_EDGE ( 'NONE', *, *, #11107, .F. ) ;
#12756=CARTESIAN_POINT ( 'NONE',  ( 1.137296650804999976, 1516.908147884120126, 210.8236964273370120 ) ) ;
#12757=VECTOR ( 'NONE', #41283, 1000.000000000000000 ) ;
#12762=CARTESIAN_POINT ( 'NONE',  ( 8.463742304414999751, 1511.382391139620040, 204.2973509411470161 ) ) ;
#12764=CARTESIAN_POINT ( 'NONE',  ( -5.012938901904998801, 1517.051603658920158, 206.6410320471169939 ) ) ;
#12781=CARTESIAN_POINT ( 'NONE',  ( 0.01244693565920149993, 1516.939646076049939, 214.9034317483770167 ) ) ;
#12783=CARTESIAN_POINT ( 'NONE',  ( 7.709236068321770219, 1516.542108215149938, 207.3618294337510122 ) ) ;
#12832=CARTESIAN_POINT ( 'NONE',  ( -7.012466319506879486, 1508.551704615640119, 214.6351047238229910 ) ) ;
#12844=CARTESIAN_POINT ( 'NONE',  ( -1.135898823814999847, 1516.958737650239982, 208.0022537503870126 ) ) ;
#12850=CYLINDRICAL_SURFACE ( 'NONE', #8599, 4.999999999999997335 ) ;
#12851=ORIENTED_EDGE ( 'NONE', *, *, #100073, .T. ) ;
#12865=CARTESIAN_POINT ( 'NONE',  ( 12.73370630486426869, 1513.317537406170231, 225.8919084108109701 ) ) ;
#12880=CARTESIAN_POINT ( 'NONE',  ( -3.487587049061890099, 1508.884219112060009, 204.6305577843690173 ) ) ;
#12882=CARTESIAN_POINT ( 'NONE',  ( -1.132949114555000136, 1516.693851263360102, 204.1241276937270186 ) ) ;
#12903=CARTESIAN_POINT ( 'NONE',  ( -6.098897551624999913, 1511.444830760690138, 201.4618419945269920 ) ) ;
#12906=FACE_OUTER_BOUND ( 'NONE', #49382, .T. ) ;
#12915=CARTESIAN_POINT ( 'NONE',  ( 12.15948096493499975, 1512.592133792520144, 225.7486201106670194 ) ) ;
#12922=CARTESIAN_POINT ( 'NONE',  ( -2.882326017515000061, 1516.969638403840008, 207.4201161117570109 ) ) ;
#12940=CARTESIAN_POINT ( 'NONE',  ( 6.343099782127201713, 1511.025938525906668, 216.5295357475528704 ) ) ;
#12960=CARTESIAN_POINT ( 'NONE',  ( 3.487592429471666033, 1508.909942010301620, 204.6312267328975452 ) ) ;
#12963=CARTESIAN_POINT ( 'NONE',  ( 3.229842584605000066, 1517.051704408389924, 200.7619551613470037 ) ) ;
#12965=LINE ( 'NONE', #71840, #98289 ) ;
#12973=CARTESIAN_POINT ( 'NONE',  ( 7.323034273964999841, 1516.609912606490070, 205.6670971239069843 ) ) ;
#12982=EDGE_LOOP ( 'NONE', ( #103564, #28910, #892, #89721 ) ) ;
#12987=CARTESIAN_POINT ( 'NONE',  ( 3.269025135755000200, 1517.026534522949987, 210.2412850599169758 ) ) ;
#13011=CARTESIAN_POINT ( 'NONE',  ( 4.608021669135000664, 1516.660388280709867, 207.4085285224269910 ) ) ;
#13021=CARTESIAN_POINT ( 'NONE',  ( -5.554947045494709634, 1511.433089852210060, 200.9123561315769848 ) ) ;
#13023=CARTESIAN_POINT ( 'NONE',  ( -5.551188713984379852, 1510.480349263560129, 201.5713426139130320 ) ) ;
#13027=CARTESIAN_POINT ( 'NONE',  ( 2.292940169014999974, 1516.565291103010168, 215.6678853655270132 ) ) ;
#13031=CARTESIAN_POINT ( 'NONE',  ( -4.997573825325000385, 1516.742629295279812, 212.5803724681170195 ) ) ;
#13047=CARTESIAN_POINT ( 'NONE',  ( 7.323034273964999841, 1516.609912606490070, 205.6670971239069843 ) ) ;
#13077=CARTESIAN_POINT ( 'NONE',  ( 8.353190717051095504, 1511.405768592756431, 204.6347806277314305 ) ) ;
#13080=( BOUNDED_CURVE ( )  B_SPLINE_CURVE ( 3, ( #101436, #17990, #8491, #67889 ),
 .UNSPECIFIED., .F., .T. ) 
 B_SPLINE_CURVE_WITH_KNOTS ( ( 4, 4 ),
 ( 4.286339028762302661, 4.712350959126750283 ),
 .UNSPECIFIED. ) 
 CURVE ( )  GEOMETRIC_REPRESENTATION_ITEM ( )  RATIONAL_B_SPLINE_CURVE ( ( 1.000000000000000000, 0.9849332492076060541, 0.9849332492076060541, 1.000000000000000000 ) ) 
 REPRESENTATION_ITEM ( '' )  );
#13089=CARTESIAN_POINT ( 'NONE',  ( -12.18971938666500066, 1512.123542805230272, 194.3960765485670095 ) ) ;
#13093=CARTESIAN_POINT ( 'NONE',  ( -6.556022232634999725, 1516.833525648419936, 202.1813725979570222 ) ) ;
#13128=CARTESIAN_POINT ( 'NONE',  ( -4.032397940005000514, 1516.981965530290154, 214.9074288837770155 ) ) ;
#13135=CARTESIAN_POINT ( 'NONE',  ( -3.265407155974999753, 1516.754149861460064, 204.5121726906670006 ) ) ;
#13146=EDGE_CURVE ( 'NONE', #81968, #33889, #64269, .T. ) ;
#13148=CARTESIAN_POINT ( 'NONE',  ( 2.298048923505000118, 1516.764084769670262, 212.5672535042169784 ) ) ;
#13153=CARTESIAN_POINT ( 'NONE',  ( -7.719573677055920236, 1516.936920898230028, 209.1135880942899803 ) ) ;
#13154=CARTESIAN_POINT ( 'NONE',  ( -2.476170635034999901, 1516.819260244609950, 210.8389306816469855 ) ) ;
#13168=CARTESIAN_POINT ( 'NONE',  ( 2.486474742745000022, 1516.560253536979872, 216.0557253731069807 ) ) ;
#13173=CARTESIAN_POINT ( 'NONE',  ( 2.872208710164999790, 1517.145312756229941, 201.7840522196070197 ) ) ;
#13174=CARTESIAN_POINT ( 'NONE',  ( -15.47073874116500036, 1511.939906524110256, 221.6147769341669971 ) ) ;
#13205=CARTESIAN_POINT ( 'NONE',  ( -4.802241272635000335, 1508.551704408389924, 213.5515886218640276 ) ) ;
#13215=CARTESIAN_POINT ( 'NONE',  ( 12.29919902959760059, 1512.135905030570029, 223.9492063288249994 ) ) ;
#13228=CARTESIAN_POINT ( 'NONE',  ( -7.861206937845000020, 1512.631076693560090, 196.3108915640669920 ) ) ;
#13256=CARTESIAN_POINT ( 'NONE',  ( 4.045182479925000685, 1517.057265928030120, 210.8256255754569963 ) ) ;
#13258=CARTESIAN_POINT ( 'NONE',  ( 2.880592928985000079, 1516.859514182039902, 211.9868180862470126 ) ) ;
#13267=CARTESIAN_POINT ( 'NONE',  ( 6.941100277744999936, 1516.858069504249897, 202.1782432786469883 ) ) ;
#13281=CARTESIAN_POINT ( 'NONE',  ( -7.326072182274999456, 1516.714320817460020, 209.8751461055349807 ) ) ;
#13286=CARTESIAN_POINT ( 'NONE',  ( 7.803201805185000062, 1511.730395268069969, 206.0441542149769987 ) ) ;
#13287=CARTESIAN_POINT ( 'NONE',  ( 0.7351097711180020200, 1516.977504706749869, 206.6301902066870184 ) ) ;
#13302=CARTESIAN_POINT ( 'NONE',  ( 4.620008207075000151, 1516.777260590120022, 214.8964555921769772 ) ) ;
#13304=CARTESIAN_POINT ( 'NONE',  ( 7.713820733194500789, 1516.717189502959855, 208.3559500364069947 ) ) ;
#13322=CARTESIAN_POINT ( 'NONE',  ( -7.012921583638330070, 1508.551704408389924, 203.6084103760139783 ) ) ;
#13333=CARTESIAN_POINT ( 'NONE',  ( -4.059671833654999951, 1511.437978678640093, 200.9086510787369946 ) ) ;
#13357=ADVANCED_FACE ( 'NONE', ( #46034 ), #8667, .F. ) ;
#13373=CARTESIAN_POINT ( 'NONE',  ( -7.447811320689449843, 1511.198033794599951, 215.3870677586729983 ) ) ;
#13377=CARTESIAN_POINT ( 'NONE',  ( -2.300729664794999962, 1516.923170579120097, 207.4211391557370234 ) ) ;
#13398=CARTESIAN_POINT ( 'NONE',  ( 14.39977812427909853, 1514.266850649818707, 225.6063674502700565 ) ) ;
#13404=VERTEX_POINT ( 'NONE', #65025 ) ;
#13405=CARTESIAN_POINT ( 'NONE',  ( 4.554954805175000843, 1508.731366866819826, 205.6342593439610198 ) ) ;
#13414=CARTESIAN_POINT ( 'NONE',  ( 6.937965660314999283, 1516.732530461250008, 204.1161457306970135 ) ) ;
#13423=CARTESIAN_POINT ( 'NONE',  ( -14.62991246550300062, 1513.722010160979835, 194.0917047335290135 ) ) ;
#13449=CARTESIAN_POINT ( 'NONE',  ( 14.32022877053500132, 1513.136578080079744, 224.9650162968669918 ) ) ;
#13481=DIRECTION ( 'NONE',  ( 0.02616798426532259553, -0.9993150019883517698, 0.02616798426532229369 ) ) ;
#13494=ORIENTED_EDGE ( 'NONE', *, *, #35346, .F. ) ;
#13508=CARTESIAN_POINT ( 'NONE',  ( -3.294781662986297377, 1511.738149259171223, 201.1454951801678135 ) ) ;
#13515=CARTESIAN_POINT ( 'NONE',  ( -6.948321743994999800, 1517.049325831759916, 205.0875650164470017 ) ) ;
#13530=CARTESIAN_POINT ( 'NONE',  ( -2.477975353594999763, 1516.839862955080207, 210.2583935552169976 ) ) ;
#13546=CARTESIAN_POINT ( 'NONE',  ( 16.25736642822587541, 1514.559393048426728, 194.3359286633053955 ) ) ;
#13557=CARTESIAN_POINT ( 'NONE',  ( 2.286472886424999906, 1516.883361325900069, 208.3638615500849767 ) ) ;
#13568=CARTESIAN_POINT ( 'NONE',  ( -5.586203269550379602, 1511.461696079649982, 200.4008954912939942 ) ) ;
#13574=CARTESIAN_POINT ( 'NONE',  ( 5.780861236055000241, 1516.783701990830195, 216.0610654530370027 ) ) ;
#13579=CARTESIAN_POINT ( 'NONE',  ( 0.01322035751810150123, 1516.939819969850078, 213.1588969678170145 ) ) ;
#13596=CARTESIAN_POINT ( 'NONE',  ( 4.028630584655000568, 1516.812923327049930, 205.6617440802170051 ) ) ;
#13605=CYLINDRICAL_SURFACE ( 'NONE', #71120, 7.500000000000000000 ) ;
#13625=CARTESIAN_POINT ( 'NONE',  ( 7.167383184274696006, 1508.551704408383557, 203.6084103738921272 ) ) ;
#13631=CARTESIAN_POINT ( 'NONE',  ( -7.494335721685672524, 1510.727597956327827, 215.1764273590825098 ) ) ;
#13634=CARTESIAN_POINT ( 'NONE',  ( -12.28497688116499909, 1512.406775501100128, 192.5826067984669976 ) ) ;
#13637=CARTESIAN_POINT ( 'NONE',  ( -2.485846037024999955, 1516.545806094630279, 201.8003900583769905 ) ) ;
#13644=CARTESIAN_POINT ( 'NONE',  ( -17.17760814124009983, 1517.051704413129983, 195.4929600000709797 ) ) ;
#13652=CARTESIAN_POINT ( 'NONE',  ( -7.803201843315000552, 1511.730395268069969, 212.1995376873570081 ) ) ;
#13672=CARTESIAN_POINT ( 'NONE',  ( 5.005700201405000271, 1516.732530461250008, 216.0598116305469887 ) ) ;
#13674=VECTOR ( 'NONE', #88619, 1000.000000000000114 ) ;
#13681=LINE ( 'NONE', #54644, #64354 ) ;
#13682=CARTESIAN_POINT ( 'NONE',  ( -3.267291643295000103, 1516.842852731759876, 205.6749038603869906 ) ) ;
#13684=CARTESIAN_POINT ( 'NONE',  ( -1.704170752255000032, 1516.927039499179955, 209.8797722570040207 ) ) ;
#13689=CARTESIAN_POINT ( 'NONE',  ( 6.742834585605000264, 1512.383155430650049, 217.4973484156870143 ) ) ;
#13697=CARTESIAN_POINT ( 'NONE',  ( 1.135185044044999980, 1516.778853242349896, 212.5689744308569971 ) ) ;
#13702=CARTESIAN_POINT ( 'NONE',  ( -7.709021946870369568, 1516.533929790709863, 211.5536301404889912 ) ) ;
#13703=( BOUNDED_CURVE ( )  B_SPLINE_CURVE ( 3, ( #82197, #105776, #47516, #13322 ),
 .UNSPECIFIED., .F., .F. ) 
 B_SPLINE_CURVE_WITH_KNOTS ( ( 4, 4 ),
 ( 5.498203534171459239, 7.068313952310489867 ),
 .UNSPECIFIED. ) 
 CURVE ( )  GEOMETRIC_REPRESENTATION_ITEM ( )  RATIONAL_B_SPLINE_CURVE ( ( 1.000000000000000000, 0.8048994966190576861, 0.8048994966190576861, 1.000000000000000000 ) ) 
 REPRESENTATION_ITEM ( '' )  );
#13704=CARTESIAN_POINT ( 'NONE',  ( 6.563915523884999992, 1517.184063036290127, 210.2461356256870033 ) ) ;
#13716=DIRECTION ( 'NONE',  ( -0.02616798426500960631, -0.9993150019883683122, 0.02616798426500965835 ) ) ;
#13720=CARTESIAN_POINT ( 'NONE',  ( 1.129386202275000084, 1516.613712827999962, 216.4452363774470030 ) ) ;
#13725=CARTESIAN_POINT ( 'NONE',  ( -4.035490750684999739, 1516.630499592039996, 201.4102952541169884 ) ) ;
#13726=CARTESIAN_POINT ( 'NONE',  ( -15.91746622356499863, 1512.594959757389915, 220.0895646873669875 ) ) ;
#13764=CARTESIAN_POINT ( 'NONE',  ( 14.49132057761110026, 1513.569700117019920, 224.2258521170180074 ) ) ;
#13786=ORIENTED_EDGE ( 'NONE', *, *, #4667, .T. ) ;
#13804=ORIENTED_EDGE ( 'NONE', *, *, #17385, .T. ) ;
#13805=CARTESIAN_POINT ( 'NONE',  ( 2.494020282435000180, 1516.876240617270014, 211.4047611534970201 ) ) ;
#13808=CARTESIAN_POINT ( 'NONE',  ( 6.948321705865000197, 1517.049325831759916, 213.1561268858870051 ) ) ;
#13817=CARTESIAN_POINT ( 'NONE',  ( 7.716878902974999122, 1516.833976295079992, 201.7919207096969672 ) ) ;
#13826=DIRECTION ( 'NONE',  ( 0.000000000000000000, -1.000000000000000000, 6.123233995736769734E-17 ) ) ;
#13828=DIRECTION ( 'NONE',  ( -0.9980967576068039415, 0.06164622171533089973, -0.001614249983439999900 ) ) ;
#13832=CARTESIAN_POINT ( 'NONE',  ( -4.031168805994999715, 1516.805675336850072, 209.8787446699039947 ) ) ;
#13840=CARTESIAN_POINT ( 'NONE',  ( -5.789394700334999477, 1517.164987839469859, 207.4150481461570052 ) ) ;
#13842=DIRECTION ( 'NONE',  ( 0.02616795315377970499, -0.9993150033772691954, 0.02616796233622665710 ) ) ;
#13848=EDGE_CURVE ( 'NONE', #44161, #2901, #96376, .T. ) ;
#13858=CARTESIAN_POINT ( 'NONE',  ( 2.291676273424999799, 1516.534976163889951, 216.4430396779769978 ) ) ;
#13860=CARTESIAN_POINT ( 'NONE',  ( 7.709114176761669768, 1516.537453364269822, 207.2981373406960017 ) ) ;
#13875=ORIENTED_EDGE ( 'NONE', *, *, #29200, .F. ) ;
#13882=PLANE ( 'NONE',  #12454 ) ;
#13905=CARTESIAN_POINT ( 'NONE',  ( -4.329791528864999961, 1515.051704408389924, 212.4519801359869859 ) ) ;
#13917=ORIENTED_EDGE ( 'NONE', *, *, #80887, .F. ) ;
#13928=CARTESIAN_POINT ( 'NONE',  ( -7.946770108222969142, 1511.532743959790196, 215.0475857338450396 ) ) ;
#13933=CARTESIAN_POINT ( 'NONE',  ( -5.788691363644999477, 1517.157901477309906, 207.9987443536870160 ) ) ;
#13964=CARTESIAN_POINT ( 'NONE',  ( 3.487587063703020185, 1509.038630936360050, 204.6345965708119934 ) ) ;
#13975=CARTESIAN_POINT ( 'NONE',  ( 7.323034273964999841, 1516.609912606490070, 205.6670971239069843 ) ) ;
#13983=CARTESIAN_POINT ( 'NONE',  ( -13.89676593410340111, 1513.004579589629884, 193.8317604122359796 ) ) ;
#14033=VERTEX_POINT ( 'NONE', #25962 ) ;
#14057=( BOUNDED_CURVE ( )  B_SPLINE_CURVE ( 3, ( #40790, #110749, #25067, #101776 ),
 .UNSPECIFIED., .F., .F. ) 
 B_SPLINE_CURVE_WITH_KNOTS ( ( 4, 4 ),
 ( 4.424456909735084764, 5.579818660943519859 ),
 .UNSPECIFIED. ) 
 CURVE ( )  GEOMETRIC_REPRESENTATION_ITEM ( )  RATIONAL_B_SPLINE_CURVE ( ( 1.000000000000000000, 0.8918208900458772792, 0.8918208900458772792, 1.000000000000000000 ) ) 
 REPRESENTATION_ITEM ( '' )  );
#14073=CARTESIAN_POINT ( 'NONE',  ( 1.119717716265000051, 1517.038650117239968, 205.6590103047369951 ) ) ;
#14076=ORIENTED_EDGE ( 'NONE', *, *, #96093, .F. ) ;
#14088=CARTESIAN_POINT ( 'NONE',  ( -3.253301419385000504, 1516.790374942449944, 210.2573062871869922 ) ) ;
#14116=CARTESIAN_POINT ( 'NONE',  ( -7.339749373344999661, 1517.224900789629828, 207.4124613591469881 ) ) ;
#14117=ORIENTED_EDGE ( 'NONE', *, *, #4240, .F. ) ;
#14119=AXIS2_PLACEMENT_3D ( 'NONE', #44820, #54328, #103595 ) ;
#14121=ORIENTED_EDGE ( 'NONE', *, *, #103630, .T. ) ;
#14122=AXIS2_PLACEMENT_3D ( 'NONE', #104679, #70013, #1138 ) ;
#14130=CARTESIAN_POINT ( 'NONE',  ( -6.372167638625000130, 1511.069621805459974, 201.7253008890070021 ) ) ;
#14135=AXIS2_PLACEMENT_3D ( 'NONE', #100961, #67959, #68506 ) ;
#14137=CARTESIAN_POINT ( 'NONE',  ( 1.708720984574999768, 1516.531533746980131, 216.4430152012269843 ) ) ;
#14138=VERTEX_POINT ( 'NONE', #804 ) ;
#14144=CARTESIAN_POINT ( 'NONE',  ( -0.7356989727169980231, 1517.020847257979995, 212.5827121409169820 ) ) ;
#14148=CARTESIAN_POINT ( 'NONE',  ( 3.487584963647319736, 1508.551704408610021, 213.9544597577999809 ) ) ;
#14149=ORIENTED_EDGE ( 'NONE', *, *, #108567, .F. ) ;
#14164=CARTESIAN_POINT ( 'NONE',  ( 7.323974606304999746, 1516.647924054489977, 205.0857262875869935 ) ) ;
#14183=CARTESIAN_POINT ( 'NONE',  ( 15.90990255763500016, 1513.492015765619954, 198.1616908427670296 ) ) ;
#14187=CARTESIAN_POINT ( 'NONE',  ( -3.793220392315020284, 1517.051709179979980, 215.8229393325320018 ) ) ;
#14191=CARTESIAN_POINT ( 'NONE',  ( 7.895892558453802224, 1512.040964529616303, 206.1210073478832783 ) ) ;
#14198=CARTESIAN_POINT ( 'NONE',  ( -7.541469379549965879, 1510.554407340499438, 214.8833459881294345 ) ) ;
#14207=CARTESIAN_POINT ( 'NONE',  ( -5.005700239535000762, 1516.732530461250008, 202.1838802717869896 ) ) ;
#14210=CARTESIAN_POINT ( 'NONE',  ( 15.91746618543499814, 1512.594959757389915, 198.1541272149669908 ) ) ;
#14220=CARTESIAN_POINT ( 'NONE',  ( -3.260378293283676232, 1516.582197291435023, 201.4115601429068079 ) ) ;
#14232=CARTESIAN_POINT ( 'NONE',  ( 8.375502445464999113, 1512.383155430630040, 202.3790113465069851 ) ) ;
#14237=ORIENTED_EDGE ( 'NONE', *, *, #105498, .F. ) ;
#14243=CARTESIAN_POINT ( 'NONE',  ( -4.615644842514999624, 1517.009964551830080, 216.0692237534070159 ) ) ;
#14250=CARTESIAN_POINT ( 'NONE',  ( -1.715704529104999931, 1516.757508073510053, 205.8704515699670026 ) ) ;
#14252=CARTESIAN_POINT ( 'NONE',  ( 4.042388501175000037, 1517.045004075700035, 209.8579434088520088 ) ) ;
#14265=CARTESIAN_POINT ( 'NONE',  ( 0.01322035751810150123, 1516.939819969850078, 213.1588969678170145 ) ) ;
#14269=CARTESIAN_POINT ( 'NONE',  ( -7.709377382076580076, 1516.547507499529956, 211.8130208532940060 ) ) ;
#14270=CARTESIAN_POINT ( 'NONE',  ( -3.251394400264999707, 1516.757508073510053, 210.8375504612070017 ) ) ;
#14285=CARTESIAN_POINT ( 'NONE',  ( 3.454748808194999743, 1516.609912606490070, 216.4448802441970088 ) ) ;
#14290=CARTESIAN_POINT ( 'NONE',  ( 5.778372563615000068, 1516.932669162149978, 202.1763558832970205 ) ) ;
#14317=DIRECTION ( 'NONE',  ( 0.7071067811865475727, 1.631342908290929267E-16, -0.7071067811865475727 ) ) ;
#14325=CARTESIAN_POINT ( 'NONE',  ( 14.08695216841010023, 1513.170547668200015, 224.3743395614490055 ) ) ;
#14344=ORIENTED_EDGE ( 'NONE', *, *, #96009, .F. ) ;
#14363=CARTESIAN_POINT ( 'NONE',  ( 2.299656316094999653, 1516.843453247299749, 211.5982966343670171 ) ) ;
#14365=CARTESIAN_POINT ( 'NONE',  ( 5.010422963235000360, 1516.929569650079884, 213.1529883219070030 ) ) ;
#14373=CARTESIAN_POINT ( 'NONE',  ( 4.615644804385000022, 1517.009964551830080, 202.1744681489270192 ) ) ;
#14388=CARTESIAN_POINT ( 'NONE',  ( 7.338411959395000572, 1517.170512887980067, 211.6064236274570192 ) ) ;
#14393=CARTESIAN_POINT ( 'NONE',  ( 7.890119370045001190, 1511.483345606789953, 205.5629819087669716 ) ) ;
#14394=CARTESIAN_POINT ( 'NONE',  ( -6.951175166914999259, 1517.170721208160103, 206.8315896683770063 ) ) ;
#14413=CARTESIAN_POINT ( 'NONE',  ( -0.7396922758749979732, 1517.135701590510052, 216.4591432822169850 ) ) ;
#14415=CARTESIAN_POINT ( 'NONE',  ( 7.716938320446660171, 1516.836245356829750, 208.7837035492700011 ) ) ;
#14443=CARTESIAN_POINT ( 'NONE',  ( -4.036380785655000025, 1511.355055856609852, 201.1360035737969838 ) ) ;
#14459=ADVANCED_FACE ( 'NONE', ( #82462 ), #74071, .F. ) ;
#14467=AXIS2_PLACEMENT_3D ( 'NONE', #62571, #54706, #44638 ) ;
#14477=ADVANCED_FACE ( 'NONE', ( #56154 ), #47756, .T. ) ;
#14491=CARTESIAN_POINT ( 'NONE',  ( -3.462835665494999660, 1517.038650117239968, 208.0021282158369900 ) ) ;
#14502=CARTESIAN_POINT ( 'NONE',  ( -15.26851443651900020, 1512.495155157800127, 222.3098048121690056 ) ) ;
#14518=CARTESIAN_POINT ( 'NONE',  ( 4.492644247030710858, 1508.880967439349888, 205.3188537370700146 ) ) ;
#14522=ADVANCED_FACE ( 'NONE', ( #24719 ), #16864, .T. ) ;
#14528=CARTESIAN_POINT ( 'NONE',  ( 2.284526458645000258, 1516.956048353049937, 205.6588971355569981 ) ) ;
#14538=CARTESIAN_POINT ( 'NONE',  ( -12.42116348050100072, 1512.160613316490071, 194.1975122379490131 ) ) ;
#14599=ADVANCED_FACE ( 'NONE', ( #56573 ), #82315, .F. ) ;
#14609=ORIENTED_EDGE ( 'NONE', *, *, #28120, .T. ) ;
#14633=CARTESIAN_POINT ( 'NONE',  ( -6.949265684145000677, 1517.089216728169959, 205.6689289091970068 ) ) ;
#14648=CARTESIAN_POINT ( 'NONE',  ( 6.952166382295000169, 1517.213554313520035, 210.8305935944869987 ) ) ;
#14661=CARTESIAN_POINT ( 'NONE',  ( -6.055196954515000840, 1514.134513140259969, 216.7673245375070223 ) ) ;
#14676=CARTESIAN_POINT ( 'NONE',  ( 5.778372563615000068, 1516.932669162149978, 202.1763558832970205 ) ) ;
#14677=CARTESIAN_POINT ( 'NONE',  ( 3.449647440015000122, 1516.829948096479939, 208.3645479958780129 ) ) ;
#14698=CARTESIAN_POINT ( 'NONE',  ( 0.8837376337392799375, 1516.687471173209360, 216.8348885015759038 ) ) ;
#14699=CARTESIAN_POINT ( 'NONE',  ( 3.460101851884999746, 1516.812923327049930, 213.1504765548870068 ) ) ;
#14717=CARTESIAN_POINT ( 'NONE',  ( 3.446942071715000111, 1516.842852731759876, 205.8545543269370057 ) ) ;
#14744=CARTESIAN_POINT ( 'NONE',  ( -4.380123784945419985, 1517.051697240460271, 216.5788674826960118 ) ) ;
#14748=CARTESIAN_POINT ( 'NONE',  ( 8.115348803788476673, 1511.538158271185011, 205.3742513834712611 ) ) ;
#14757=CARTESIAN_POINT ( 'NONE',  ( -14.87514316876499976, 1513.853571676670072, 194.0180321211670105 ) ) ;
#14761=CARTESIAN_POINT ( 'NONE',  ( 4.034280915654999689, 1517.049325831759916, 202.1735242262370207 ) ) ;
#14765=CARTESIAN_POINT ( 'NONE',  ( 15.82925651883499896, 1512.053076656670100, 196.3893797332669919 ) ) ;
#14798=CARTESIAN_POINT ( 'NONE',  ( 4.618119666265000589, 1516.706638732659940, 216.0591847158069925 ) ) ;
#14804=ORIENTED_EDGE ( 'NONE', *, *, #105498, .T. ) ;
#14805=CARTESIAN_POINT ( 'NONE',  ( 2.865588684285000021, 1516.890356958860139, 205.8536102114670143 ) ) ;
#14807=CARTESIAN_POINT ( 'NONE',  ( -7.719640941135000212, 1516.939452820819952, 209.1319487995289705 ) ) ;
#14818=CARTESIAN_POINT ( 'NONE',  ( -4.611879723454999969, 1516.858533673840157, 213.7437437946470027 ) ) ;
#14823=CARTESIAN_POINT ( 'NONE',  ( 6.952166382295000169, 1517.213554313520035, 210.8305935944869987 ) ) ;
#14837=CARTESIAN_POINT ( 'NONE',  ( -3.452917061035000401, 1517.089216728169959, 216.0711116162470091 ) ) ;
#14842=CARTESIAN_POINT ( 'NONE',  ( -5.781490582474999584, 1516.807958722750072, 202.5702025453269925 ) ) ;
#14843=CARTESIAN_POINT ( 'NONE',  ( -16.72999346986500058, 1513.736060322949925, 223.1141918444669727 ) ) ;
#14873=ORIENTED_EDGE ( 'NONE', *, *, #51415, .F. ) ;
#14901=EDGE_CURVE ( 'NONE', #64419, #42748, #48108, .T. ) ;
#14905=CARTESIAN_POINT ( 'NONE',  ( -7.713496591364999766, 1516.704809569559984, 214.3604687893070206 ) ) ;
#14913=CARTESIAN_POINT ( 'NONE',  ( 4.625359524845000792, 1517.025470194390209, 211.6020329869469947 ) ) ;
#14916=CARTESIAN_POINT ( 'NONE',  ( 4.042417777704999438, 1516.904492006980036, 212.5700528489170154 ) ) ;
#14920=ORIENTED_EDGE ( 'NONE', *, *, #34575, .F. ) ;
#14922=CARTESIAN_POINT ( 'NONE',  ( -0.7543882209519990889, 1516.727502608469877, 202.5709757879969857 ) ) ;
#14937=CARTESIAN_POINT ( 'NONE',  ( 4.044321679994999919, 1517.001127920769704, 211.4073335515969916 ) ) ;
#14942=CARTESIAN_POINT ( 'NONE',  ( -5.788436372295000076, 1517.116049120239950, 206.8334885244969712 ) ) ;
#14953=CARTESIAN_POINT ( 'NONE',  ( 15.93623140273500027, 1516.904916668740043, 224.2983129015669874 ) ) ;
#14959=CARTESIAN_POINT ( 'NONE',  ( -7.012921583605000286, 1508.551704408389924, 214.6352815282469919 ) ) ;
#14960=CARTESIAN_POINT ( 'NONE',  ( 0.01126491619350150110, 1516.939530130779985, 216.0663127125970107 ) ) ;
#14962=CARTESIAN_POINT ( 'NONE',  ( 7.709487153813650018, 1516.551696783219995, 206.3620776923469862 ) ) ;
#14980=CARTESIAN_POINT ( 'NONE',  ( -4.045182518055000287, 1517.057265928030120, 207.4180663268770104 ) ) ;
#15000=ORIENTED_EDGE ( 'NONE', *, *, #73545, .F. ) ;
#15002=CARTESIAN_POINT ( 'NONE',  ( -2.000000019065000245, 1520.551704408390151, 222.4523892994670007 ) ) ;
#15032=CARTESIAN_POINT ( 'NONE',  ( -1.133653179125000188, 1516.978425811520083, 208.3843950493249793 ) ) ;
#15041=CARTESIAN_POINT ( 'NONE',  ( -14.89373269229610131, 1512.150422497879845, 221.5012839471549739 ) ) ;
#15043=B_SPLINE_CURVE_WITH_KNOTS ( 'NONE', 5,
 ( #55946, #72744, #4440, #107426, #22850, #106871 ),
 .UNSPECIFIED., .F., .F.,
 ( 6, 6 ),
 ( 0.000000000000000000, 1.000000000000000000 ),
 .UNSPECIFIED. ) ;
#15048=CARTESIAN_POINT ( 'NONE',  ( 13.33054332923500063, 1517.051704408389924, 211.1218459511669892 ) ) ;
#15054=ORIENTED_EDGE ( 'NONE', *, *, #85786, .T. ) ;
#15059=CARTESIAN_POINT ( 'NONE',  ( 4.426499554645539902, 1508.728286212990042, 204.9620041230130312 ) ) ;
#15066=CARTESIAN_POINT ( 'NONE',  ( -4.487249399419609652, 1509.038630936360050, 205.6342588683990016 ) ) ;
#15068=CARTESIAN_POINT ( 'NONE',  ( -5.784638357945000031, 1516.939574742129935, 204.5080835752170003 ) ) ;
#15072=CARTESIAN_POINT ( 'NONE',  ( 15.30573751214310008, 1512.900351074040145, 195.3517817113319950 ) ) ;
#15076=EDGE_CURVE ( 'NONE', #66885, #78702, #96457, .T. ) ;
#15079=CARTESIAN_POINT ( 'NONE',  ( -13.83393990147829911, 1512.951873711579992, 193.8224831105249848 ) ) ;
#15132=ORIENTED_EDGE ( 'NONE', *, *, #40559, .T. ) ;
#15150=EDGE_LOOP ( 'NONE', ( #71746, #72518, #14076, #45593 ) ) ;
#15159=CARTESIAN_POINT ( 'NONE',  ( -4.963932502907999478, 1511.398736650825185, 200.6109342551562804 ) ) ;
#15166=CARTESIAN_POINT ( 'NONE',  ( -2.298369507954999946, 1516.779243033999819, 205.8702346062869992 ) ) ;
#15181=CARTESIAN_POINT ( 'NONE',  ( 0.7579262867720020225, 1516.927039499179955, 210.8260166843570005 ) ) ;
#15209=CARTESIAN_POINT ( 'NONE',  ( -2.872700555325000238, 1516.559109716219837, 201.4121646638069763 ) ) ;
#15210=CARTESIAN_POINT ( 'NONE',  ( -6.564578723344999922, 1517.199196846569976, 207.4137433428170141 ) ) ;
#15223=CARTESIAN_POINT ( 'NONE',  ( -5.768664141499007414, 1510.557600715827675, 201.5810540284795422 ) ) ;
#15230=CARTESIAN_POINT ( 'NONE',  ( 5.004442038985000174, 1516.690345681169902, 216.8349637732169697 ) ) ;
#15236=CARTESIAN_POINT ( 'NONE',  ( 2.067604332986444859, 1516.528072456315613, 216.8307144992771498 ) ) ;
#15237=CARTESIAN_POINT ( 'NONE',  ( -7.710285875814999912, 1516.582197289609894, 212.3822242253069987 ) ) ;
#15240=CARTESIAN_POINT ( 'NONE',  ( 4.487358445059079770, 1509.034524749680031, 212.9235806931369837 ) ) ;
#15255=CARTESIAN_POINT ( 'NONE',  ( -3.267603553834999897, 1516.858171774179937, 205.8687047948669999 ) ) ;
#15276=CARTESIAN_POINT ( 'NONE',  ( -14.79239591447758606, 1514.564605521402655, 192.8689679281645510 ) ) ;
#15302=CARTESIAN_POINT ( 'NONE',  ( 6.941100277744999936, 1516.858069504249897, 202.1782432786469883 ) ) ;
#15305=CARTESIAN_POINT ( 'NONE',  ( 15.08013800783500002, 1512.195694528090144, 196.5109711095670093 ) ) ;
#15318=CARTESIAN_POINT ( 'NONE',  ( -7.777794748224999388, 1511.980236064749988, 212.0143493490369906 ) ) ;
#15337=CARTESIAN_POINT ( 'NONE',  ( -1.708102627415000185, 1517.199196846569976, 215.6864246554469844 ) ) ;
#15345=CARTESIAN_POINT ( 'NONE',  ( 4.609673241434999902, 1516.754149861460064, 205.8564388142570181 ) ) ;
#15347=CARTESIAN_POINT ( 'NONE',  ( 7.337297311985000015, 1517.135701590510052, 209.8615382079770200 ) ) ;
#15361=CARTESIAN_POINT ( 'NONE',  ( 7.721907888235000073, 1517.026025493960105, 214.1263215447669950 ) ) ;
#15364=VECTOR ( 'NONE', #11269, 1000.000000000000114 ) ;
#15369=CARTESIAN_POINT ( 'NONE',  ( 3.463767257884999839, 1517.014196759610059, 210.8246003415769962 ) ) ;
#15372=( BOUNDED_CURVE ( )  B_SPLINE_CURVE ( 3, ( #91240, #56551, #40281, #22350 ),
 .UNSPECIFIED., .F., .F. ) 
 B_SPLINE_CURVE_WITH_KNOTS ( ( 4, 4 ),
 ( 2.001957627660153403E-12, 0.4510268114855987553 ),
 .UNSPECIFIED. ) 
 CURVE ( )  GEOMETRIC_REPRESENTATION_ITEM ( )  RATIONAL_B_SPLINE_CURVE ( ( 1.000000000000000000, 0.9831196230105689882, 0.9831196230105689882, 1.000000000000000000 ) ) 
 REPRESENTATION_ITEM ( '' )  );
#15388=CARTESIAN_POINT ( 'NONE',  ( -6.556022232634999725, 1516.833525648419936, 202.1813725979570222 ) ) ;
#15390=CARTESIAN_POINT ( 'NONE',  ( -16.52887565636499900, 1513.466724478469814, 223.3227970231669985 ) ) ;
#15407=CARTESIAN_POINT ( 'NONE',  ( -4.580855544014999836, 1515.987684277770086, 217.2759425653769938 ) ) ;
#15409=CARTESIAN_POINT ( 'NONE',  ( -3.487586739969820382, 1508.731366863229823, 213.6768007669170117 ) ) ;
#15418=CARTESIAN_POINT ( 'NONE',  ( 3.173602151875000388, 1510.830536680500245, 216.6815192743169973 ) ) ;
#15437=DIRECTION ( 'NONE',  ( 0.7063774289747313251, 0.04540766091858282338, 0.7063774289747313251 ) ) ;
#15457=ORIENTED_EDGE ( 'NONE', *, *, #878, .F. ) ;
#15461=CARTESIAN_POINT ( 'NONE',  ( -1.118353254094999860, 1516.977201124959947, 211.6155430111569729 ) ) ;
#15465=CARTESIAN_POINT ( 'NONE',  ( -1.119439127814999990, 1517.026534522949987, 212.3908711059869745 ) ) ;
#15471=CARTESIAN_POINT ( 'NONE',  ( 4.033653264325000265, 1517.028034847769959, 202.5611037067669997 ) ) ;
#15473=CARTESIAN_POINT ( 'NONE',  ( -7.526515395903619954, 1517.051704408389924, 208.6825894896870182 ) ) ;
#15479=ORIENTED_EDGE ( 'NONE', *, *, #86, .F. ) ;
#15485=CARTESIAN_POINT ( 'NONE',  ( -0.7350232362959980836, 1516.970035769810011, 211.4194755912870107 ) ) ;
#15490=CARTESIAN_POINT ( 'NONE',  ( -6.563595907815000352, 1517.154223579619838, 206.8322214998769937 ) ) ;
#15504=CARTESIAN_POINT ( 'NONE',  ( -1.704794841465000044, 1517.096587378560116, 213.7484378375869767 ) ) ;
#15507=CARTESIAN_POINT ( 'NONE',  ( -1.708747662384999977, 1517.213554313520035, 216.0740123525270064 ) ) ;
#15519=B_SPLINE_CURVE_WITH_KNOTS ( 'NONE', 3,
 ( #88479, #55437, #99055, #89567, #39723, #72246 ),
 .UNSPECIFIED., .F., .F.,
 ( 4, 2, 4 ),
 ( 0.000000000000000000, 0.5000000000000000000, 1.000000000000000000 ),
 .UNSPECIFIED. ) ;
#15576=CARTESIAN_POINT ( 'NONE',  ( 5.781585778145000631, 1516.939646076049939, 209.1093989964429909 ) ) ;
#15585=CARTESIAN_POINT ( 'NONE',  ( -15.16811422921670172, 1512.319979277489892, 221.9811700865099908 ) ) ;
#15588=CARTESIAN_POINT ( 'NONE',  ( 7.722580314247720068, 1517.051704408590012, 209.5565402419049974 ) ) ;
#15611=CARTESIAN_POINT ( 'NONE',  ( -2.877744984375000037, 1516.723920667490120, 204.5127816287269980 ) ) ;
#15614=CARTESIAN_POINT ( 'NONE',  ( 15.23581456386730082, 1513.231391185889834, 194.9678178315319883 ) ) ;
#15620=CARTESIAN_POINT ( 'NONE',  ( -13.46561928155499999, 1512.674009804160050, 193.8142106494929919 ) ) ;
#15671=PLANE ( 'NONE',  #79650 ) ;
#15695=CARTESIAN_POINT ( 'NONE',  ( 15.87603342115862581, 1512.359593911811089, 198.0975645610432707 ) ) ;
#15704=CARTESIAN_POINT ( 'NONE',  ( 2.864972116015000125, 1516.859514182039902, 206.2412530031170093 ) ) ;
#15715=CARTESIAN_POINT ( 'NONE',  ( -16.53955851760778373, 1513.001574290527287, 221.0043300851906451 ) ) ;
#15719=CARTESIAN_POINT ( 'NONE',  ( 5.012938863775000087, 1517.051603658920158, 211.6026598552170128 ) ) ;
#15739=CARTESIAN_POINT ( 'NONE',  ( 3.879787089154707491, 1516.685805519455926, 215.5416050467851221 ) ) ;
#15744=CARTESIAN_POINT ( 'NONE',  ( -4.036119682645000317, 1516.647924054489977, 201.7978713257969900 ) ) ;
#15745=CARTESIAN_POINT ( 'NONE',  ( -5.789394700334999477, 1517.164987839469859, 207.4150481461570052 ) ) ;
#15748=CARTESIAN_POINT ( 'NONE',  ( 4.822579926217737345, 1511.395344347225546, 217.5857078699854696 ) ) ;
#15765=CARTESIAN_POINT ( 'NONE',  ( 2.485845998894999909, 1516.545806094630279, 216.4433018439569878 ) ) ;
#15769=CARTESIAN_POINT ( 'NONE',  ( -4.999456428534999830, 1516.830644417779922, 213.7431138541670066 ) ) ;
#15772=CARTESIAN_POINT ( 'NONE',  ( 4.236980904132630066, 1508.610336716400070, 213.6558567133870099 ) ) ;
#15787=CARTESIAN_POINT ( 'NONE',  ( 2.284526458645000258, 1516.956048353049937, 205.6588971355569981 ) ) ;
#15829=CARTESIAN_POINT ( 'NONE',  ( -7.545803654736770838, 1510.531931302273733, 214.8296908414164363 ) ) ;
#15832=CARTESIAN_POINT ( 'NONE',  ( -15.21523573936500107, 1514.242353506929931, 194.1595280392670020 ) ) ;
#15836=CYLINDRICAL_SURFACE ( 'NONE', #14135, 2.999999999999996447 ) ;
#15839=CARTESIAN_POINT ( 'NONE',  ( 3.451033388965000004, 1517.025653221279981, 203.3353183697670090 ) ) ;
#15842=CARTESIAN_POINT ( 'NONE',  ( 16.62677414043499979, 1512.592133792520144, 196.9623649671669909 ) ) ;
#15865=CARTESIAN_POINT ( 'NONE',  ( -13.92686555291570194, 1517.051704405520013, 226.1812314194930025 ) ) ;
#15878=CARTESIAN_POINT ( 'NONE',  ( 5.780232077335000440, 1516.760434454289907, 216.4486414936069991 ) ) ;
#15880=B_SPLINE_SURFACE_WITH_KNOTS ( 'NONE', 5, 5, ( 
 ( #99355, #75301, #91532, #107224, #40019, #64703, #48996, #99912, #65790 ),
 ( #109444, #74198, #83129, #98268, #21539, #98820, #22082, #90968, #31613 ),
 ( #57407, #13689, #6426, #40571, #5317, #74742, #32173, #56278, #47874 ),
 ( #82012, #66357, #100476, #23758, #50095, #16986, #42235, #103215, #76947 ),
 ( #68557, #85315, #84767, #42787, #41680, #85885, #9188, #256, #33818 ),
 ( #101555, #16441, #75840, #59050, #92618, #110532, #8610, #102656, #51186 ),
 ( #34383, #15895, #109989, #58491, #25400, #67455, #84222, #68011, #34927 ),
 ( #77498, #59593, #8065, #43350, #94272, #33266, #7522, #76383, #25956 ),
 ( #24847, #93171, #17548, #60151, #93709, #51750, #798, #102121, #50637 ) ),
 .UNSPECIFIED., .F., .F., .F.,
 ( 6, 3, 6 ),
 ( 6, 3, 6 ),
 ( 3.580107477800000382, 6.558749095639999638, 9.700153431669999549 ),
 ( 0.000000000000000000, 0.5000000000000000000, 1.000000000000000000 ),
 .UNSPECIFIED. ) ;
#15881=VECTOR ( 'NONE', #100076, 1000.000000000000000 ) ;
#15890=CARTESIAN_POINT ( 'NONE',  ( 3.253462060665000433, 1516.874084700499907, 205.6604858388269861 ) ) ;
#15892=CARTESIAN_POINT ( 'NONE',  ( 3.267039691854999983, 1517.012231669750008, 209.8574146130079896 ) ) ;
#15895=CARTESIAN_POINT ( 'NONE',  ( 7.942826972685000264, 1514.298059036119867, 215.9745877768969819 ) ) ;
#15897=ORIENTED_EDGE ( 'NONE', *, *, #107452, .T. ) ;
#15904=CARTESIAN_POINT ( 'NONE',  ( 5.784008635194999748, 1516.911981270829983, 214.1231845985469988 ) ) ;
#15909=CARTESIAN_POINT ( 'NONE',  ( -7.721740324595189442, 1517.019662593890189, 208.8141823649340267 ) ) ;
#15910=CARTESIAN_POINT ( 'NONE',  ( 1.136814033864999907, 1516.854133554269993, 211.4058994415870245 ) ) ;
#15919=CARTESIAN_POINT ( 'NONE',  ( -5.563540966273840205, 1516.551188145990182, 218.9354434241149931 ) ) ;
#15925=CARTESIAN_POINT ( 'NONE',  ( 0.01010282929720150019, 1516.939452820819952, 216.8414868732370167 ) ) ;
#15930=CARTESIAN_POINT ( 'NONE',  ( -0.7543882209519990889, 1516.727502608469877, 202.5709757879969857 ) ) ;
#15931=CARTESIAN_POINT ( 'NONE',  ( 5.775165619278840978, 1509.036904577107407, 216.6345513647272298 ) ) ;
#15953=CARTESIAN_POINT ( 'NONE',  ( -4.987078467651929969, 1508.551704408389924, 212.6094300751769879 ) ) ;
#15957=CARTESIAN_POINT ( 'NONE',  ( -13.62888597016050163, 1517.051704413129983, 226.2994540733420195 ) ) ;
#15964=EDGE_CURVE ( 'NONE', #89576, #31839, #75067, .T. ) ;
#16010=CARTESIAN_POINT ( 'NONE',  ( 7.812463224191407818, 1516.551704356460050, 206.2591310155938515 ) ) ;
#16013=CARTESIAN_POINT ( 'NONE',  ( 2.491188358395000080, 1516.733363207009916, 213.1488973760370129 ) ) ;
#16020=CARTESIAN_POINT ( 'NONE',  ( 1.708102589285000139, 1517.199196846569976, 202.5572672468869939 ) ) ;
#16037=CARTESIAN_POINT ( 'NONE',  ( -7.321193745875000047, 1516.534976163889951, 211.4135222436570132 ) ) ;
#16042=CARTESIAN_POINT ( 'NONE',  ( 3.251611325815000342, 1516.779243033999819, 206.8234764622770001 ) ) ;
#16057=CARTESIAN_POINT ( 'NONE',  ( 2.296124850935000072, 1516.677239312369920, 213.7299927514870319 ) ) ;
#16060=CARTESIAN_POINT ( 'NONE',  ( 0.7538707352880020807, 1516.719999691880048, 216.0603247549969979 ) ) ;
#16078=EDGE_LOOP ( 'NONE', ( #13804, #110006, #14237, #21390 ) ) ;
#16131=CARTESIAN_POINT ( 'NONE',  ( -7.558249345183369883, 1510.689985724130111, 214.8113843319750060 ) ) ;
#16136=CARTESIAN_POINT ( 'NONE',  ( 7.332063939445000678, 1516.939491476980038, 209.1111146381379911 ) ) ;
#16170=CARTESIAN_POINT ( 'NONE',  ( -5.785582951674999919, 1516.981965530290154, 205.0894480302270040 ) ) ;
#16173=CARTESIAN_POINT ( 'NONE',  ( 14.81793322097859900, 1514.080593477140155, 194.2006236339620102 ) ) ;
#16199=CARTESIAN_POINT ( 'NONE',  ( -2.759740495412019712, 1516.551695078709827, 201.4123589199890034 ) ) ;
#16215=DIRECTION ( 'NONE',  ( 0.4999999999998399058, 0.7071067811867739472, 0.4999999999998399058 ) ) ;
#16239=CARTESIAN_POINT ( 'NONE',  ( 8.324963398134689996, 1511.468585895311890, 203.7405340362687411 ) ) ;
#16262=CARTESIAN_POINT ( 'NONE',  ( 5.772403774305000290, 1516.676340709600026, 205.8583240277470168 ) ) ;
#16266=CARTESIAN_POINT ( 'NONE',  ( -16.67046855446390197, 1516.551188146170034, 196.0483986024819956 ) ) ;
#16272=CARTESIAN_POINT ( 'NONE',  ( -16.31974137077875397, 1514.485057817183815, 223.8138502433834276 ) ) ;
#16276=CARTESIAN_POINT ( 'NONE',  ( 4.625693865015000128, 1517.042661899400173, 211.4082922958669997 ) ) ;
#16294=DIRECTION ( 'NONE',  ( 0.000000000000000000, -1.000000000000000000, 6.123233995736769734E-17 ) ) ;
#16302=CARTESIAN_POINT ( 'NONE',  ( 1.125509850285000280, 1517.203017563489766, 201.7827387294869936 ) ) ;
#16303=CARTESIAN_POINT ( 'NONE',  ( 2.486220101774999858, 1516.939658295650133, 209.1086089184300079 ) ) ;
#16308=CARTESIAN_POINT ( 'NONE',  ( 3.699323150121441639, 1511.553933485618018, 217.2221040787129027 ) ) ;
#16329=CARTESIAN_POINT ( 'NONE',  ( 7.334328272665000092, 1517.005755693489846, 214.1256940922069987 ) ) ;
#16348=CARTESIAN_POINT ( 'NONE',  ( 1.119439089684999944, 1517.026534522949987, 205.8528207963470038 ) ) ;
#16369=CARTESIAN_POINT ( 'NONE',  ( -14.69197387124563292, 1514.485034114827613, 192.8020852113455135 ) ) ;
#16384=CARTESIAN_POINT ( 'NONE',  ( -6.455447987151660350, 1508.551704612109916, 215.9494998419519902 ) ) ;
#16391=CARTESIAN_POINT ( 'NONE',  ( 7.889297498873377279, 1517.051704408389924, 211.8362768761033124 ) ) ;
#16393=CARTESIAN_POINT ( 'NONE',  ( -3.262264688434999726, 1516.633288330999903, 202.5742890007669814 ) ) ;
#16397=DIRECTION ( 'NONE',  ( 0.7063774289747313251, 0.04540766091858282338, 0.7063774289747313251 ) ) ;
#16409=CARTESIAN_POINT ( 'NONE',  ( -8.002723402924999618, 1516.551704408390151, 212.1748218667169965 ) ) ;
#16421=CARTESIAN_POINT ( 'NONE',  ( 7.777075013794999769, 1512.220794350750111, 202.5940153888870157 ) ) ;
#16430=CARTESIAN_POINT ( 'NONE',  ( 2.872700517194999748, 1516.559109716219837, 216.8315272385270021 ) ) ;
#16431=CARTESIAN_POINT ( 'NONE',  ( -7.910120449074414140, 1511.948750844499273, 212.1811042407670129 ) ) ;
#16436=CARTESIAN_POINT ( 'NONE',  ( -1.716392779905000054, 1516.788317650260069, 206.2580580763669786 ) ) ;
#16441=CARTESIAN_POINT ( 'NONE',  ( 7.809063913224999709, 1513.978875661350230, 216.3009730514370119 ) ) ;
#16449=CARTESIAN_POINT ( 'NONE',  ( 3.459156578084999989, 1516.769879638719885, 213.7318425517769924 ) ) ;
#16454=CARTESIAN_POINT ( 'NONE',  ( 0.01319650876840149957, 1516.941178807709775, 211.4140629809269853 ) ) ;
#16470=CARTESIAN_POINT ( 'NONE',  ( 11.92849869073500102, 1511.839858410419993, 224.1270719350669935 ) ) ;
#16476=CARTESIAN_POINT ( 'NONE',  ( -4.618749106614999711, 1516.729202374750002, 202.5720834851169911 ) ) ;
#16515=CARTESIAN_POINT ( 'NONE',  ( 6.795238182784275160, 1516.616925273614470, 205.9304268409078702 ) ) ;
#16532=CARTESIAN_POINT ( 'NONE',  ( 7.396545043095000160, 1511.069621805459974, 202.7496783316070150 ) ) ;
#16551=CARTESIAN_POINT ( 'NONE',  ( 2.295485501044999932, 1516.651306816259876, 214.1175719399469983 ) ) ;
#16554=ORIENTED_EDGE ( 'NONE', *, *, #56227, .T. ) ;
#16556=CARTESIAN_POINT ( 'NONE',  ( -1.710004586925000236, 1516.557392317769882, 202.5758445815369839 ) ) ;
#16563=LINE ( 'NONE', #85439, #110171 ) ;
#16570=CARTESIAN_POINT ( 'NONE',  ( -2.864043456445000135, 1516.811292230880099, 211.4208600009669965 ) ) ;
#16576=CARTESIAN_POINT ( 'NONE',  ( 3.449647440015000122, 1516.829948096479939, 208.3645479958780129 ) ) ;
#16590=CARTESIAN_POINT ( 'NONE',  ( -1.906499791370919845E-08, 1509.038615934239942, 213.6090957241370063 ) ) ;
#16592=CARTESIAN_POINT ( 'NONE',  ( -3.255967424474999650, 1516.989560013210166, 214.1335248082570217 ) ) ;
#16649=DIRECTION ( 'NONE',  ( -0.7384854939282339270, 8.827210057988519180E-16, 0.6742693640212139572 ) ) ;
#16671=CARTESIAN_POINT ( 'NONE',  ( -7.550412427349730393, 1510.476657126699820, 214.6722958288490020 ) ) ;
#16678=CARTESIAN_POINT ( 'NONE',  ( -4.618583430005000601, 1516.939762005280045, 209.1349059721700030 ) ) ;
#16687=CARTESIAN_POINT ( 'NONE',  ( -15.29490965391659962, 1512.594488815719842, 222.4682760166489857 ) ) ;
#16701=LINE ( 'NONE', #50901, #96737 ) ;
#16707=CARTESIAN_POINT ( 'NONE',  ( -3.910140144818339714, 1508.551704408389924, 204.2884083085430120 ) ) ;
#16709=CARTESIAN_POINT ( 'NONE',  ( 2.865588684285000021, 1516.890356958860139, 205.8536102114670143 ) ) ;
#16761=CARTESIAN_POINT ( 'NONE',  ( -2.866857931135000204, 1516.951766529250108, 213.1652121904069759 ) ) ;
#16803=CARTESIAN_POINT ( 'NONE',  ( 1.118903270415000151, 1517.003078582959688, 206.2405205581369785 ) ) ;
#16811=B_SPLINE_CURVE_WITH_KNOTS ( 'NONE', 3,
 ( #34555, #17722, #17163, #26136, #77130, #9906, #2090, #35658, #52484, #18840 ),
 .UNSPECIFIED., .F., .F.,
 ( 4, 2, 2, 2, 4 ),
 ( 0.000000000000000000, 0.2500000000000000000, 0.5000000000000000000, 0.7500000000000000000, 1.000000000000000000 ),
 .UNSPECIFIED. ) ;
#16814=CARTESIAN_POINT ( 'NONE',  ( -16.26362611520470836, 1514.552098283620808, 223.8986760177197368 ) ) ;
#16818=CARTESIAN_POINT ( 'NONE',  ( -0.7350232362959980836, 1516.970035769810011, 211.4194755912870107 ) ) ;
#16847=CARTESIAN_POINT ( 'NONE',  ( 3.259729297834999873, 1517.119374999550018, 201.7846921639870175 ) ) ;
#16848=CARTESIAN_POINT ( 'NONE',  ( 2.297629621054999571, 1516.970035769810011, 209.8568691683980205 ) ) ;
#16851=CARTESIAN_POINT ( 'NONE',  ( 4.993685203717481258, 1511.399999645683920, 217.6426921449797476 ) ) ;
#16864=CYLINDRICAL_SURFACE ( 'NONE', #71478, 0.5000000000000022204 ) ;
#16876=CARTESIAN_POINT ( 'NONE',  ( 3.958629193967660331, 1508.551704408389924, 214.1089270130739806 ) ) ;
#16891=CARTESIAN_POINT ( 'NONE',  ( -3.461047329755000401, 1516.858765657450249, 205.6745815831370123 ) ) ;
#16893=LINE ( 'NONE', #86888, #58922 ) ;
#16898=ADVANCED_FACE ( 'NONE', ( #3407, #88497 ), #56974, .T. ) ;
#16940=CARTESIAN_POINT ( 'NONE',  ( 7.713117802984999827, 1516.690345681169902, 204.1174038931170003 ) ) ;
#16966=CARTESIAN_POINT ( 'NONE',  ( 5.986375103784999929, 1514.050458741980037, 201.4853999038570009 ) ) ;
#16974=CARTESIAN_POINT ( 'NONE',  ( -2.291514335905000088, 1517.194972660189933, 216.8481778957070105 ) ) ;
#16975=CARTESIAN_POINT ( 'NONE',  ( -8.463898933797024071, 1511.395345385101564, 213.9445291291372939 ) ) ;
#16981=CARTESIAN_POINT ( 'NONE',  ( -2.299656354225000143, 1516.843453247299749, 206.6453952679669896 ) ) ;
#16986=CARTESIAN_POINT ( 'NONE',  ( 6.775684820614999992, 1512.341575225289944, 216.5029582879269867 ) ) ;
#16994=CARTESIAN_POINT ( 'NONE',  ( -5.775236830874999505, 1516.804776704140068, 214.1294346171470124 ) ) ;
#16998=CARTESIAN_POINT ( 'NONE',  ( 7.012466281656729805, 1508.551704615640119, 214.6351047168390096 ) ) ;
#16999=CARTESIAN_POINT ( 'NONE',  ( -0.7351098092479989576, 1516.977504706749869, 211.6135016956469883 ) ) ;
#17012=CARTESIAN_POINT ( 'NONE',  ( 12.07722019553499848, 1511.957228877180114, 223.9708055708669860 ) ) ;
#17018=CARTESIAN_POINT ( 'NONE',  ( -0.01171164408179850049, 1516.939568781210028, 202.5649949355269825 ) ) ;
#17034=CARTESIAN_POINT ( 'NONE',  ( -8.134103169834999036, 1515.224164712790071, 203.4316902230170001 ) ) ;
#17036=CARTESIAN_POINT ( 'NONE',  ( 14.72576938353500076, 1512.123542805230272, 196.9321265835669976 ) ) ;
#17038=CARTESIAN_POINT ( 'NONE',  ( -4.119399150550410837, 1508.879003890470131, 213.4915664277669975 ) ) ;
#17052=ORIENTED_EDGE ( 'NONE', *, *, #34365, .T. ) ;
#17058=CARTESIAN_POINT ( 'NONE',  ( 7.322103118964429669, 1516.556754281647045, 207.4728157223430571 ) ) ;
#17078=CARTESIAN_POINT ( 'NONE',  ( 7.494335682567689005, 1510.727597960018329, 203.0672645389179252 ) ) ;
#17087=CARTESIAN_POINT ( 'NONE',  ( -7.487063421429379417, 1517.051703294439903, 208.6815157772669806 ) ) ;
#17098=CARTESIAN_POINT ( 'NONE',  ( -1.121383629864999953, 1517.104192383289956, 213.7476359466970166 ) ) ;
#17101=ORIENTED_EDGE ( 'NONE', *, *, #24948, .F. ) ;
#17105=CARTESIAN_POINT ( 'NONE',  ( 2.287084270065000258, 1517.068517094990057, 204.1085709707169826 ) ) ;
#17115=ORIENTED_EDGE ( 'NONE', *, *, #96646, .T. ) ;
#17121=CARTESIAN_POINT ( 'NONE',  ( -2.283570671295000132, 1516.909589401870107, 212.0033943946770023 ) ) ;
#17125=CARTESIAN_POINT ( 'NONE',  ( 3.253301381255000013, 1516.790374942449944, 207.9863856151469861 ) ) ;
#17126=VERTEX_POINT ( 'NONE', #93844 ) ;
#17134=EDGE_CURVE ( 'NONE', #51148, #85474, #28812, .T. ) ;
#17141=CARTESIAN_POINT ( 'NONE',  ( 6.557909882634999299, 1516.908489800550115, 214.8995913655070069 ) ) ;
#17144=CARTESIAN_POINT ( 'NONE',  ( 4.616861508414999093, 1516.666407245520077, 216.8343369232169948 ) ) ;
#17145=ORIENTED_EDGE ( 'NONE', *, *, #61921, .F. ) ;
#17163=CARTESIAN_POINT ( 'NONE',  ( 7.460636164861699449, 1509.035273820331440, 203.0850866401826522 ) ) ;
#17213=B_SPLINE_CURVE_WITH_KNOTS ( 'NONE', 5,
 ( #22045, #53651, #104017, #22593, #21500, #14220, #72501, #29919, #4189, #30477, #90933, #27312, #10515, #106630, #107188 ),
 .UNSPECIFIED., .F., .F.,
 ( 6, 3, 3, 3, 6 ),
 ( 0.000000000000000000, 0.02279422308916183651, 0.2182353784632560800, 0.6091176892316280123, 1.000000000000000000 ),
 .UNSPECIFIED. ) ;
#17227=CARTESIAN_POINT ( 'NONE',  ( -5.011551406145000165, 1517.080322339569875, 208.3849417611969841 ) ) ;
#17237=CARTESIAN_POINT ( 'NONE',  ( -15.28467106619119953, 1512.548660307860018, 222.3969343260469884 ) ) ;
#17263=CARTESIAN_POINT ( 'NONE',  ( -5.786837717054999608, 1517.040132827679827, 205.8646253294070050 ) ) ;
#17313=CARTESIAN_POINT ( 'NONE',  ( -4.998515195425000002, 1516.787536375099990, 213.1617432482970003 ) ) ;
#17318=ORIENTED_EDGE ( 'NONE', *, *, #108128, .F. ) ;
#17358=CARTESIAN_POINT ( 'NONE',  ( 1.701729820345000199, 1516.969638403840008, 206.2395199527169893 ) ) ;
#17359=CIRCLE ( 'NONE', #38813, 0.9999999999999986677 ) ;
#17368=VERTEX_POINT ( 'NONE', #46800 ) ;
#17369=CARTESIAN_POINT ( 'NONE',  ( -16.25286372485815178, 1514.564622118826492, 223.9142624678142681 ) ) ;
#17373=CARTESIAN_POINT ( 'NONE',  ( 0.7578857918350010436, 1516.872851364150165, 211.6022732247369902 ) ) ;
#17382=VERTEX_POINT ( 'NONE', #80930 ) ;
#17385=EDGE_CURVE ( 'NONE', #110691, #98390, #98054, .T. ) ;
#17398=CARTESIAN_POINT ( 'NONE',  ( 1.949295068010844068, 1516.541277319971186, 216.3661146437771947 ) ) ;
#17403=CARTESIAN_POINT ( 'NONE',  ( 0.7386049046750020608, 1517.122674412569950, 202.5597518628069906 ) ) ;
#17404=CARTESIAN_POINT ( 'NONE',  ( 7.719640903004999721, 1516.939452820819952, 209.1117431028050078 ) ) ;
#17407=CARTESIAN_POINT ( 'NONE',  ( 3.179695852932951095, 1511.827406192486478, 217.0650637690530687 ) ) ;
#17414=CARTESIAN_POINT ( 'NONE',  ( -0.4392564938140909869, 1517.051704408389924, 216.6483608045730023 ) ) ;
#17439=CARTESIAN_POINT ( 'NONE',  ( -15.48184693596499883, 1513.486273623730085, 223.7694329180669968 ) ) ;
#17446=CARTESIAN_POINT ( 'NONE',  ( 0.7353365397730019515, 1516.995911393979895, 206.2425275143270085 ) ) ;
#17448=CARTESIAN_POINT ( 'NONE',  ( 7.512750208045280154, 1509.038615934079871, 214.6352815289239970 ) ) ;
#17460=CARTESIAN_POINT ( 'NONE',  ( -2.625066807925000134, 1511.873873588870083, 201.5029411752969963 ) ) ;
#17468=CARTESIAN_POINT ( 'NONE',  ( -13.24888725095132358, 1513.564944022936288, 192.3379340659209618 ) ) ;
#17496=CARTESIAN_POINT ( 'NONE',  ( 5.775236792744999903, 1516.804776704140068, 204.1142572851869943 ) ) ;
#17520=CARTESIAN_POINT ( 'NONE',  ( -6.933879441005000643, 1516.560253536979872, 211.6083207129769903 ) ) ;
#17524=CARTESIAN_POINT ( 'NONE',  ( 6.470331875434999880, 1513.423632355030122, 201.6536730834770026 ) ) ;
#17533=CARTESIAN_POINT ( 'NONE',  ( -6.941727290454999810, 1516.882217593000178, 216.4530290611770056 ) ) ;
#17535=CARTESIAN_POINT ( 'NONE',  ( -7.887702616237564079, 1512.266405701032454, 212.0598010800264888 ) ) ;
#17542=CARTESIAN_POINT ( 'NONE',  ( 7.322105067625000352, 1516.572193931679976, 206.2485165713470110 ) ) ;
#17548=CARTESIAN_POINT ( 'NONE',  ( 7.962346576125000297, 1514.830240247470101, 215.1813356062270088 ) ) ;
#17550=ORIENTED_EDGE ( 'NONE', *, *, #100780, .F. ) ;
#17558=CARTESIAN_POINT ( 'NONE',  ( 4.618749068485000109, 1516.729202374750002, 215.6716084172169872 ) ) ;
#17562=CARTESIAN_POINT ( 'NONE',  ( 5.513222314298020343, 1508.611138448550037, 216.4434734792089898 ) ) ;
#17563=CARTESIAN_POINT ( 'NONE',  ( -6.933616859135000254, 1516.548716157039962, 211.4141532006069895 ) ) ;
#17581=CARTESIAN_POINT ( 'NONE',  ( 2.286446325635000054, 1517.042661899400173, 204.4961520670869959 ) ) ;
#17600=CARTESIAN_POINT ( 'NONE',  ( -4.487358476232119919, 1509.034524880150002, 212.9235703428400086 ) ) ;
#17604=CARTESIAN_POINT ( 'NONE',  ( -1.906499846882070084E-08, 1517.051704408389924, 209.1218459511669892 ) ) ;
#17619=CARTESIAN_POINT ( 'NONE',  ( 7.245172990059893792, 1516.542928138167781, 207.1721856874727905 ) ) ;
#17634=ADVANCED_FACE ( 'NONE', ( #71902 ), #25518, .T. ) ;
#17637=CARTESIAN_POINT ( 'NONE',  ( 7.544470622717365238, 1510.539524131637791, 203.3949290437643072 ) ) ;
#17646=PLANE ( 'NONE',  #2025 ) ;
#17660=CARTESIAN_POINT ( 'NONE',  ( 4.039897278065000208, 1516.787536375099990, 214.1203611275269907 ) ) ;
#17665=CARTESIAN_POINT ( 'NONE',  ( -1.132949114555000136, 1516.693851263360102, 204.1241276937270186 ) ) ;
#17679=CARTESIAN_POINT ( 'NONE',  ( 1.716392741775000008, 1516.788317650260069, 211.9856338259669997 ) ) ;
#17681=CARTESIAN_POINT ( 'NONE',  ( -3.267039729984999585, 1517.012231669750008, 208.3862772893259887 ) ) ;
#17688=( GEOMETRIC_REPRESENTATION_CONTEXT ( 3 ) GLOBAL_UNCERTAINTY_ASSIGNED_CONTEXT ( ( #34543 ) ) GLOBAL_UNIT_ASSIGNED_CONTEXT ( ( #96849, #61062, #35829 ) ) REPRESENTATION_CONTEXT ( 'NONE', 'WORKASPACE' ) );
#17698=CARTESIAN_POINT ( 'NONE',  ( 2.877744946244999991, 1516.723920667490120, 213.7309102736070088 ) ) ;
#17701=CARTESIAN_POINT ( 'NONE',  ( 2.485217193935000068, 1516.534320418310244, 216.8308781079170160 ) ) ;
#17722=CARTESIAN_POINT ( 'NONE',  ( 7.512705394502938283, 1509.036904577181758, 203.3466803227199193 ) ) ;
#17737=CARTESIAN_POINT ( 'NONE',  ( -1.660008066423290130, 1516.550879573519751, 201.4123801776780169 ) ) ;
#17769=VECTOR ( 'NONE', #16649, 1000.000000000000114 ) ;
#17776=( BOUNDED_CURVE ( )  B_SPLINE_CURVE ( 3, ( #32605, #26389, #67328, #86307 ),
 .UNSPECIFIED., .F., .F. ) 
 B_SPLINE_CURVE_WITH_KNOTS ( ( 4, 4 ),
 ( 1.144704971675025273, 1.570796326799507314 ),
 .UNSPECIFIED. ) 
 CURVE ( )  GEOMETRIC_REPRESENTATION_ITEM ( )  RATIONAL_B_SPLINE_CURVE ( ( 1.000000000000000000, 0.9849276519253457041, 0.9849276519253457041, 1.000000000000000000 ) ) 
 REPRESENTATION_ITEM ( '' )  );
#17777=CARTESIAN_POINT ( 'NONE',  ( -8.210436200376010518, 1511.433570353809955, 214.6767451177750274 ) ) ;
#17785=CARTESIAN_POINT ( 'NONE',  ( -4.612671377915000370, 1516.783665406140017, 209.8782801844560026 ) ) ;
#17801=CARTESIAN_POINT ( 'NONE',  ( 4.997718238375000510, 1516.693851263360102, 207.9888968556769839 ) ) ;
#17818=CARTESIAN_POINT ( 'NONE',  ( 3.252530615595000452, 1516.827328999679821, 206.2418890071470230 ) ) ;
#17823=ORIENTED_EDGE ( 'NONE', *, *, #59405, .F. ) ;
#17824=CARTESIAN_POINT ( 'NONE',  ( 4.730384163222276506, 1508.603735221688339, 212.6094383991669758 ) ) ;
#17844=EDGE_CURVE ( 'NONE', #29094, #71004, #31485, .T. ) ;
#17873=CARTESIAN_POINT ( 'NONE',  ( -6.935457963315000640, 1516.627618683580067, 212.5772239474869991 ) ) ;
#17874=EDGE_CURVE ( 'NONE', #323, #3290, #97845, .T. ) ;
#17914=CARTESIAN_POINT ( 'NONE',  ( -5.258175134983901877, 1511.418042823260521, 200.5125726690029637 ) ) ;
#17915=CARTESIAN_POINT ( 'NONE',  ( -6.916946890995543384, 1516.591588929718000, 212.0217231930357968 ) ) ;
#17919=CARTESIAN_POINT ( 'NONE',  ( 3.251888829344999898, 1516.793978928989873, 206.6294022811970024 ) ) ;
#17932=CARTESIAN_POINT ( 'NONE',  ( 6.563595869685000750, 1517.154223579619838, 211.4114704024570131 ) ) ;
#17939=CARTESIAN_POINT ( 'NONE',  ( 2.862715419362055869, 1516.551704408386058, 216.9343088578988841 ) ) ;
#17957=CARTESIAN_POINT ( 'NONE',  ( 6.551899150602929822, 1508.551566291330118, 202.1600032511879874 ) ) ;
#17963=CARTESIAN_POINT ( 'NONE',  ( -3.261635970955000019, 1516.613881697390070, 202.1867125516770045 ) ) ;
#17964=CARTESIAN_POINT ( 'NONE',  ( -2.286472924554999953, 1516.883361325900069, 209.8798303522490016 ) ) ;
#17990=CARTESIAN_POINT ( 'NONE',  ( 16.95839603458921729, 1517.034034081944128, 223.2333545903914285 ) ) ;
#17995=( BOUNDED_CURVE ( )  B_SPLINE_CURVE ( 3, ( #87937, #44276, #18477, #78990 ),
 .UNSPECIFIED., .F., .T. ) 
 B_SPLINE_CURVE_WITH_KNOTS ( ( 4, 4 ),
 ( 5.447131716497384701, 6.315249268837864527 ),
 .UNSPECIFIED. ) 
 CURVE ( )  GEOMETRIC_REPRESENTATION_ITEM ( )  RATIONAL_B_SPLINE_CURVE ( ( 1.000000000000000000, 0.9381775213690333182, 0.9381775213690333182, 1.000000000000000000 ) ) 
 REPRESENTATION_ITEM ( '' )  );
#18008=CARTESIAN_POINT ( 'NONE',  ( -16.89844956606500048, 1513.192861445620110, 222.1868582675669757 ) ) ;
#18013=CARTESIAN_POINT ( 'NONE',  ( 1.118353215965000036, 1516.977201124959947, 206.6281488911770055 ) ) ;
#18015=CARTESIAN_POINT ( 'NONE',  ( 7.012921545624998920, 1508.551704408389924, 214.6352815241970120 ) ) ;
#18017=EDGE_CURVE ( 'NONE', #14033, #90411, #23081, .T. ) ;
#18031=CARTESIAN_POINT ( 'NONE',  ( -2.838447005044999916, 1511.534866634170157, 201.5062903025470007 ) ) ;
#18066=CARTESIAN_POINT ( 'NONE',  ( -3.263521942484999716, 1516.676340709600026, 203.3494421577970002 ) ) ;
#18089=CARTESIAN_POINT ( 'NONE',  ( -5.770883602015000058, 1516.603620185149794, 211.4160555996369908 ) ) ;
#18093=CARTESIAN_POINT ( 'NONE',  ( 6.557434856144999991, 1513.513616978020082, 201.6636742605270172 ) ) ;
#18099=CARTESIAN_POINT ( 'NONE',  ( -7.072298227815000615, 1512.974587999920004, 216.2923917488670043 ) ) ;
#18102=CARTESIAN_POINT ( 'NONE',  ( 0.01010282929720150019, 1516.939452820819952, 216.8414868732370167 ) ) ;
#18110=CARTESIAN_POINT ( 'NONE',  ( -7.725372170364999569, 1517.158319634930194, 206.2490093095770192 ) ) ;
#18121=CARTESIAN_POINT ( 'NONE',  ( -6.170974612161120199, 1511.326458810320219, 201.5850279059119714 ) ) ;
#18127=CARTESIAN_POINT ( 'NONE',  ( -2.288357445734999995, 1517.116049120239950, 214.9102823043970147 ) ) ;
#18131=CARTESIAN_POINT ( 'NONE',  ( 2.299983577604999940, 1516.861367446839949, 211.4044688825970013 ) ) ;
#18151=CARTESIAN_POINT ( 'NONE',  ( 7.325541787135000149, 1516.710692850270107, 204.1167749238070144 ) ) ;
#18191=CARTESIAN_POINT ( 'NONE',  ( 7.179997236714190656, 1516.543639203995554, 206.9492468735227533 ) ) ;
#18225=CARTESIAN_POINT ( 'NONE',  ( -7.711550716115000093, 1516.630499592039996, 213.1573366827869904 ) ) ;
#18226=CARTESIAN_POINT ( 'NONE',  ( 2.475398936714999998, 1511.813148765560072, 216.7072503566170099 ) ) ;
#18231=CARTESIAN_POINT ( 'NONE',  ( 0.7369041709050019318, 1517.080322339569875, 204.1102945640870132 ) ) ;
#18245=CARTESIAN_POINT ( 'NONE',  ( 5.787476994515000861, 1517.070197312179971, 211.9915394291670054 ) ) ;
#18251=CARTESIAN_POINT ( 'NONE',  ( -1.135898823814999847, 1516.958737650239982, 208.0022537503870126 ) ) ;
#18259=DIRECTION ( 'NONE',  ( -3.659266894335750173E-33, -6.123233995736769734E-17, -1.000000000000000000 ) ) ;
#18268=CARTESIAN_POINT ( 'NONE',  ( -5.001338666445000136, 1516.911981270829983, 214.9058546054269812 ) ) ;
#18271=CARTESIAN_POINT ( 'NONE',  ( -3.454172653555000139, 1517.122088787240045, 216.8462693643270143 ) ) ;
#18342=CARTESIAN_POINT ( 'NONE',  ( -8.380780172617267709, 1511.478807872990046, 214.6783014743539866 ) ) ;
#18349=CARTESIAN_POINT ( 'NONE',  ( 2.299667965875000331, 1516.965971551240045, 210.2399506998270056 ) ) ;
#18357=CARTESIAN_POINT ( 'NONE',  ( -15.30900801332620098, 1512.850289816019767, 222.8271770998339889 ) ) ;
#18364=CARTESIAN_POINT ( 'NONE',  ( -3.460866208815000178, 1517.020847257979995, 208.3861469975149987 ) ) ;
#18379=CARTESIAN_POINT ( 'NONE',  ( -2.298369507954999946, 1516.779243033999819, 205.8702346062869992 ) ) ;
#18396=DIRECTION ( 'NONE',  ( 0.000000000000000000, 1.000000000000000000, -6.123233995736769734E-17 ) ) ;
#18398=CARTESIAN_POINT ( 'NONE',  ( -1.121383629864999953, 1517.104192383289956, 213.7476359466970166 ) ) ;
#18404=CARTESIAN_POINT ( 'NONE',  ( 4.590060377064090424, 1517.051704403100075, 201.3992656192910147 ) ) ;
#18423=CARTESIAN_POINT ( 'NONE',  ( 5.009478067315000338, 1516.886345593249871, 213.7343532441369973 ) ) ;
#18469=CARTESIAN_POINT ( 'NONE',  ( -1.136814071995000175, 1516.854133554269993, 206.8377924607469822 ) ) ;
#18477=CARTESIAN_POINT ( 'NONE',  ( 13.29425500587429099, 1516.551188142742603, 192.2497704072501108 ) ) ;
#18478=EDGE_CURVE ( 'NONE', #46912, #42405, #49698, .T. ) ;
#18483=CARTESIAN_POINT ( 'NONE',  ( -4.609064341505000328, 1516.723920667490120, 211.9995909164769898 ) ) ;
#18498=ORIENTED_EDGE ( 'NONE', *, *, #55754, .T. ) ;
#18506=CARTESIAN_POINT ( 'NONE',  ( 7.512716716675900130, 1509.034509426269778, 202.9804468418519718 ) ) ;
#18511=CARTESIAN_POINT ( 'NONE',  ( -2.292307268505000106, 1516.548716157039962, 202.1882291110970300 ) ) ;
#18512=CARTESIAN_POINT ( 'NONE',  ( 2.491655725414999800, 1516.977504706749869, 209.8569557413499922 ) ) ;
#18517=CARTESIAN_POINT ( 'NONE',  ( 3.801724495280383476, 1509.034510030706542, 213.6092049197077358 ) ) ;
#18554=CARTESIAN_POINT ( 'NONE',  ( -16.64927610386499879, 1512.799725290110018, 221.1696797412670037 ) ) ;
#18558=CARTESIAN_POINT ( 'NONE',  ( 7.321455873725000174, 1516.545806094630279, 206.6359999332069890 ) ) ;
#18573=CARTESIAN_POINT ( 'NONE',  ( -2.392017086155000083, 1512.336926113599930, 201.5227265233669982 ) ) ;
#18594=EDGE_CURVE ( 'NONE', #2720, #10258, #17359, .T. ) ;
#18598=CARTESIAN_POINT ( 'NONE',  ( -6.081399352906980305, 1508.610505977480216, 216.4418972120009812 ) ) ;
#18608=CARTESIAN_POINT ( 'NONE',  ( 0.7365611785030020675, 1517.066898074209803, 204.4979538714769944 ) ) ;
#18615=ORIENTED_EDGE ( 'NONE', *, *, #65043, .F. ) ;
#18624=( BOUNDED_CURVE ( )  B_SPLINE_CURVE ( 3, ( #19700, #1831, #2938, #37057 ),
 .UNSPECIFIED., .F., .F. ) 
 B_SPLINE_CURVE_WITH_KNOTS ( ( 4, 4 ),
 ( 0.9036827175325773398, 1.148836376245267354 ),
 .UNSPECIFIED. ) 
 CURVE ( )  GEOMETRIC_REPRESENTATION_ITEM ( )  RATIONAL_B_SPLINE_CURVE ( ( 1.000000000000000000, 0.9949979080785074093, 0.9949979080785074093, 1.000000000000000000 ) ) 
 REPRESENTATION_ITEM ( '' )  );
#18634=CARTESIAN_POINT ( 'NONE',  ( -4.609673279564999504, 1516.754149861460064, 212.3872530880769887 ) ) ;
#18637=CARTESIAN_POINT ( 'NONE',  ( 6.852741806675000547, 1514.298059036119867, 201.1790189594169931 ) ) ;
#18645=CARTESIAN_POINT ( 'NONE',  ( -7.263042217704999359, 1512.240414293150025, 215.9313971026869865 ) ) ;
#18648=CARTESIAN_POINT ( 'NONE',  ( 0.7533001353030019942, 1516.714320817460020, 216.4479181143769893 ) ) ;
#18656=CARTESIAN_POINT ( 'NONE',  ( 1.701729820345000199, 1516.969638403840008, 206.2395199527169893 ) ) ;
#18665=CARTESIAN_POINT ( 'NONE',  ( -6.265221826568949659, 1511.198033794599951, 201.6740346495409995 ) ) ;
#18674=CARTESIAN_POINT ( 'NONE',  ( 6.944231748164999551, 1516.882690742909972, 215.6753703478370028 ) ) ;
#18676=CARTESIAN_POINT ( 'NONE',  ( 5.910253135570970429, 1511.600194708689969, 217.7510657911269902 ) ) ;
#18678=CARTESIAN_POINT ( 'NONE',  ( 1.136004274065000041, 1516.815173273089840, 211.9874827793370287 ) ) ;
#18695=CARTESIAN_POINT ( 'NONE',  ( -3.263521942484999716, 1516.676340709600026, 203.3494421577970002 ) ) ;
#18731=ORIENTED_EDGE ( 'NONE', *, *, #96197, .F. ) ;
#18741=CARTESIAN_POINT ( 'NONE',  ( 4.034908559714999399, 1517.068717944079935, 201.7859449365070077 ) ) ;
#18744=CARTESIAN_POINT ( 'NONE',  ( -5.496430460230245174, 1510.805212306242311, 201.5628357701014011 ) ) ;
#18753=CARTESIAN_POINT ( 'NONE',  ( -7.564413999595000604, 1511.011611623900080, 212.4015039894770212 ) ) ;
#18773=CARTESIAN_POINT ( 'NONE',  ( 6.559798056295000457, 1516.987478262539980, 213.7368632980669929 ) ) ;
#18774=CARTESIAN_POINT ( 'NONE',  ( 2.966689972984999812, 1511.639769324940062, 216.8150789852670073 ) ) ;
#18775=B_SPLINE_CURVE_WITH_KNOTS ( 'NONE', 5,
 ( #90832, #39335, #87685, #62508, #96066, #73508 ),
 .UNSPECIFIED., .F., .F.,
 ( 6, 6 ),
 ( 0.000000000000000000, 1.000000000000000000 ),
 .UNSPECIFIED. ) ;
#18780=CARTESIAN_POINT ( 'NONE',  ( -1.711311266675000109, 1516.591755933730155, 203.3510257909670145 ) ) ;
#18783=CARTESIAN_POINT ( 'NONE',  ( -5.551188713984379852, 1510.480349263560129, 201.5713426139130320 ) ) ;
#18792=CARTESIAN_POINT ( 'NONE',  ( -1.906499846882070084E-08, 1517.051704408389924, 209.1218459511669892 ) ) ;
#18797=CARTESIAN_POINT ( 'NONE',  ( 3.267603515704999850, 1516.858171774179937, 212.3749871074670068 ) ) ;
#18803=CARTESIAN_POINT ( 'NONE',  ( -4.623892098755000291, 1517.066898074209803, 208.3852847535989952 ) ) ;
#18805=ORIENTED_EDGE ( 'NONE', *, *, #48148, .T. ) ;
#18819=CARTESIAN_POINT ( 'NONE',  ( -2.482067898354999969, 1517.099836525840146, 214.9099431973869798 ) ) ;
#18822=CARTESIAN_POINT ( 'NONE',  ( -5.778999811904999895, 1516.955859323880077, 216.4549161051170074 ) ) ;
#18824=CARTESIAN_POINT ( 'NONE',  ( 2.291514297774999598, 1517.194972660189933, 201.3955140066269962 ) ) ;
#18829=CARTESIAN_POINT ( 'NONE',  ( 8.467409380977830580, 1511.685461860059831, 203.1348221448780009 ) ) ;
#18837=CARTESIAN_POINT ( 'NONE',  ( 6.391938627041045429, 1508.551704408389924, 216.1347676210409077 ) ) ;
#18840=CARTESIAN_POINT ( 'NONE',  ( 5.513435558552499671, 1509.038615934029849, 201.6090957240569992 ) ) ;
#18855=CARTESIAN_POINT ( 'NONE',  ( -2.409189714827860040, 1516.533014244449987, 201.4128479977840129 ) ) ;
#18857=EDGE_LOOP ( 'NONE', ( #39733, #12445, #28894, #12750 ) ) ;
#18887=ADVANCED_FACE ( 'NONE', ( #66658 ), #110280, .F. ) ;
#18901=CARTESIAN_POINT ( 'NONE',  ( -2.284053509485000077, 1516.854133554269993, 210.2586600040969813 ) ) ;
#18902=CARTESIAN_POINT ( 'NONE',  ( -7.012921583638330070, 1508.551704408389924, 203.6084103760139783 ) ) ;
#18916=CARTESIAN_POINT ( 'NONE',  ( 3.253301381255000013, 1516.790374942449944, 207.9863856151469861 ) ) ;
#18926=EDGE_CURVE ( 'NONE', #52986, #40123, #57707, .T. ) ;
#18934=CARTESIAN_POINT ( 'NONE',  ( -2.492443689034999910, 1516.793978928989873, 205.8699571027569846 ) ) ;
#18936=VERTEX_POINT ( 'NONE', #16199 ) ;
#18954=CARTESIAN_POINT ( 'NONE',  ( 2.295485501044999932, 1516.651306816259876, 214.1175719399469983 ) ) ;
#18957=DIRECTION ( 'NONE',  ( 0.01484500364209119690, 0.5669078173028199163, -0.8236474686100957454 ) ) ;
#18980=CARTESIAN_POINT ( 'NONE',  ( -4.997573825325000385, 1516.742629295279812, 212.5803724681170195 ) ) ;
#18984=ORIENTED_EDGE ( 'NONE', *, *, #72053, .F. ) ;
#19020=B_SPLINE_CURVE_WITH_KNOTS ( 'NONE', 3,
 ( #82819, #7227, #5011, #22889, #64944, #15588 ),
 .UNSPECIFIED., .F., .F.,
 ( 4, 2, 4 ),
 ( 1.358608016385320016E-06, 0.01184128846600049877, 0.02355710845665270198 ),
 .UNSPECIFIED. ) ;
#19022=CARTESIAN_POINT ( 'NONE',  ( -2.881548462575000080, 1516.909589401870107, 206.8382752989369919 ) ) ;
#19036=CARTESIAN_POINT ( 'NONE',  ( -0.7353365779029981120, 1516.995911393979895, 212.0011643880069698 ) ) ;
#19052=ORIENTED_EDGE ( 'NONE', *, *, #26725, .T. ) ;
#19062=CARTESIAN_POINT ( 'NONE',  ( 7.328049280255000575, 1516.809497469189864, 202.5664528150769854 ) ) ;
#19063=CARTESIAN_POINT ( 'NONE',  ( 2.299667965875000331, 1516.965971551240045, 210.2399506998270056 ) ) ;
#19085=CARTESIAN_POINT ( 'NONE',  ( -8.038901823954999415, 1514.330398624140116, 202.2117929003169934 ) ) ;
#19086=ORIENTED_EDGE ( 'NONE', *, *, #3822, .F. ) ;
#19102=CARTESIAN_POINT ( 'NONE',  ( 8.788316489185000080, 1511.741868877540128, 202.8695794779170001 ) ) ;
#19107=CARTESIAN_POINT ( 'NONE',  ( 4.995994787574999485, 1516.665179208830068, 206.6322283937570035 ) ) ;
#19126=CARTESIAN_POINT ( 'NONE',  ( -2.234922686965000516, 1512.341036949130057, 201.5226187864570022 ) ) ;
#19157=CARTESIAN_POINT ( 'NONE',  ( -6.947377821305000367, 1517.009964551830080, 204.5062011277169916 ) ) ;
#19179=CARTESIAN_POINT ( 'NONE',  ( 5.786837678925000006, 1517.040132827679827, 212.3790665729270017 ) ) ;
#19189=CARTESIAN_POINT ( 'NONE',  ( -8.371228039894999640, 1512.069761553110084, 215.5056669251370067 ) ) ;
#19192=AXIS2_PLACEMENT_3D ( 'NONE', #5633, #106435, #55497 ) ;
#19201=CARTESIAN_POINT ( 'NONE',  ( 4.995725969715000048, 1516.651306816259876, 206.8263604310569690 ) ) ;
#19212=FACE_OUTER_BOUND ( 'NONE', #1337, .T. ) ;
#19219=CARTESIAN_POINT ( 'NONE',  ( -1.121950782074999875, 1517.123342927159911, 214.1352753262870010 ) ) ;
#19223=CARTESIAN_POINT ( 'NONE',  ( -4.027697264044999947, 1516.766397346390022, 212.0005392193770035 ) ) ;
#19240=CARTESIAN_POINT ( 'NONE',  ( -2.489617576474999705, 1516.665179208830068, 204.1258511445269903 ) ) ;
#19250=EDGE_CURVE ( 'NONE', #12028, #29708, #22255, .T. ) ;
#19273=CYLINDRICAL_SURFACE ( 'NONE', #68066, 0.9999999999999988898 ) ;
#19278=B_SPLINE_CURVE_WITH_KNOTS ( 'NONE', 3,
 ( #44740, #27918, #17824, #36310, #77771, #69395 ),
 .UNSPECIFIED., .F., .F.,
 ( 4, 2, 4 ),
 ( 0.000000000000000000, 0.5000000000000000000, 1.000000000000000000 ),
 .UNSPECIFIED. ) ;
#19285=CARTESIAN_POINT ( 'NONE',  ( -3.229842622735000113, 1517.051704408389924, 217.4817367409870030 ) ) ;
#19306=CARTESIAN_POINT ( 'NONE',  ( -7.567811406605000180, 1511.141271963170084, 212.1712098993370148 ) ) ;
#19322=ORIENTED_EDGE ( 'NONE', *, *, #80964, .F. ) ;
#19326=CARTESIAN_POINT ( 'NONE',  ( 4.620008207075000151, 1516.777260590120022, 214.8964555921769772 ) ) ;
#19327=CARTESIAN_POINT ( 'NONE',  ( 3.049363929105000093, 1511.141271963160079, 216.6896573387070077 ) ) ;
#19335=CARTESIAN_POINT ( 'NONE',  ( -4.620008245204999753, 1516.777260590120022, 203.3472363101570011 ) ) ;
#19350=CARTESIAN_POINT ( 'NONE',  ( -4.027051443935000030, 1516.733363207009916, 211.6130343286269806 ) ) ;
#19355=CARTESIAN_POINT ( 'NONE',  ( 2.879318417774999972, 1516.995911393979895, 209.8571825100049750 ) ) ;
#19370=CARTESIAN_POINT ( 'NONE',  ( 5.006329581384999727, 1516.755758396839838, 215.6722354023569892 ) ) ;
#19381=CARTESIAN_POINT ( 'NONE',  ( 7.533847528226220724, 1510.598356033829987, 203.2091179615540284 ) ) ;
#19387=ADVANCED_FACE ( 'NONE', ( #26127 ), #53587, .F. ) ;
#19414=DIRECTION ( 'NONE',  ( 0.7071067811865475727, -6.078560574715863648E-17, 0.7071067811865475727 ) ) ;
#19415=CARTESIAN_POINT ( 'NONE',  ( -1.579129830164079928, 1516.559523801380010, 201.4121538206049706 ) ) ;
#19462=CARTESIAN_POINT ( 'NONE',  ( -3.447128498755000159, 1516.778853242349896, 210.2570310142770040 ) ) ;
#19464=DIRECTION ( 'NONE',  ( -0.7071067811865475727, 0.000000000000000000, 0.7071067811865475727 ) ) ;
#19468=B_SPLINE_SURFACE_WITH_KNOTS ( 'NONE', 5, 5, ( 
 ( #54072, #88198, #95486, #27730, #46213, #45112 ),
 ( #80347, #53508, #62477, #105554, #63037, #54617 ),
 ( #2004, #79806, #96597, #79253, #45667, #2562 ),
 ( #38325, #106094, #3111, #10369, #3664, #72504 ),
 ( #46765, #37240, #61918, #37793, #36685, #55165 ),
 ( #71981, #97142, #29372, #97688, #18753, #96035 ),
 ( #52950, #70879, #20961, #89288, #19306, #80895 ),
 ( #106633, #13652, #21503, #92046, #22048, #64113 ),
 ( #82553, #15318, #56245, #5847, #49512, #38871 ),
 ( #23173, #65757, #40537, #98786, #47292, #73614 ),
 ( #100444, #74164, #22596, #83636, #56799, #98234 ),
 ( #90936, #39987, #31580, #48965, #57373, #65209 ) ),
 .UNSPECIFIED., .F., .F., .F.,
 ( 6, 3, 3, 6 ),
 ( 6, 6 ),
 ( 3.672001930560000016, 6.062162762939999894, 7.801458206509999549, 8.912489289850000773 ),
 ( 0.000000000000000000, 1.000000000000000000 ),
 .UNSPECIFIED. ) ;
#19477=ORIENTED_EDGE ( 'NONE', *, *, #54848, .T. ) ;
#19479=CARTESIAN_POINT ( 'NONE',  ( -7.726684725664999753, 1517.208444099459939, 207.9957078235169945 ) ) ;
#19496=LINE ( 'NONE', #53129, #671 ) ;
#19497=CARTESIAN_POINT ( 'NONE',  ( -3.268235758764999943, 1516.890356958860139, 206.2562572478169898 ) ) ;
#19506=CARTESIAN_POINT ( 'NONE',  ( 7.592573332174999301, 1517.051705360460119, 213.6085791126270124 ) ) ;
#19515=CARTESIAN_POINT ( 'NONE',  ( -1.705466448594999962, 1517.120861839400050, 214.1360410720469929 ) ) ;
#19517=ORIENTED_EDGE ( 'NONE', *, *, #77071, .T. ) ;
#19585=CARTESIAN_POINT ( 'NONE',  ( -6.039224196466708605, 1516.749004811059876, 213.5695341108769583 ) ) ;
#19589=CARTESIAN_POINT ( 'NONE',  ( -7.338753868364999988, 1517.184383877180153, 206.8309596656170015 ) ) ;
#19602=CARTESIAN_POINT ( 'NONE',  ( -2.282915221395000138, 1516.876240617270014, 211.6158662526670184 ) ) ;
#19612=CARTESIAN_POINT ( 'NONE',  ( 13.20762147703265654, 1513.543684532346106, 225.9078262356120774 ) ) ;
#19613=B_SPLINE_CURVE_WITH_KNOTS ( 'NONE', 5,
 ( #22959, #90731, #108081, #31376, #65558, #54959, #91289, #89087, #48760 ),
 .UNSPECIFIED., .F., .F.,
 ( 6, 3, 6 ),
 ( 0.000000000000000000, 0.5000000000000000000, 1.000000000000000000 ),
 .UNSPECIFIED. ) ;
#19616=EDGE_LOOP ( 'NONE', ( #51925, #38891, #10932, #19517, #25132 ) ) ;
#19624=CARTESIAN_POINT ( 'NONE',  ( 6.766140024152450749, 1508.878901399440110, 201.8613017694559915 ) ) ;
#19630=CARTESIAN_POINT ( 'NONE',  ( -3.455378015385000001, 1516.627618683580067, 202.1863880069169852 ) ) ;
#19631=CARTESIAN_POINT ( 'NONE',  ( -1.119592219845000125, 1516.958737650239982, 210.2577447559170025 ) ) ;
#19652=CARTESIAN_POINT ( 'NONE',  ( -7.570419153255000033, 1513.830194289050041, 202.8006730981169596 ) ) ;
#19667=CARTESIAN_POINT ( 'NONE',  ( 11.95959062223499991, 1513.007288725360013, 225.7330057136669836 ) ) ;
#19676=CARTESIAN_POINT ( 'NONE',  ( -1.717084749545000122, 1516.819260244609950, 206.6456753351970121 ) ) ;
#19697=CARTESIAN_POINT ( 'NONE',  ( -2.566007203944999926, 1512.021995456199875, 201.5004268114669799 ) ) ;
#19700=CARTESIAN_POINT ( 'NONE',  ( 17.17760792425680094, 1517.051704368240053, 222.7507317666290305 ) ) ;
#19733=CARTESIAN_POINT ( 'NONE',  ( 5.774609621945000271, 1516.777260590120022, 204.5018377250270021 ) ) ;
#19743=VERTEX_POINT ( 'NONE', #34225 ) ;
#19753=CARTESIAN_POINT ( 'NONE',  ( -6.547556969464999987, 1516.633288330999903, 212.3841106205370011 ) ) ;
#19763=CARTESIAN_POINT ( 'NONE',  ( -8.232567760474999830, 1512.371207877109782, 215.7807634015769906 ) ) ;
#19774=CARTESIAN_POINT ( 'NONE',  ( 6.933587655514999781, 1516.542957540330008, 207.4124872689769745 ) ) ;
#19792=CARTESIAN_POINT ( 'NONE',  ( -4.033653302454999867, 1517.028034847769959, 215.6825881955670070 ) ) ;
#19794=CARTESIAN_POINT ( 'NONE',  ( 5.619917992193439460, 1511.009256124219974, 216.8017735542370019 ) ) ;
#19796=CARTESIAN_POINT ( 'NONE',  ( 0.7574259850960020080, 1516.837969789639828, 212.3776558342370038 ) ) ;
#19797=CARTESIAN_POINT ( 'NONE',  ( 4.329791512777563689, 1515.051704408389924, 213.0376480771570868 ) ) ;
#19812=CARTESIAN_POINT ( 'NONE',  ( 6.549762446985000430, 1516.729202374750002, 204.5030968636170030 ) ) ;
#19837=B_SPLINE_CURVE_WITH_KNOTS ( 'NONE', 5,
 ( #49473, #64080, #14744, #31545, #81945, #23135, #14187, #55681, #48374 ),
 .UNSPECIFIED., .F., .F.,
 ( 6, 3, 6 ),
 ( 0.8631820001114760554, 2.053866005420000196, 3.194080077832680331 ),
 .UNSPECIFIED. ) ;
#19851=CARTESIAN_POINT ( 'NONE',  ( -14.69977925956500009, 1513.518111364920060, 193.4636334463669982 ) ) ;
#19855=CARTESIAN_POINT ( 'NONE',  ( 6.554151426245000245, 1516.906641539930206, 201.7900338461269882 ) ) ;
#19859=CARTESIAN_POINT ( 'NONE',  ( 7.686100004535000529, 1512.192993275409890, 206.4318633740769826 ) ) ;
#19885=CARTESIAN_POINT ( 'NONE',  ( 0.7560907277860019482, 1516.770163853809890, 214.1221759657669850 ) ) ;
#19886=CARTESIAN_POINT ( 'NONE',  ( 4.538868744795000687, 1511.336728379370243, 217.2220504028269943 ) ) ;
#19887=MECHANICAL_DESIGN_GEOMETRIC_PRESENTATION_REPRESENTATION('',(#10959),#82490);
#19892=EDGE_CURVE ( 'NONE', #49664, #42497, #92517, .T. ) ;
#19895=CARTESIAN_POINT ( 'NONE',  ( 7.324914918154999732, 1516.685667699390024, 204.5043554653269950 ) ) ;
#19910=CARTESIAN_POINT ( 'NONE',  ( 3.267291605165000057, 1516.842852731759876, 212.5687880419470162 ) ) ;
#19915=CARTESIAN_POINT ( 'NONE',  ( -2.868112169295000236, 1516.855632454399938, 209.8795095036720113 ) ) ;
#19916=VERTEX_POINT ( 'NONE', #98322 ) ;
#19930=ADVANCED_FACE ( 'NONE', ( #4811 ), #99411, .F. ) ;
#19933=CARTESIAN_POINT ( 'NONE',  ( -6.551643424905000401, 1516.807958722750072, 214.9033365145770063 ) ) ;
#19938=CARTESIAN_POINT ( 'NONE',  ( 4.616899834755000320, 1517.050041317280147, 201.3993091674070115 ) ) ;
#19958=VERTEX_POINT ( 'NONE', #3202 ) ;
#20019=CARTESIAN_POINT ( 'NONE',  ( 3.267039691854999983, 1517.012231669750008, 209.8574146130079896 ) ) ;
#20020=CARTESIAN_POINT ( 'NONE',  ( -7.141639615954698428, 1508.551704408398564, 203.6084103740969624 ) ) ;
#20029=CARTESIAN_POINT ( 'NONE',  ( -2.485217232065000115, 1516.534320418310244, 201.4128137944169907 ) ) ;
#20034=CARTESIAN_POINT ( 'NONE',  ( 1.119592181715000079, 1516.958737650239982, 207.9859471464170326 ) ) ;
#20052=CARTESIAN_POINT ( 'NONE',  ( 4.608146781254999880, 1516.677239312369920, 206.8257210811669893 ) ) ;
#20069=CARTESIAN_POINT ( 'NONE',  ( 5.782749401605000727, 1516.858301627840092, 214.8983370654769942 ) ) ;
#20073=LINE ( 'NONE', #97334, #79546 ) ;
#20086=DIRECTION ( 'NONE',  ( 0.000000000000000000, 1.000000000000000000, -6.123233995736769734E-17 ) ) ;
#20112=VERTEX_POINT ( 'NONE', #97223 ) ;
#20140=CARTESIAN_POINT ( 'NONE',  ( 7.708770007014999592, 1516.524310051880093, 206.8307984429870032 ) ) ;
#20144=DIRECTION ( 'NONE',  ( -1.577721810442025012E-32, -1.000000000000000000, 6.123233995736769734E-17 ) ) ;
#20146=ORIENTED_EDGE ( 'NONE', *, *, #37375, .T. ) ;
#20157=ORIENTED_EDGE ( 'NONE', *, *, #11192, .T. ) ;
#20178=CARTESIAN_POINT ( 'NONE',  ( 3.255340926295000159, 1516.962555622980062, 204.4977466407669908 ) ) ;
#20200=CARTESIAN_POINT ( 'NONE',  ( -6.772137629935000014, 1511.702066573619959, 201.9100861211470033 ) ) ;
#20215=CARTESIAN_POINT ( 'NONE',  ( 14.20095105293500026, 1513.466724478469814, 225.6507215884670075 ) ) ;
#20223=CARTESIAN_POINT ( 'NONE',  ( -0.01319654689839849966, 1516.941178807709775, 206.8296289214069930 ) ) ;
#20275=CARTESIAN_POINT ( 'NONE',  ( -3.458526536014999930, 1516.742629295279812, 204.1242721449069961 ) ) ;
#20278=LINE ( 'NONE', #12438, #13674 ) ;
#20297=CARTESIAN_POINT ( 'NONE',  ( 3.267291605165000057, 1516.842852731759876, 212.5687880419470162 ) ) ;
#20307=CARTESIAN_POINT ( 'NONE',  ( -7.641097616105000156, 1512.520476835140016, 215.8818590920970166 ) ) ;
#20310=CARTESIAN_POINT ( 'NONE',  ( -7.012921583605000286, 1508.551704408389924, 214.6352815282469919 ) ) ;
#20318=CARTESIAN_POINT ( 'NONE',  ( 3.445407533985000104, 1516.764084769670262, 206.8237970085970119 ) ) ;
#20323=CARTESIAN_POINT ( 'NONE',  ( -6.725660328943730448, 1508.728103662679814, 201.9181051944200078 ) ) ;
#20329=CARTESIAN_POINT ( 'NONE',  ( 14.76103602627950018, 1512.125809830880144, 196.8968599408240152 ) ) ;
#20331=CARTESIAN_POINT ( 'NONE',  ( -6.161099280462069672, 1511.774605969369986, 200.4817672165819999 ) ) ;
#20337=CARTESIAN_POINT ( 'NONE',  ( -7.716252091104999877, 1516.810037859429940, 216.0641906620670056 ) ) ;
#20341=CARTESIAN_POINT ( 'NONE',  ( -2.865588722415000067, 1516.890356958860139, 212.3900816908670208 ) ) ;
#20358=CARTESIAN_POINT ( 'NONE',  ( 4.610938211375000151, 1516.815231249920089, 205.0813186281270077 ) ) ;
#20389=CARTESIAN_POINT ( 'NONE',  ( -13.07344736774610183, 1516.551188146160030, 225.7923144865690119 ) ) ;
#20395=CARTESIAN_POINT ( 'NONE',  ( -14.21596113916499959, 1513.125294087170005, 193.6610111176670159 ) ) ;
#20402=CARTESIAN_POINT ( 'NONE',  ( 7.693233015035000122, 1511.639769324940062, 206.1551559591169962 ) ) ;
#20422=DIRECTION ( 'NONE',  ( 0.4770263929453589236, -0.7067418228232984490, 0.5224574779883445208 ) ) ;
#20430=CARTESIAN_POINT ( 'NONE',  ( -4.031142389804999837, 1516.929569650079884, 214.1322689334670031 ) ) ;
#20431=CARTESIAN_POINT ( 'NONE',  ( 3.173602151875000388, 1510.830536680500245, 216.6815192743169973 ) ) ;
#20437=CARTESIAN_POINT ( 'NONE',  ( -2.491188396525000126, 1516.733363207009916, 205.0947945262969938 ) ) ;
#20450=CARTESIAN_POINT ( 'NONE',  ( -2.865588722415000067, 1516.890356958860139, 212.3900816908670208 ) ) ;
#20452=VECTOR ( 'NONE', #71560, 1000.000000000000000 ) ;
#20456=CARTESIAN_POINT ( 'NONE',  ( 0.7468175155120010400, 1517.006509894990131, 209.1147170949500094 ) ) ;
#20457=ORIENTED_EDGE ( 'NONE', *, *, #2359, .F. ) ;
#20460=CARTESIAN_POINT ( 'NONE',  ( -5.513435773845334786, 1508.731359864534170, 201.6768079085695433 ) ) ;
#20468=CARTESIAN_POINT ( 'NONE',  ( 2.292940169014999974, 1516.565291103010168, 215.6678853655270132 ) ) ;
#20475=CARTESIAN_POINT ( 'NONE',  ( -15.85140264816500100, 1511.863761374039996, 220.8632120430669943 ) ) ;
#20487=CARTESIAN_POINT ( 'NONE',  ( 13.40786183173499779, 1517.051704408389924, 218.6219621693470003 ) ) ;
#20503=CARTESIAN_POINT ( 'NONE',  ( -3.958649448056769327, 1508.551704408389924, 214.1089243834869933 ) ) ;
#20509=CARTESIAN_POINT ( 'NONE',  ( -0.6353530967299270138, 1516.751726750550233, 201.4071208092509835 ) ) ;
#20514=CARTESIAN_POINT ( 'NONE',  ( 12.97811970330590192, 1512.378201925209851, 224.3338094387339936 ) ) ;
#20517=EDGE_CURVE ( 'NONE', #10258, #58764, #80027, .T. ) ;
#20554=CARTESIAN_POINT ( 'NONE',  ( -2.476450702264999748, 1516.843453247299749, 211.4215022863270121 ) ) ;
#20559=DIRECTION ( 'NONE',  ( 0.000000000000000000, -1.000000000000000000, 6.123233995736769734E-17 ) ) ;
#20561=DIRECTION ( 'NONE',  ( -8.673617379884002932E-16, 0.02617694830786544691, -0.9996573249755575929 ) ) ;
#20562=VECTOR ( 'NONE', #22221, 1000.000000000000000 ) ;
#20563=CARTESIAN_POINT ( 'NONE',  ( 4.035536225084999984, 1517.086065052259983, 201.3983658527070020 ) ) ;
#20585=CARTESIAN_POINT ( 'NONE',  ( -0.7578858299649979813, 1516.872851364150165, 206.6414186775969881 ) ) ;
#20602=CARTESIAN_POINT ( 'NONE',  ( 0.7553264358530019651, 1516.745833913490060, 214.8974710475970085 ) ) ;
#20645=ORIENTED_EDGE ( 'NONE', *, *, #40285, .F. ) ;
#20663=CARTESIAN_POINT ( 'NONE',  ( -7.166260544089549711, 1508.551565390810083, 215.1547104977369997 ) ) ;
#20668=CYLINDRICAL_SURFACE ( 'NONE', #14119, 1.000000000000076383 ) ;
#20677=CARTESIAN_POINT ( 'NONE',  ( 6.933587655514999781, 1516.542957540330008, 207.4124872689769745 ) ) ;
#20699=CARTESIAN_POINT ( 'NONE',  ( 12.05347594647225939, 1513.055456493726751, 225.7288246710316173 ) ) ;
#20719=CARTESIAN_POINT ( 'NONE',  ( 4.999456390405000228, 1516.830644417779922, 204.5005780481670001 ) ) ;
#20722=CARTESIAN_POINT ( 'NONE',  ( 5.441672279850854110, 1511.126521620429685, 216.8250749836011835 ) ) ;
#20728=( BOUNDED_CURVE ( )  B_SPLINE_CURVE ( 3, ( #2829, #87934, #11223, #80619 ),
 .UNSPECIFIED., .F., .T. ) 
 B_SPLINE_CURVE_WITH_KNOTS ( ( 4, 4 ),
 ( 4.712545041747917551, 6.283338160402144545 ),
 .UNSPECIFIED. ) 
 CURVE ( )  GEOMETRIC_REPRESENTATION_ITEM ( )  RATIONAL_B_SPLINE_CURVE ( ( 1.000000000000000000, 0.8047386102897660098, 0.8047386102897660098, 1.000000000000000000 ) ) 
 REPRESENTATION_ITEM ( '' )  );
#20741=CARTESIAN_POINT ( 'NONE',  ( -6.564976431375000310, 1512.035910181030204, 201.6179728287370096 ) ) ;
#20758=EDGE_CURVE ( 'NONE', #97290, #89473, #78808, .T. ) ;
#20764=CARTESIAN_POINT ( 'NONE',  ( 3.251611325815000342, 1516.779243033999819, 206.8234764622770001 ) ) ;
#20805=ORIENTED_EDGE ( 'NONE', *, *, #110602, .T. ) ;
#20825=CARTESIAN_POINT ( 'NONE',  ( 2.867803626105000170, 1516.994127245590107, 204.4971090729170271 ) ) ;
#20832=ORIENTED_EDGE ( 'NONE', *, *, #108567, .T. ) ;
#20833=ORIENTED_EDGE ( 'NONE', *, *, #83756, .F. ) ;
#20845=CARTESIAN_POINT ( 'NONE',  ( -1.702406023195000007, 1516.999105586269934, 212.3918307515370145 ) ) ;
#20855=CARTESIAN_POINT ( 'NONE',  ( -6.787530816394999889, 1514.254015528269974, 216.9772499547270002 ) ) ;
#20868=CARTESIAN_POINT ( 'NONE',  ( 2.476170596904999854, 1516.819260244609950, 207.4047612206870213 ) ) ;
#20872=ORIENTED_EDGE ( 'NONE', *, *, #100073, .F. ) ;
#20885=CARTESIAN_POINT ( 'NONE',  ( -3.452917061035000401, 1517.089216728169959, 216.0711116162470091 ) ) ;
#20887=CARTESIAN_POINT ( 'NONE',  ( 6.014475185372909927, 1511.645396655840159, 217.0724277449770057 ) ) ;
#20889=CARTESIAN_POINT ( 'NONE',  ( 4.043366220174999803, 1516.951766529250108, 211.9887038632370206 ) ) ;
#20902=VECTOR ( 'NONE', #85070, 1000.000000000000000 ) ;
#20905=VERTEX_POINT ( 'NONE', #83202 ) ;
#20906=CARTESIAN_POINT ( 'NONE',  ( -0.7568987378019988999, 1516.805675336850072, 205.0906771642370074 ) ) ;
#20910=CARTESIAN_POINT ( 'NONE',  ( -7.627639037761098528, 1513.425324099843010, 202.6766267095247258 ) ) ;
#20913=CARTESIAN_POINT ( 'NONE',  ( 3.424720300894999792, 1517.051704408389924, 200.5840233334270124 ) ) ;
#20926=CARTESIAN_POINT ( 'NONE',  ( -12.03841672722804290, 1513.050507398017544, 192.5203960790572069 ) ) ;
#20933=CARTESIAN_POINT ( 'NONE',  ( 7.891777514710270225, 1512.314860025949883, 206.1798159824890035 ) ) ;
#20943=CARTESIAN_POINT ( 'NONE',  ( -11.74940792826499880, 1512.456207068040158, 192.6559229132670055 ) ) ;
#20946=CARTESIAN_POINT ( 'NONE',  ( -1.708092304294999808, 1516.523379810429788, 201.4131002843170108 ) ) ;
#20950=CARTESIAN_POINT ( 'NONE',  ( 15.52404075913500137, 1511.843510977570077, 197.7123968315669913 ) ) ;
#20961=CARTESIAN_POINT ( 'NONE',  ( -7.717016657154999848, 1511.440441732939917, 212.3987529968069907 ) ) ;
#20967=PRESENTATION_STYLE_ASSIGNMENT (( #78696 ) ) ;
#20972=DIRECTION ( 'NONE',  ( 0.9996573249755574819, 0.02617694830786558916, 0.000000000000000000 ) ) ;
#20973=ORIENTED_EDGE ( 'NONE', *, *, #89633, .T. ) ;
#20981=CARTESIAN_POINT ( 'NONE',  ( 7.333070134885000257, 1516.955859323880077, 214.9008457440070003 ) ) ;
#20988=CARTESIAN_POINT ( 'NONE',  ( -5.010423001364999962, 1516.929569650079884, 205.0907035804270038 ) ) ;
#20990=DIRECTION ( 'NONE',  ( 0.02616798426500960631, 0.9993150019883683122, 0.02616798426500960631 ) ) ;
#21000=CARTESIAN_POINT ( 'NONE',  ( 6.948321705865000197, 1517.049325831759916, 213.1561268858870051 ) ) ;
#21006=CARTESIAN_POINT ( 'NONE',  ( -7.708848719128969407, 1516.527314490149820, 211.2746510465439940 ) ) ;
#21007=CARTESIAN_POINT ( 'NONE',  ( -7.326072182274999456, 1516.714320817460020, 209.8751461055349807 ) ) ;
#21019=CARTESIAN_POINT ( 'NONE',  ( 4.617490466775000080, 1516.685667699390024, 216.4467608883869900 ) ) ;
#21023=VECTOR ( 'NONE', #46255, 1000.000000000000000 ) ;
#21025=CARTESIAN_POINT ( 'NONE',  ( -2.872700555325000238, 1516.559109716219837, 201.4121646638069763 ) ) ;
#21028=CARTESIAN_POINT ( 'NONE',  ( -15.90990259576500065, 1512.830284628050094, 220.0820010595669771 ) ) ;
#21042=VERTEX_POINT ( 'NONE', #20389 ) ;
#21053=CARTESIAN_POINT ( 'NONE',  ( -7.315867787722543092, 1516.555258207057705, 210.7873785203714760 ) ) ;
#21063=CARTESIAN_POINT ( 'NONE',  ( 12.37943797690240189, 1512.150422497869840, 224.0155786243819875 ) ) ;
#21104=CARTESIAN_POINT ( 'NONE',  ( -2.864043456445000135, 1516.811292230880099, 211.4208600009669965 ) ) ;
#21111=CARTESIAN_POINT ( 'NONE',  ( 6.941727252324999320, 1516.882217593000178, 201.7906628411569727 ) ) ;
#21130=CARTESIAN_POINT ( 'NONE',  ( 1.701729820345000199, 1516.969638403840008, 206.2395199527169893 ) ) ;
#21146=CARTESIAN_POINT ( 'NONE',  ( -0.7376675409259989546, 1517.104497701820037, 214.9086937099069985 ) ) ;
#21148=CARTESIAN_POINT ( 'NONE',  ( 7.708852660943830593, 1516.527466478090219, 206.9210818302649955 ) ) ;
#21213=CARTESIAN_POINT ( 'NONE',  ( 6.548200587644999793, 1516.632821972880038, 207.9912384682270101 ) ) ;
#21215=VECTOR ( 'NONE', #28420, 1000.000000000000000 ) ;
#21235=CARTESIAN_POINT ( 'NONE',  ( 13.95549232207893553, 1513.969110081093959, 225.7819657676807594 ) ) ;
#21252=CARTESIAN_POINT ( 'NONE',  ( -5.782749439735000330, 1516.858301627840092, 203.3453548368569841 ) ) ;
#21257=EDGE_LOOP ( 'NONE', ( #93173, #2329, #65321, #38487, #94984, #66478, #14920, #7957 ) ) ;
#21278=CARTESIAN_POINT ( 'NONE',  ( -6.527830581335000382, 1512.220794350740107, 201.3447709183070060 ) ) ;
#21290=CYLINDRICAL_SURFACE ( 'NONE', #19192, 0.9999999999999569233 ) ;
#21291=AXIS2_PLACEMENT_3D ( 'NONE', #54, #605, #34735 ) ;
#21294=CARTESIAN_POINT ( 'NONE',  ( 15.37680647863500205, 1514.414736986979960, 224.4895214034669948 ) ) ;
#21302=CARTESIAN_POINT ( 'NONE',  ( -0.7579263249019989601, 1516.927039499179955, 207.4176752179770347 ) ) ;
#21360=CARTESIAN_POINT ( 'NONE',  ( 3.448206878685000198, 1516.904492006980036, 205.0794281543969646 ) ) ;
#21366=ORIENTED_EDGE ( 'NONE', *, *, #77, .F. ) ;
#21374=CARTESIAN_POINT ( 'NONE',  ( -4.028611259245000298, 1516.744381837270112, 210.2562039408269925 ) ) ;
#21389=VERTEX_POINT ( 'NONE', #96728 ) ;
#21390=ORIENTED_EDGE ( 'NONE', *, *, #105003, .F. ) ;
#21391=CARTESIAN_POINT ( 'NONE',  ( -6.017564101925000131, 1514.771170611759999, 217.0138083832570146 ) ) ;
#21392=CARTESIAN_POINT ( 'NONE',  ( 16.44706023844862841, 1514.320576807016550, 194.6473512539881199 ) ) ;
#21404=CARTESIAN_POINT ( 'NONE',  ( -1.136814071995000175, 1516.854133554269993, 206.8377924607469822 ) ) ;
#21415=CARTESIAN_POINT ( 'NONE',  ( -5.704331135097779892, 1511.494703458840149, 200.8748168550339983 ) ) ;
#21417=CARTESIAN_POINT ( 'NONE',  ( -5.567211192487503624, 1510.484595312941110, 201.5712314627286617 ) ) ;
#21423=CARTESIAN_POINT ( 'NONE',  ( 2.487103419534999915, 1516.577434278289957, 215.6681487122470173 ) ) ;
#21428=CARTESIAN_POINT ( 'NONE',  ( 7.723480079395000253, 1517.086065052259983, 213.1573821953169841 ) ) ;
#21445=CARTESIAN_POINT ( 'NONE',  ( -2.297085753945000253, 1516.718889242609976, 205.0950684461469962 ) ) ;
#21447=EDGE_CURVE ( 'NONE', #30006, #84966, #87215, .T. ) ;
#21474=CARTESIAN_POINT ( 'NONE',  ( 8.053223258311438926, 1511.610050756687770, 205.5741034559911782 ) ) ;
#21483=CARTESIAN_POINT ( 'NONE',  ( -12.84824846446499969, 1512.167884426309911, 193.7405250718670118 ) ) ;
#21488=CARTESIAN_POINT ( 'NONE',  ( -2.873958889724999910, 1516.588006113850042, 202.1873174023370154 ) ) ;
#21500=CARTESIAN_POINT ( 'NONE',  ( -3.043932075285961769, 1516.569307157451021, 201.4118976829438736 ) ) ;
#21503=CARTESIAN_POINT ( 'NONE',  ( -7.693233053164999724, 1511.639769324940062, 212.0885359432170389 ) ) ;
#21525=CARTESIAN_POINT ( 'NONE',  ( 2.488360629304999794, 1516.616791731099966, 214.8929950451170043 ) ) ;
#21532=CARTESIAN_POINT ( 'NONE',  ( 2.285487581364999965, 1517.001127920769704, 205.0775242521070254 ) ) ;
#21539=CARTESIAN_POINT ( 'NONE',  ( 6.277682552355000389, 1511.927085655879864, 217.0033795624569848 ) ) ;
#21550=CARTESIAN_POINT ( 'NONE',  ( -2.865911554774999814, 1516.906233342200039, 212.5838411289170153 ) ) ;
#21557=CARTESIAN_POINT ( 'NONE',  ( -7.716338871780399344, 1516.813354641049955, 209.5384311660010042 ) ) ;
#21559=CARTESIAN_POINT ( 'NONE',  ( -3.449647478144999724, 1516.829948096479939, 209.8791439064560223 ) ) ;
#21573=CARTESIAN_POINT ( 'NONE',  ( 7.330554133425000174, 1516.857992118400034, 216.4511490482170188 ) ) ;
#21578=CARTESIAN_POINT ( 'NONE',  ( 7.329303077985000137, 1516.857992118400034, 201.7912917986770083 ) ) ;
#21610=CARTESIAN_POINT ( 'NONE',  ( -1.906499846882070084E-08, 1516.801704408389924, 209.1218459511669892 ) ) ;
#21611=CARTESIAN_POINT ( 'NONE',  ( 0.4346943641293429805, 1517.051704428850144, 201.3992661435559910 ) ) ;
#21615=CARTESIAN_POINT ( 'NONE',  ( 13.96132452455360173, 1513.058738973300024, 224.4023983419680235 ) ) ;
#21616=VERTEX_POINT ( 'NONE', #83768 ) ;
#21632=AXIS2_PLACEMENT_3D ( 'NONE', #110085, #42890, #42328 ) ;
#21637=ORIENTED_EDGE ( 'NONE', *, *, #108527, .F. ) ;
#21654=CARTESIAN_POINT ( 'NONE',  ( 3.269984781304999810, 1516.999105586269934, 210.8242519552970009 ) ) ;
#21656=CARTESIAN_POINT ( 'NONE',  ( 5.786837678925000006, 1517.040132827679827, 212.3790665729270017 ) ) ;
#21662=CARTESIAN_POINT ( 'NONE',  ( -0.01073133209419849937, 1516.939491476980038, 201.7897819926569980 ) ) ;
#21678=CARTESIAN_POINT ( 'NONE',  ( 0.7579262867720020225, 1516.927039499179955, 210.8260166843570005 ) ) ;
#21684=CARTESIAN_POINT ( 'NONE',  ( 7.618992673874999788, 1511.297452611750032, 205.9539561133169911 ) ) ;
#21685=CARTESIAN_POINT ( 'NONE',  ( -3.462620856235000044, 1516.938330505699923, 206.6435391121569864 ) ) ;
#21688=CARTESIAN_POINT ( 'NONE',  ( -0.9370951672101170971, 1516.671995221562156, 201.6725580799513011 ) ) ;
#21689=ORIENTED_EDGE ( 'NONE', *, *, #72159, .F. ) ;
#21702=CARTESIAN_POINT ( 'NONE',  ( 4.037378256055000669, 1516.688761843659904, 215.6706679112870120 ) ) ;
#21704=CARTESIAN_POINT ( 'NONE',  ( 7.712858129429029930, 1516.680429148250141, 208.2106503431979831 ) ) ;
#21710=DIRECTION ( 'NONE',  ( -0.001619481660810790291, -0.06184550950385309803, 0.9980844203940660853 ) ) ;
#21765=CARTESIAN_POINT ( 'NONE',  ( -8.790528956024720841, 1511.742084109019970, 215.3764313309009992 ) ) ;
#21769=CARTESIAN_POINT ( 'NONE',  ( 7.321169230994999388, 1516.531533746980131, 207.4131249475269954 ) ) ;
#21790=CARTESIAN_POINT ( 'NONE',  ( 12.99084550840746566, 1513.436209034644207, 225.9095066078032801 ) ) ;
#21799=CARTESIAN_POINT ( 'NONE',  ( 4.534010743204659910, 1508.610336716400070, 204.8848650279689991 ) ) ;
#21807=CARTESIAN_POINT ( 'NONE',  ( -4.038637500854999729, 1516.734985836460055, 203.3481771172569950 ) ) ;
#21815=CARTESIAN_POINT ( 'NONE',  ( 4.678155150208202606, 1508.611350403811457, 205.6342600829154321 ) ) ;
#21817=CARTESIAN_POINT ( 'NONE',  ( -13.34643008454949964, 1512.594488815709838, 193.8269363163149990 ) ) ;
#21843=CARTESIAN_POINT ( 'NONE',  ( 13.99234587423499931, 1513.736060322949925, 225.8518394019669984 ) ) ;
#21849=CARTESIAN_POINT ( 'NONE',  ( 0.7350231981660010350, 1516.970035769810011, 206.8242163110469960 ) ) ;
#21887=EDGE_CURVE ( 'NONE', #97701, #55731, #50642, .T. ) ;
#21898=CARTESIAN_POINT ( 'NONE',  ( -3.179706416137069169, 1511.827399571667684, 201.1786234408949952 ) ) ;
#21905=CARTESIAN_POINT ( 'NONE',  ( -0.7572979743539989261, 1516.829948096479939, 205.6721984920870057 ) ) ;
#21919=CARTESIAN_POINT ( 'NONE',  ( 7.339107202615000602, 1517.203017563489766, 210.2473558205170150 ) ) ;
#21931=VERTEX_POINT ( 'NONE', #52398 ) ;
#21932=ORIENTED_EDGE ( 'NONE', *, *, #7006, .F. ) ;
#21935=CARTESIAN_POINT ( 'NONE',  ( 16.25130722332281152, 1514.566425926116381, 194.3271904957884999 ) ) ;
#21939=LINE ( 'NONE', #39329, #35793 ) ;
#21947=CARTESIAN_POINT ( 'NONE',  ( 2.865636809105000182, 1516.815173273089840, 207.9858416580370033 ) ) ;
#21956=B_SPLINE_CURVE_WITH_KNOTS ( 'NONE', 3,
 ( #92740, #102775, #101125, #50216 ),
 .UNSPECIFIED., .F., .F.,
 ( 4, 4 ),
 ( 0.9214954035317776126, 1.000000000000000000 ),
 .UNSPECIFIED. ) ;
#21958=CARTESIAN_POINT ( 'NONE',  ( -6.247704817804169863, 1510.876154134900162, 201.6775610366950104 ) ) ;
#21960=CARTESIAN_POINT ( 'NONE',  ( -5.761500042352934337, 1510.554407334616599, 201.5803765894013111 ) ) ;
#21964=CARTESIAN_POINT ( 'NONE',  ( -7.328676208015000526, 1516.833844030519913, 216.0648195994369871 ) ) ;
#21969=CARTESIAN_POINT ( 'NONE',  ( 2.412842859265553308, 1516.533219998030972, 216.8308492924006998 ) ) ;
#21970=CARTESIAN_POINT ( 'NONE',  ( -1.702754409475000008, 1517.014196759610059, 212.5856132281170119 ) ) ;
#21983=EDGE_CURVE ( 'NONE', #1894, #5115, #5218, .T. ) ;
#21988=CARTESIAN_POINT ( 'NONE',  ( 5.772727908745000747, 1516.691414181030041, 205.6645793267070133 ) ) ;
#22008=CARTESIAN_POINT ( 'NONE',  ( -11.28286893315524964, 1512.859150068915596, 192.9221778144517145 ) ) ;
#22009=EDGE_CURVE ( 'NONE', #17382, #68939, #43861, .T. ) ;
#22016=CARTESIAN_POINT ( 'NONE',  ( 8.150367991650082189, 1511.506734315487620, 205.2632391311709057 ) ) ;
#22024=CARTESIAN_POINT ( 'NONE',  ( -7.469839269216643984, 1510.808998940006859, 215.2720920852931101 ) ) ;
#22028=CARTESIAN_POINT ( 'NONE',  ( -12.38398713116500005, 1512.136030808819896, 194.2018088040669852 ) ) ;
#22031=ADVANCED_FACE ( 'NONE', ( #53797 ), #12850, .F. ) ;
#22032=CARTESIAN_POINT ( 'NONE',  ( -4.036119682645000317, 1516.647924054489977, 201.7978713257969900 ) ) ;
#22045=CARTESIAN_POINT ( 'NONE',  ( -2.759740495412019712, 1516.551695078709827, 201.4123589199890034 ) ) ;
#22048=CARTESIAN_POINT ( 'NONE',  ( -7.575166957224999997, 1511.422242621320265, 211.8233863454470054 ) ) ;
#22068=CARTESIAN_POINT ( 'NONE',  ( 3.261007131564999995, 1516.596789218710001, 216.4445556570670135 ) ) ;
#22077=CARTESIAN_POINT ( 'NONE',  ( -7.722536802824999214, 1517.050041317280147, 204.5049460973469877 ) ) ;
#22079=CARTESIAN_POINT ( 'NONE',  ( -1.122033430074999893, 1516.972341476009888, 209.8777854684929878 ) ) ;
#22082=CARTESIAN_POINT ( 'NONE',  ( 6.396410510614999545, 1511.623805160500069, 216.5973402254469988 ) ) ;
#22090=CARTESIAN_POINT ( 'NONE',  ( -5.772403812434999892, 1516.676340709600026, 212.3853678745870184 ) ) ;
#22093=EDGE_CURVE ( 'NONE', #42405, #29094, #20728, .T. ) ;
#22096=CARTESIAN_POINT ( 'NONE',  ( -7.709261221864290192, 1516.543067334049965, 210.8692578450250039 ) ) ;
#22097=CARTESIAN_POINT ( 'NONE',  ( -2.284053509485000077, 1516.854133554269993, 210.2586600040969813 ) ) ;
#22100=CARTESIAN_POINT ( 'NONE',  ( -5.513435759310994833, 1508.884207225798491, 201.6131390159873717 ) ) ;
#22107=CARTESIAN_POINT ( 'NONE',  ( 7.549016763624999626, 1510.423579818979988, 204.6938642082269837 ) ) ;
#22112=CARTESIAN_POINT ( 'NONE',  ( 3.455377977254999955, 1516.627618683580067, 216.0573038954169931 ) ) ;
#22117=CARTESIAN_POINT ( 'NONE',  ( -1.708721022705000037, 1516.531533746980131, 201.8006767011069940 ) ) ;
#22120=CARTESIAN_POINT ( 'NONE',  ( -15.52404079726500896, 1511.843510977570077, 220.5312950707671291 ) ) ;
#22124=CARTESIAN_POINT ( 'NONE',  ( 8.321056393114139027, 1511.434991102970116, 203.7361516517889868 ) ) ;
#22152=CARTESIAN_POINT ( 'NONE',  ( -0.1688575540563629906, 1516.885624574960048, 201.4036151776949737 ) ) ;
#22157=CARTESIAN_POINT ( 'NONE',  ( 14.21962190857029995, 1513.293387711980131, 224.3376499801869954 ) ) ;
#22159=ORIENTED_EDGE ( 'NONE', *, *, #18478, .F. ) ;
#22161=CARTESIAN_POINT ( 'NONE',  ( 7.396545043095000160, 1511.069621805459974, 202.7496783316070150 ) ) ;
#22201=CARTESIAN_POINT ( 'NONE',  ( 4.044321679994999919, 1517.001127920769704, 211.4073335515969916 ) ) ;
#22204=CARTESIAN_POINT ( 'NONE',  ( -6.546951720715000533, 1516.606339319019980, 211.9964348928969855 ) ) ;
#22212=CARTESIAN_POINT ( 'NONE',  ( 7.716252052974999387, 1516.810037859429940, 202.1795012402670011 ) ) ;
#22221=DIRECTION ( 'NONE',  ( 0.01484500364079610613, 0.5669078173018522460, -0.8236474686107853049 ) ) ;
#22225=CARTESIAN_POINT ( 'NONE',  ( 6.952166382295000169, 1517.213554313520035, 210.8305935944869987 ) ) ;
#22230=CARTESIAN_POINT ( 'NONE',  ( 7.552141914295000369, 1510.542924508009946, 205.3415595432570058 ) ) ;
#22232=CARTESIAN_POINT ( 'NONE',  ( -2.300729664794999962, 1516.923170579120097, 207.4211391557370234 ) ) ;
#22241=LINE ( 'NONE', #91127, #27086 ) ;
#22248=CARTESIAN_POINT ( 'NONE',  ( 2.487103419534999915, 1516.577434278289957, 215.6681487122470173 ) ) ;
#22250=CARTESIAN_POINT ( 'NONE',  ( 7.712420241246189967, 1516.663706873209776, 208.1377185825360243 ) ) ;
#22255=LINE ( 'NONE', #39647, #37059 ) ;
#22276=CARTESIAN_POINT ( 'NONE',  ( -4.805077596034999843, 1510.399296111369949, 201.5734650597370035 ) ) ;
#22287=ORIENTED_EDGE ( 'NONE', *, *, #43609, .F. ) ;
#22306=ORIENTED_EDGE ( 'NONE', *, *, #91361, .F. ) ;
#22308=CARTESIAN_POINT ( 'NONE',  ( -7.321627547103849665, 1508.611138448550037, 214.6350682845269944 ) ) ;
#22315=VECTOR ( 'NONE', #102512, 1000.000000000000114 ) ;
#22316=CARTESIAN_POINT ( 'NONE',  ( -7.658720568233269965, 1511.445028088800200, 215.2217939408990048 ) ) ;
#22320=CARTESIAN_POINT ( 'NONE',  ( 6.935801261535000428, 1516.621991115350056, 207.9918434378369909 ) ) ;
#22349=CARTESIAN_POINT ( 'NONE',  ( 4.237005577396040223, 1508.610336687640029, 204.5878445095659970 ) ) ;
#22350=CARTESIAN_POINT ( 'NONE',  ( -8.537822636805000087, 1517.051704408389924, 205.6971256312070011 ) ) ;
#22359=CARTESIAN_POINT ( 'NONE',  ( -1.713317447804999949, 1516.660388280709867, 204.5138242629670060 ) ) ;
#22366=CARTESIAN_POINT ( 'NONE',  ( -12.82673418834020040, 1512.305164330070056, 193.9674763234050090 ) ) ;
#22449=CARTESIAN_POINT ( 'NONE',  ( -3.196839497313484380, 1511.813433987939788, 201.1737305778248697 ) ) ;
#22450=DIRECTION ( 'NONE',  ( 1.000000000000000000, 0.000000000000000000, 0.000000000000000000 ) ) ;
#22456=CARTESIAN_POINT ( 'NONE',  ( -5.010423001364999962, 1516.929569650079884, 205.0907035804270038 ) ) ;
#22471=CARTESIAN_POINT ( 'NONE',  ( -6.938478822895000064, 1516.719999691880048, 209.8757167055200057 ) ) ;
#22474=CARTESIAN_POINT ( 'NONE',  ( 2.234897854288949937, 1512.314859079350072, 217.7207912642259942 ) ) ;
#22495=CARTESIAN_POINT ( 'NONE',  ( 7.717505752974999744, 1516.857914730730045, 201.4043401791270185 ) ) ;
#22496=CARTESIAN_POINT ( 'NONE',  ( 2.284053471355000031, 1516.854133554269993, 207.9850318982369970 ) ) ;
#22497=VERTEX_POINT ( 'NONE', #11489 ) ;
#22508=CARTESIAN_POINT ( 'NONE',  ( -6.343099832323124687, 1511.025938544041082, 201.7141561594071959 ) ) ;
#22513=CARTESIAN_POINT ( 'NONE',  ( 6.554764161265000055, 1516.786099423779888, 216.8374711732070068 ) ) ;
#22517=CARTESIAN_POINT ( 'NONE',  ( 2.155390440473662128, 1516.527465808152328, 216.8306986136358887 ) ) ;
#22518=CARTESIAN_POINT ( 'NONE',  ( -3.448206916814999801, 1516.904492006980036, 213.1642637479369853 ) ) ;
#22538=CARTESIAN_POINT ( 'NONE',  ( 0.7365611785030020675, 1517.066898074209803, 204.4979538714769944 ) ) ;
#22554=CARTESIAN_POINT ( 'NONE',  ( 4.329790235878672178, 1515.051704408389924, 205.2060425482754056 ) ) ;
#22565=CARTESIAN_POINT ( 'NONE',  ( 8.280658185778859703, 1511.427938672825576, 204.8576795970872695 ) ) ;
#22572=CARTESIAN_POINT ( 'NONE',  ( -7.501250516761643894, 1510.704533478968187, 215.1450708915986070 ) ) ;
#22579=CARTESIAN_POINT ( 'NONE',  ( -1.129386240404999908, 1516.613712827999962, 201.7984555248870038 ) ) ;
#22582=CARTESIAN_POINT ( 'NONE',  ( 16.42424928753500168, 1513.961173499609913, 194.5327833756670088 ) ) ;
#22587=CARTESIAN_POINT ( 'NONE',  ( 4.802241234501059886, 1508.551704408389924, 204.6921032804660001 ) ) ;
#22593=CARTESIAN_POINT ( 'NONE',  ( -2.827546459321990557, 1516.555886569700306, 201.4122491134000086 ) ) ;
#22596=CARTESIAN_POINT ( 'NONE',  ( -7.686100042665000132, 1512.192993275409890, 211.8118285282569957 ) ) ;
#22616=CARTESIAN_POINT ( 'NONE',  ( -0.7386049428049979992, 1517.122674412569950, 215.6839400395269877 ) ) ;
#22618=AXIS2_PLACEMENT_3D ( 'NONE', #75875, #2373, #36489 ) ;
#22624=CARTESIAN_POINT ( 'NONE',  ( -1.135460355084999762, 1516.790374942449944, 205.8685445508469911 ) ) ;
#22626=CARTESIAN_POINT ( 'NONE',  ( -7.332063977575000280, 1516.939491476980038, 209.1325772641960157 ) ) ;
#22639=CARTESIAN_POINT ( 'NONE',  ( -4.029572678834999699, 1516.858649670339901, 213.1633184439769764 ) ) ;
#22643=CARTESIAN_POINT ( 'NONE',  ( -7.711857127811300394, 1516.642200982649911, 210.2014009544199951 ) ) ;
#22645=CARTESIAN_POINT ( 'NONE',  ( -3.445201526505000000, 1516.743010792419909, 210.8372070624770060 ) ) ;
#22654=CARTESIAN_POINT ( 'NONE',  ( -7.891777529692960869, 1512.314860027450095, 212.0638759934929851 ) ) ;
#22655=EDGE_CURVE ( 'NONE', #107049, #22497, #37237, .T. ) ;
#22657=VECTOR ( 'NONE', #3306, 1000.000000000000000 ) ;
#22665=CARTESIAN_POINT ( 'NONE',  ( -6.941727290454999810, 1516.882217593000178, 216.4530290611770056 ) ) ;
#22670=CARTESIAN_POINT ( 'NONE',  ( 1.125509850285000280, 1517.203017563489766, 201.7827387294869936 ) ) ;
#22695=AXIS2_PLACEMENT_3D ( 'NONE', #1920, #88670, #36057 ) ;
#22698=PLANE ( 'NONE',  #63357 ) ;
#22703=CARTESIAN_POINT ( 'NONE',  ( 5.181410150655000990, 1510.418062979269962, 216.6707182703270291 ) ) ;
#22707=CARTESIAN_POINT ( 'NONE',  ( 12.53206804002270047, 1512.191474810040063, 224.1219235409020030 ) ) ;
#22708=ORIENTED_EDGE ( 'NONE', *, *, #27359, .T. ) ;
#22711=CARTESIAN_POINT ( 'NONE',  ( 6.298908594212630163, 1516.706529261382684, 205.0487668162192563 ) ) ;
#22748=CARTESIAN_POINT ( 'NONE',  ( 0.01265818781360149997, 1516.959716008189844, 210.8316124642570060 ) ) ;
#22752=CARTESIAN_POINT ( 'NONE',  ( -4.609673279564999504, 1516.754149861460064, 212.3872530880769887 ) ) ;
#22758=CARTESIAN_POINT ( 'NONE',  ( 3.452289182574999948, 1517.069378699710114, 202.5601595088670024 ) ) ;
#22767=ORIENTED_EDGE ( 'NONE', *, *, #25752, .T. ) ;
#22775=CARTESIAN_POINT ( 'NONE',  ( 2.300729626665000360, 1516.923170579120097, 210.8225527465970117 ) ) ;
#22781=CARTESIAN_POINT ( 'NONE',  ( 7.557029907284999126, 1510.729589429620091, 203.9615281313170101 ) ) ;
#22782=CARTESIAN_POINT ( 'NONE',  ( 7.710966977635000497, 1516.608208975040043, 207.9930883710269711 ) ) ;
#22783=ORIENTED_EDGE ( 'NONE', *, *, #21447, .F. ) ;
#22802=CARTESIAN_POINT ( 'NONE',  ( 1.709358663124999955, 1516.542957540330008, 216.0554336257470140 ) ) ;
#22804=CARTESIAN_POINT ( 'NONE',  ( 7.710670337728189772, 1516.596880753980031, 207.8068798501710148 ) ) ;
#22822=ORIENTED_EDGE ( 'NONE', *, *, #48148, .F. ) ;
#22836=CARTESIAN_POINT ( 'NONE',  ( -4.813011424114999492, 1510.693074690949970, 201.5657718700469729 ) ) ;
#22847=ORIENTED_EDGE ( 'NONE', *, *, #35885, .T. ) ;
#22850=CARTESIAN_POINT ( 'NONE',  ( 3.487587010899057205, 1508.884207228265495, 213.6131390680183983 ) ) ;
#22871=CARTESIAN_POINT ( 'NONE',  ( -7.558973857277559993, 1511.169205552290123, 215.1889176642449968 ) ) ;
#22876=CARTESIAN_POINT ( 'NONE',  ( 3.445201488374999954, 1516.743010792419909, 207.4064848398570291 ) ) ;
#22886=CARTESIAN_POINT ( 'NONE',  ( -14.97619056944999905, 1512.179780174510142, 221.6162844670500078 ) ) ;
#22889=CARTESIAN_POINT ( 'NONE',  ( 7.644479751013899538, 1517.051704408389924, 209.5582147999029985 ) ) ;
#22890=ADVANCED_FACE ( 'NONE', ( #61099 ), #10667, .T. ) ;
#22904=CARTESIAN_POINT ( 'NONE',  ( 4.487249369889919848, 1509.038630944639863, 205.6342588291649918 ) ) ;
#22912=CARTESIAN_POINT ( 'NONE',  ( -4.491288177712689844, 1508.884219106000046, 205.6342588895329868 ) ) ;
#22914=CARTESIAN_POINT ( 'NONE',  ( 4.610938211375000151, 1516.815231249920089, 205.0813186281270077 ) ) ;
#22924=FACE_OUTER_BOUND ( 'NONE', #86981, .T. ) ;
#22930=CARTESIAN_POINT ( 'NONE',  ( 5.385523159618170297, 1511.435001054559962, 217.7746220610370074 ) ) ;
#22940=CARTESIAN_POINT ( 'NONE',  ( -7.665825202615000222, 1514.407352313670117, 203.3587699272470104 ) ) ;
#22957=CARTESIAN_POINT ( 'NONE',  ( -5.242935297045000276, 1514.523084723979991, 216.7782120477669991 ) ) ;
#22959=CARTESIAN_POINT ( 'NONE',  ( 10.96015508933500016, 1512.830284628050094, 225.0317485278669949 ) ) ;
#23002=EDGE_LOOP ( 'NONE', ( #107902, #69674, #56107, #65279, #28038, #31999, #11542, #50629, #7848, #63714 ) ) ;
#23014=CARTESIAN_POINT ( 'NONE',  ( -4.264264835409092846, 1511.427926070662124, 200.8411546547189630 ) ) ;
#23021=CARTESIAN_POINT ( 'NONE',  ( -2.491188396525000126, 1516.733363207009916, 205.0947945262969938 ) ) ;
#23036=CARTESIAN_POINT ( 'NONE',  ( 5.014195101815000832, 1517.120861839400050, 210.8273123806970091 ) ) ;
#23061=CARTESIAN_POINT ( 'NONE',  ( 6.941100277744999936, 1516.858069504249897, 202.1782432786469883 ) ) ;
#23062=CARTESIAN_POINT ( 'NONE',  ( 4.612671339784999880, 1516.783665406140017, 208.3654117178780041 ) ) ;
#23063=ORIENTED_EDGE ( 'NONE', *, *, #102982, .F. ) ;
#23075=CARTESIAN_POINT ( 'NONE',  ( -5.835879630796829254, 1511.569910118449798, 200.8476638080379928 ) ) ;
#23077=CARTESIAN_POINT ( 'NONE',  ( -5.818054453628801248, 1510.580107419785463, 201.5859676881361224 ) ) ;
#23081=B_SPLINE_CURVE_WITH_KNOTS ( 'NONE', 3,
 ( #22930, #80109, #80666, #29699, #39193, #72282 ),
 .UNSPECIFIED., .F., .F.,
 ( 4, 2, 4 ),
 ( 0.000000000000000000, 0.5000000000000000000, 1.000000000000000000 ),
 .UNSPECIFIED. ) ;
#23083=CARTESIAN_POINT ( 'NONE',  ( -5.779627092215000594, 1516.977993847330026, 216.8424961055369806 ) ) ;
#23086=PLANE ( 'NONE',  #46243 ) ;
#23091=CARTESIAN_POINT ( 'NONE',  ( 6.949265646015000186, 1517.089216728169959, 212.5747629931370000 ) ) ;
#23094=CARTESIAN_POINT ( 'NONE',  ( 4.487249361289610050, 1509.038630936360050, 212.6094330339349767 ) ) ;
#23110=CARTESIAN_POINT ( 'NONE',  ( 7.322105067625000352, 1516.572193931679976, 206.2485165713470110 ) ) ;
#23130=CARTESIAN_POINT ( 'NONE',  ( -11.65724572759794064, 1512.939396361188756, 192.6905581653945774 ) ) ;
#23134=AXIS2_PLACEMENT_3D ( 'NONE', #106417, #91266, #98001 ) ;
#23135=CARTESIAN_POINT ( 'NONE',  ( -3.873571707704530187, 1517.051704409849890, 215.9268917042280123 ) ) ;
#23139=CARTESIAN_POINT ( 'NONE',  ( 7.948111852743331873, 1511.813436676051879, 205.9250125053374632 ) ) ;
#23156=CARTESIAN_POINT ( 'NONE',  ( 5.777745395274999751, 1516.908489800550115, 202.5639360494670029 ) ) ;
#23159=CARTESIAN_POINT ( 'NONE',  ( 15.64724539423500360, 1513.113451381389950, 194.8383152136670162 ) ) ;
#23166=VERTEX_POINT ( 'NONE', #67565 ) ;
#23173=CARTESIAN_POINT ( 'NONE',  ( -7.883543530645000352, 1512.115618635729788, 212.0728052921269864 ) ) ;
#23193=CARTESIAN_POINT ( 'NONE',  ( 7.331183090945000203, 1516.882217593000178, 216.0635732225570109 ) ) ;
#23200=CARTESIAN_POINT ( 'NONE',  ( 0.7356989345870019736, 1517.020847257979995, 205.6609797614169963 ) ) ;
#23203=CARTESIAN_POINT ( 'NONE',  ( 2.873919002525000099, 1516.940252185109784, 209.1085733957019954 ) ) ;
#23215=CARTESIAN_POINT ( 'NONE',  ( -1.704794841465000044, 1517.096587378560116, 213.7484378375869767 ) ) ;
#23219=CARTESIAN_POINT ( 'NONE',  ( -7.712247387419390421, 1516.657104395800161, 210.1350615241800028 ) ) ;
#23220=CARTESIAN_POINT ( 'NONE',  ( -7.323390445344999833, 1516.613712827999962, 210.2512321725070024 ) ) ;
#23237=CARTESIAN_POINT ( 'NONE',  ( 7.717505752974999744, 1516.857914730730045, 216.8393517232070167 ) ) ;
#23242=CARTESIAN_POINT ( 'NONE',  ( 2.290256263724999908, 1517.170721208160103, 202.1706708033170230 ) ) ;
#23243=CARTESIAN_POINT ( 'NONE',  ( -16.00554747716499904, 1513.636261293280086, 223.8634274198670084 ) ) ;
#23264=CIRCLE ( 'NONE', #85869, 7.500000000000000000 ) ;
#23273=CARTESIAN_POINT ( 'NONE',  ( 2.234923043937409926, 1512.341036938790012, 216.7210731156089878 ) ) ;
#23275=ORIENTED_EDGE ( 'NONE', *, *, #63978, .T. ) ;
#23282=CARTESIAN_POINT ( 'NONE',  ( 6.212573846741591410, 1516.720895353221294, 204.9194608389200596 ) ) ;
#23320=CARTESIAN_POINT ( 'NONE',  ( -4.026777524084999449, 1516.718889242609976, 211.4189316860469887 ) ) ;
#23323=CARTESIAN_POINT ( 'NONE',  ( -7.322709724964999722, 1516.596789218710001, 212.3828531017969965 ) ) ;
#23331=CARTESIAN_POINT ( 'NONE',  ( 7.328049280255000575, 1516.809497469189864, 202.5664528150769854 ) ) ;
#23348=CARTESIAN_POINT ( 'NONE',  ( -1.700706814495000163, 1516.923170579120097, 211.4225755968969906 ) ) ;
#23354=CARTESIAN_POINT ( 'NONE',  ( -1.718203501584999904, 1516.898441858519845, 207.4215862561470090 ) ) ;
#23372=CARTESIAN_POINT ( 'NONE',  ( -6.553524415734999664, 1516.882690742909972, 216.0660777183969969 ) ) ;
#23374=CARTESIAN_POINT ( 'NONE',  ( 7.709409411809799550, 1516.548727935889929, 207.4433096617889873 ) ) ;
#23393=EDGE_CURVE ( 'NONE', #58764, #104774, #34363, .T. ) ;
#23404=CARTESIAN_POINT ( 'NONE',  ( -3.385713919165000085, 1511.191277613550028, 201.4988854453669944 ) ) ;
#23421=B_SPLINE_CURVE_WITH_KNOTS ( 'NONE', 5,
 ( #8979, #100820, #15695, #67265, #92421, #86238, #58848, #66714, #93526 ),
 .UNSPECIFIED., .F., .F.,
 ( 6, 3, 6 ),
 ( 0.000000000000000000, 0.5000000000000000000, 1.000000000000000000 ),
 .UNSPECIFIED. ) ;
#23442=CARTESIAN_POINT ( 'NONE',  ( -8.469038851160551218, 1511.685732531849681, 215.1092167430809923 ) ) ;
#23448=CARTESIAN_POINT ( 'NONE',  ( 6.550870144104999682, 1516.727502608469877, 208.3674577492799926 ) ) ;
#23483=CARTESIAN_POINT ( 'NONE',  ( -4.556911044178249881, 1508.729442775010057, 205.2988566914049784 ) ) ;
#23485=CARTESIAN_POINT ( 'NONE',  ( -5.010423001364999962, 1516.929569650079884, 205.0907035804270038 ) ) ;
#23489=CARTESIAN_POINT ( 'NONE',  ( 15.28467102806859934, 1512.548660307890032, 195.8467575762399804 ) ) ;
#23491=ORIENTED_EDGE ( 'NONE', *, *, #33357, .T. ) ;
#23494=CARTESIAN_POINT ( 'NONE',  ( -12.53206807815550050, 1512.191474810040063, 194.1217683614299858 ) ) ;
#23546=EDGE_LOOP ( 'NONE', ( #87040, #72741, #38695, #94531, #41945, #21689, #110369, #107299, #70612, #17318 ) ) ;
#23574=CARTESIAN_POINT ( 'NONE',  ( -4.434000058850124937, 1511.410071747451866, 200.7859701086250936 ) ) ;
#23582=CARTESIAN_POINT ( 'NONE',  ( -2.297085753945000253, 1516.718889242609976, 205.0950684461469962 ) ) ;
#23585=CARTESIAN_POINT ( 'NONE',  ( -17.17760814124009983, 1517.051704413129983, 195.4929600000709797 ) ) ;
#23597=CARTESIAN_POINT ( 'NONE',  ( 2.300729626665000360, 1516.923170579120097, 210.8225527465970117 ) ) ;
#23610=ORIENTED_EDGE ( 'NONE', *, *, #81716, .T. ) ;
#23629=CARTESIAN_POINT ( 'NONE',  ( 6.553524377605000062, 1516.882690742909972, 202.1776141839370098 ) ) ;
#23630=CARTESIAN_POINT ( 'NONE',  ( -2.491655763544999846, 1516.977504706749869, 208.3867361609839861 ) ) ;
#23651=CARTESIAN_POINT ( 'NONE',  ( 0.8692293861700702839, 1516.691033975803066, 216.8349817968451703 ) ) ;
#23652=CARTESIAN_POINT ( 'NONE',  ( -4.610938249504999753, 1516.815231249920089, 213.1623732742069990 ) ) ;
#23655=CARTESIAN_POINT ( 'NONE',  ( 4.678149135874779319, 1508.611352721110052, 212.6094320121750059 ) ) ;
#23669=CARTESIAN_POINT ( 'NONE',  ( -0.7574260232259989456, 1516.837969789639828, 205.8660360680970030 ) ) ;
#23687=CARTESIAN_POINT ( 'NONE',  ( -12.73368289317676094, 1513.317521358512295, 192.3517865229087533 ) ) ;
#23700=ADVANCED_FACE ( 'NONE', ( #86698 ), #25115, .F. ) ;
#23708=CARTESIAN_POINT ( 'NONE',  ( -7.326141170133179337, 1517.051704409989952, 204.8440844730560002 ) ) ;
#23710=CARTESIAN_POINT ( 'NONE',  ( 3.258474578945000033, 1517.083030555940013, 202.5598499717069956 ) ) ;
#23713=CARTESIAN_POINT ( 'NONE',  ( 16.72999343173500009, 1513.736060322960157, 195.1295000578670056 ) ) ;
#23716=CARTESIAN_POINT ( 'NONE',  ( 4.329791490734999471, 1515.051704408389924, 205.7917117663369879 ) ) ;
#23744=CARTESIAN_POINT ( 'NONE',  ( -0.7391220051939990654, 1517.130100026000036, 216.0715493048870144 ) ) ;
#23745=CARTESIAN_POINT ( 'NONE',  ( -8.394782641223070385, 1511.398921086017026, 213.7356158315847665 ) ) ;
#23749=CARTESIAN_POINT ( 'NONE',  ( 5.649719750514999639, 1514.243099272629934, 201.4728115316369781 ) ) ;
#23753=CARTESIAN_POINT ( 'NONE',  ( 5.772403774305000290, 1516.676340709600026, 205.8583240277470168 ) ) ;
#23755=CARTESIAN_POINT ( 'NONE',  ( 5.781585778145000631, 1516.939646076049939, 209.1093989964429909 ) ) ;
#23758=CARTESIAN_POINT ( 'NONE',  ( 6.844666213235000463, 1512.637906871319728, 217.0439743110670179 ) ) ;
#23766=CARTESIAN_POINT ( 'NONE',  ( -0.7365612166329978949, 1517.066898074209803, 213.7457380308570123 ) ) ;
#23771=CARTESIAN_POINT ( 'NONE',  ( -4.028611259245000298, 1516.744381837270112, 210.2562039408269925 ) ) ;
#23784=CARTESIAN_POINT ( 'NONE',  ( -5.004475612664999851, 1517.026025493960105, 216.8437538584669824 ) ) ;
#23789=CARTESIAN_POINT ( 'NONE',  ( 4.615017327834999961, 1516.987478262539980, 202.5620478758069964 ) ) ;
#23790=CARTESIAN_POINT ( 'NONE',  ( -15.46083485256500012, 1513.125294087170005, 223.3378070712669796 ) ) ;
#23791=CARTESIAN_POINT ( 'NONE',  ( 6.520293663361448111, 1509.032998980578441, 216.3821515562998457 ) ) ;
#23808=CARTESIAN_POINT ( 'NONE',  ( -3.861663332592479847, 1508.610718243669908, 213.8016401467760090 ) ) ;
#23817=FACE_OUTER_BOUND ( 'NONE', #69412, .T. ) ;
#23852=EDGE_CURVE ( 'NONE', #100324, #107049, #100055, .T. ) ;
#23861=CARTESIAN_POINT ( 'NONE',  ( -6.546302780145000000, 1516.577434278289957, 211.6089493897669911 ) ) ;
#23864=CARTESIAN_POINT ( 'NONE',  ( 5.785582913545000316, 1516.981965530290154, 213.1542438721070027 ) ) ;
#23871=CARTESIAN_POINT ( 'NONE',  ( 1.124894050234999998, 1517.194816588360027, 202.1703287997270309 ) ) ;
#23883=CARTESIAN_POINT ( 'NONE',  ( -2.344512381655610156, 1516.526058395550081, 201.4130302485380071 ) ) ;
#23886=CARTESIAN_POINT ( 'NONE',  ( 0.7578857918350010436, 1516.872851364150165, 211.6022732247369902 ) ) ;
#23892=CARTESIAN_POINT ( 'NONE',  ( 3.251394362135000105, 1516.757508073510053, 207.4061414411269766 ) ) ;
#23909=CARTESIAN_POINT ( 'NONE',  ( -7.328049318385000177, 1516.809497469189864, 215.6772390872569929 ) ) ;
#23911=CARTESIAN_POINT ( 'NONE',  ( 7.719201501412129574, 1516.922672751009941, 209.0804826056520085 ) ) ;
#23940=CARTESIAN_POINT ( 'NONE',  ( -5.110470226864999965, 1511.399604276809896, 200.8758674234269961 ) ) ;
#23983=CARTESIAN_POINT ( 'NONE',  ( 6.938478784765000462, 1516.719999691880048, 208.3679751968140010 ) ) ;
#24016=CARTESIAN_POINT ( 'NONE',  ( 2.865911516645000212, 1516.906233342200039, 205.6598507734169914 ) ) ;
#24024=CARTESIAN_POINT ( 'NONE',  ( -12.57832850835009886, 1512.205851781539877, 194.0924024796699996 ) ) ;
#24044=B_SPLINE_SURFACE_WITH_KNOTS ( 'NONE', 5, 5, ( 
 ( #86376, #67951, #8556, #35426, #102060, #69613 ),
 ( #27034, #95337, #18598, #24784, #58986, #93113 ),
 ( #16384, #25342, #42175, #70177, #56511, #47554 ),
 ( #29095, #78540, #80601, #97393, #104288, #38047 ),
 ( #63280, #20663, #107991, #35989, #4453, #30175 ),
 ( #12832, #10220, #22308, #72224, #44398, #5545 ) ),
 .UNSPECIFIED., .F., .F., .F.,
 ( 6, 6 ),
 ( 6, 6 ),
 ( 5.893388896111249942, 9.819930328988748514 ),
 ( -0.0002947352087483990084, 0.5000000000000000000 ),
 .UNSPECIFIED. ) ;
#24109=CARTESIAN_POINT ( 'NONE',  ( -2.983385501069631740, 1512.076650117638792, 201.2296962218204328 ) ) ;
#24115=CARTESIAN_POINT ( 'NONE',  ( 2.865588684285000021, 1516.890356958860139, 205.8536102114670143 ) ) ;
#24126=CARTESIAN_POINT ( 'NONE',  ( -16.78503329099363839, 1513.553906385462142, 222.3493531866972148 ) ) ;
#24130=CARTESIAN_POINT ( 'NONE',  ( -3.251394400264999707, 1516.757508073510053, 210.8375504612070017 ) ) ;
#24159=CARTESIAN_POINT ( 'NONE',  ( -6.554764199395000546, 1516.786099423779888, 201.4062207291269999 ) ) ;
#24160=CARTESIAN_POINT ( 'NONE',  ( 7.326072144144999854, 1516.714320817460020, 208.3685457967989976 ) ) ;
#24164=CARTESIAN_POINT ( 'NONE',  ( 3.294745913766051082, 1511.738168994502985, 217.0981794534744722 ) ) ;
#24165=EDGE_LOOP ( 'NONE', ( #89231, #102520, #108476, #65526 ) ) ;
#24182=CARTESIAN_POINT ( 'NONE',  ( 4.616861508414999093, 1516.666407245520077, 216.8343369232169948 ) ) ;
#24186=CARTESIAN_POINT ( 'NONE',  ( 0.6913041155385422076, 1516.736466343139227, 216.8361714852529190 ) ) ;
#24187=CARTESIAN_POINT ( 'NONE',  ( 2.296124850935000072, 1516.677239312369920, 213.7299927514870319 ) ) ;
#24208=CARTESIAN_POINT ( 'NONE',  ( 4.609673241434999902, 1516.754149861460064, 205.8564388142570181 ) ) ;
#24224=DIRECTION ( 'NONE',  ( -1.643460219210440075E-32, 1.000000000000000000, -6.123233995736769734E-17 ) ) ;
#24231=CARTESIAN_POINT ( 'NONE',  ( -14.30569713659541620, 1514.201165865805024, 192.5944094235600801 ) ) ;
#24260=CARTESIAN_POINT ( 'NONE',  ( -3.457266643525000127, 1516.691414181030041, 203.3491180233569935 ) ) ;
#24263=CARTESIAN_POINT ( 'NONE',  ( 16.20130417443500193, 1512.842772631639946, 197.8702892259670136 ) ) ;
#24295=CARTESIAN_POINT ( 'NONE',  ( -2.871580426725000024, 1517.129577905929864, 216.0720609035170128 ) ) ;
#24296=CARTESIAN_POINT ( 'NONE',  ( -8.510911714697881436, 1511.398736650778574, 214.0857784337908356 ) ) ;
#24305=CARTESIAN_POINT ( 'NONE',  ( -6.561995998525000040, 1517.083030555940013, 205.8633713531569924 ) ) ;
#24307=CARTESIAN_POINT ( 'NONE',  ( -1.906501101195560124E-08, 1517.020990152690047, 209.1218459511669892 ) ) ;
#24318=CARTESIAN_POINT ( 'NONE',  ( 3.458526497885000328, 1516.742629295279812, 214.1194197574270106 ) ) ;
#24324=CARTESIAN_POINT ( 'NONE',  ( -4.608417544644999531, 1516.691389976299888, 211.6120918846570191 ) ) ;
#24345=CARTESIAN_POINT ( 'NONE',  ( -6.944231786295000042, 1516.882690742909972, 202.5683215544970039 ) ) ;
#24346=CARTESIAN_POINT ( 'NONE',  ( 7.112123167431945170, 1509.032357809081304, 215.8638901911494941 ) ) ;
#24374=CARTESIAN_POINT ( 'NONE',  ( 2.258825551794999775, 1511.942942747529969, 216.7106486523369995 ) ) ;
#24380=ORIENTED_EDGE ( 'NONE', *, *, #80990, .F. ) ;
#24420=CARTESIAN_POINT ( 'NONE',  ( 0.01327404799950150129, 1516.939877939420057, 212.5773418040870126 ) ) ;
#24422=CARTESIAN_POINT ( 'NONE',  ( 5.381311975764999644, 1511.468585915670019, 217.4468093916769931 ) ) ;
#24426=CARTESIAN_POINT ( 'NONE',  ( -7.331183129075000693, 1516.882217593000178, 202.1801186797769674 ) ) ;
#24439=CARTESIAN_POINT ( 'NONE',  ( 5.012938863775000087, 1517.051603658920158, 211.6026598552170128 ) ) ;
#24445=CARTESIAN_POINT ( 'NONE',  ( -3.269984819434999856, 1516.999105586269934, 207.4194399470370058 ) ) ;
#24458=PLANE ( 'NONE',  #59453 ) ;
#24459=CARTESIAN_POINT ( 'NONE',  ( -4.999456428534999830, 1516.830644417779922, 213.7431138541670066 ) ) ;
#24462=CARTESIAN_POINT ( 'NONE',  ( 3.261635932824999973, 1516.613881697390070, 216.0569793506570022 ) ) ;
#24496=LINE ( 'NONE', #75497, #8890 ) ;
#24537=CARTESIAN_POINT ( 'NONE',  ( -3.460866208815000178, 1517.020847257979995, 208.3861469975149987 ) ) ;
#24545=CARTESIAN_POINT ( 'NONE',  ( -14.82736039673160100, 1512.135905030570029, 221.4210449998400065 ) ) ;
#24568=CARTESIAN_POINT ( 'NONE',  ( -7.722536802824999214, 1517.050041317280147, 204.5049460973469877 ) ) ;
#24643=DIRECTION ( 'NONE',  ( 0.7384854939282339270, -4.128709092058508552E-17, -0.6742693640212139572 ) ) ;
#24647=FACE_OUTER_BOUND ( 'NONE', #39695, .T. ) ;
#24655=CARTESIAN_POINT ( 'NONE',  ( -4.042729840925000317, 1516.919782530640077, 205.8674445284970034 ) ) ;
#24666=CARTESIAN_POINT ( 'NONE',  ( -16.67556694314024668, 1513.118420038618069, 221.3657088474023169 ) ) ;
#24672=CARTESIAN_POINT ( 'NONE',  ( -0.7351098092479989576, 1516.977504706749869, 211.6135016956469883 ) ) ;
#24696=CARTESIAN_POINT ( 'NONE',  ( 3.724929213431543484, 1516.669760784861410, 215.6322040485396485 ) ) ;
#24702=CARTESIAN_POINT ( 'NONE',  ( -0.7533001734329990429, 1516.714320817460020, 201.7957737879569891 ) ) ;
#24703=CARTESIAN_POINT ( 'NONE',  ( -7.719640941135000212, 1516.939452820819952, 209.1319487995289705 ) ) ;
#24706=CARTESIAN_POINT ( 'NONE',  ( 2.994315780531499271, 1512.053483454412799, 217.0162803964337854 ) ) ;
#24719=FACE_OUTER_BOUND ( 'NONE', #63119, .T. ) ;
#24723=CARTESIAN_POINT ( 'NONE',  ( 1.708092266164999984, 1516.523379810429788, 216.8305916180169959 ) ) ;
#24727=CARTESIAN_POINT ( 'NONE',  ( 0.9839655838812769728, 1516.663585454903341, 216.8342630320297246 ) ) ;
#24728=CARTESIAN_POINT ( 'NONE',  ( -0.7365612166329978949, 1517.066898074209803, 213.7457380308570123 ) ) ;
#24731=CARTESIAN_POINT ( 'NONE',  ( 4.987080938901260474, 1508.551704408389924, 213.0804906078760155 ) ) ;
#24745=CARTESIAN_POINT ( 'NONE',  ( 5.772403774305000290, 1516.676340709600026, 205.8583240277470168 ) ) ;
#24768=CARTESIAN_POINT ( 'NONE',  ( -14.79463505727891004, 1514.566409480255743, 192.8705245058147568 ) ) ;
#24784=CARTESIAN_POINT ( 'NONE',  ( -6.120117913879710159, 1508.729257035799947, 216.5649250963629981 ) ) ;
#24787=CARTESIAN_POINT ( 'NONE',  ( -15.00364260096500146, 1514.335759350750095, 193.0073477423669885 ) ) ;
#24793=CARTESIAN_POINT ( 'NONE',  ( -7.720650173434999708, 1516.977993847330026, 203.3422188780170075 ) ) ;
#24796=CARTESIAN_POINT ( 'NONE',  ( 15.87603342113500027, 1512.359593911809952, 198.0975645610670028 ) ) ;
#24809=CARTESIAN_POINT ( 'NONE',  ( -3.487592467065000257, 1509.038615934169911, 213.6090957241370063 ) ) ;
#24822=CARTESIAN_POINT ( 'NONE',  ( 5.818574454934999807, 1514.487275757750012, 201.4289454835769959 ) ) ;
#24830=AXIS2_PLACEMENT_3D ( 'NONE', #105644, #106717, #64198 ) ;
#24832=CARTESIAN_POINT ( 'NONE',  ( 4.616861508414999093, 1516.666407245520077, 216.8343369232169948 ) ) ;
#24833=CARTESIAN_POINT ( 'NONE',  ( -7.924515700752487568, 1511.889608912520998, 212.2345484715577584 ) ) ;
#24842=CARTESIAN_POINT ( 'NONE',  ( 4.028307740155000261, 1516.797038924770050, 205.8554964580370097 ) ) ;
#24847=CARTESIAN_POINT ( 'NONE',  ( 8.126234247455000670, 1514.923664147150021, 215.2485921136969864 ) ) ;
#24857=CARTESIAN_POINT ( 'NONE',  ( -6.548821979184999975, 1516.688761843659904, 213.1592242262869945 ) ) ;
#24860=CARTESIAN_POINT ( 'NONE',  ( -7.722579826676089887, 1517.051704428850144, 208.6871515679729896 ) ) ;
#24861=CARTESIAN_POINT ( 'NONE',  ( -5.771149113014999443, 1516.616791731099966, 211.6102065995370083 ) ) ;
#24872=CARTESIAN_POINT ( 'NONE',  ( 11.46842531143500032, 1512.169992403149990, 225.2408885909669891 ) ) ;
#24878=CARTESIAN_POINT ( 'NONE',  ( 2.483322453895000059, 1517.139039350860003, 202.5585910412470128 ) ) ;
#24894=ORIENTED_EDGE ( 'NONE', *, *, #91338, .T. ) ;
#24898=CARTESIAN_POINT ( 'NONE',  ( -4.237005615526038937, 1508.610336687640029, 213.6558473927679813 ) ) ;
#24903=CARTESIAN_POINT ( 'NONE',  ( 13.89942583313499824, 1515.383078152259941, 193.2773559084670012 ) ) ;
#24912=EDGE_CURVE ( 'NONE', #40123, #19916, #16811, .T. ) ;
#24916=ORIENTED_EDGE ( 'NONE', *, *, #28118, .F. ) ;
#24929=CARTESIAN_POINT ( 'NONE',  ( 9.090771158884999537, 1511.924334870729808, 220.7486671641670171 ) ) ;
#24948=EDGE_CURVE ( 'NONE', #53542, #44160, #78775, .T. ) ;
#24959=CARTESIAN_POINT ( 'NONE',  ( 0.7568986996720019622, 1516.805675336850072, 213.1530147380969993 ) ) ;
#24960=CARTESIAN_POINT ( 'NONE',  ( 5.551188673975000043, 1510.480349266450048, 216.6723492941569873 ) ) ;
#24966=CARTESIAN_POINT ( 'NONE',  ( 6.939219482805000005, 1516.783701990830195, 203.3409846960470020 ) ) ;
#24982=CARTESIAN_POINT ( 'NONE',  ( -4.987078451384999944, 1508.551704408389924, 205.1631965221770031 ) ) ;
#24985=VECTOR ( 'NONE', #13481, 1000.000000000000227 ) ;
#24986=CARTESIAN_POINT ( 'NONE',  ( -5.770883602015000058, 1516.603620185149794, 211.4160555996369908 ) ) ;
#24990=CARTESIAN_POINT ( 'NONE',  ( 4.612671339784999880, 1516.783665406140017, 208.3654117178780041 ) ) ;
#24993=CARTESIAN_POINT ( 'NONE',  ( -1.906499758064230099E-08, 1516.051704408390151, 209.1218459511669892 ) ) ;
#25009=CARTESIAN_POINT ( 'NONE',  ( -2.286446363765000100, 1517.042661899400173, 213.7475398352470108 ) ) ;
#25012=CARTESIAN_POINT ( 'NONE',  ( 5.005071008295000290, 1516.710692850270107, 216.4473877573669824 ) ) ;
#25023=AXIS2_PLACEMENT_3D ( 'NONE', #73060, #29933, #20972 ) ;
#25052=ORIENTED_EDGE ( 'NONE', *, *, #55754, .F. ) ;
#25067=CARTESIAN_POINT ( 'NONE',  ( -8.104522071583946996, 1514.095142040220935, 201.7913770512302563 ) ) ;
#25085=CARTESIAN_POINT ( 'NONE',  ( -7.679927622135040544, 1511.009256124219974, 214.7417639624250114 ) ) ;
#25090=CARTESIAN_POINT ( 'NONE',  ( -1.127928371535000140, 1516.989863902050047, 209.1319708558790182 ) ) ;
#25101=CARTESIAN_POINT ( 'NONE',  ( -15.23581460173349988, 1513.231391186749988, 223.2758740717220007 ) ) ;
#25115=PLANE ( 'NONE',  #74240 ) ;
#25125=CARTESIAN_POINT ( 'NONE',  ( -4.623788007495000407, 1516.947419719950176, 205.6726967363569827 ) ) ;
#25129=CARTESIAN_POINT ( 'NONE',  ( 15.22870587831669908, 1512.406412988020065, 196.0902778419350057 ) ) ;
#25132=ORIENTED_EDGE ( 'NONE', *, *, #57524, .T. ) ;
#25174=CARTESIAN_POINT ( 'NONE',  ( -1.703779643355000095, 1517.057265928030120, 213.1670284501570052 ) ) ;
#25202=DIRECTION ( 'NONE',  ( -0.8164965809278522668, -0.5773502691894472072, 0.000000000000000000 ) ) ;
#25217=CARTESIAN_POINT ( 'NONE',  ( -0.7576635715699989726, 1516.855632454399938, 206.2537338009369989 ) ) ;
#25226=CARTESIAN_POINT ( 'NONE',  ( -16.78766067578666465, 1513.436209035151933, 222.1126914816819635 ) ) ;
#25230=CARTESIAN_POINT ( 'NONE',  ( 7.726331925474999807, 1517.194972660189933, 211.4133602680070112 ) ) ;
#25248=AXIS2_PLACEMENT_3D ( 'NONE', #82644, #315, #61337 ) ;
#25259=CARTESIAN_POINT ( 'NONE',  ( -7.717505791104999346, 1516.857914730730045, 201.4043401791270185 ) ) ;
#25260=CARTESIAN_POINT ( 'NONE',  ( -1.127928371535000140, 1516.989863902050047, 209.1319708558790182 ) ) ;
#25264=CARTESIAN_POINT ( 'NONE',  ( 3.806606270525944247, 1511.520894735526781, 217.2557709082670101 ) ) ;
#25283=CARTESIAN_POINT ( 'NONE',  ( -4.364191719525152280, 1509.032014410905276, 205.0059630720760140 ) ) ;
#25287=CARTESIAN_POINT ( 'NONE',  ( 4.554954796684620000, 1508.731366863229823, 212.6094326720719891 ) ) ;
#25300=CARTESIAN_POINT ( 'NONE',  ( 7.709681268295000223, 1516.559109716219837, 206.2491454149069909 ) ) ;
#25305=EDGE_CURVE ( 'NONE', #110638, #80871, #304, .T. ) ;
#25342=CARTESIAN_POINT ( 'NONE',  ( -6.551899188738270041, 1508.551566291330118, 216.0836886511409887 ) ) ;
#25353=CARTESIAN_POINT ( 'NONE',  ( -4.620008245204999753, 1516.777260590120022, 203.3472363101570011 ) ) ;
#25380=CARTESIAN_POINT ( 'NONE',  ( 5.649719750514999639, 1514.243099272629934, 201.4728115316369781 ) ) ;
#25385=CARTESIAN_POINT ( 'NONE',  ( 7.006565492904999637, 1516.551704408390151, 221.0781589314669873 ) ) ;
#25388=CARTESIAN_POINT ( 'NONE',  ( -5.778999811904999895, 1516.955859323880077, 216.4549161051170074 ) ) ;
#25389=CARTESIAN_POINT ( 'NONE',  ( -8.053242336889125497, 1511.610022726261377, 212.6696535251155069 ) ) ;
#25392=CARTESIAN_POINT ( 'NONE',  ( 7.098162965876308128, 1512.239113741298070, 201.9714854511515796 ) ) ;
#25395=CARTESIAN_POINT ( 'NONE',  ( 3.252530615595000452, 1516.827328999679821, 206.2418890071470230 ) ) ;
#25400=CARTESIAN_POINT ( 'NONE',  ( 7.653848867554999380, 1514.071098020780028, 215.6856573818370180 ) ) ;
#25409=CARTESIAN_POINT ( 'NONE',  ( -4.031142389804999837, 1516.929569650079884, 214.1322689334670031 ) ) ;
#25412=CARTESIAN_POINT ( 'NONE',  ( 6.961842680912760706, 1508.551566291330118, 215.6737451208340133 ) ) ;
#25413=CARTESIAN_POINT ( 'NONE',  ( -1.118353254094999860, 1516.977201124959947, 211.6155430111569729 ) ) ;
#25433=CARTESIAN_POINT ( 'NONE',  ( 4.032397901875000024, 1516.981965530290154, 203.3362630185569913 ) ) ;
#25475=ORIENTED_EDGE ( 'NONE', *, *, #105774, .F. ) ;
#25495=ORIENTED_EDGE ( 'NONE', *, *, #54284, .F. ) ;
#25516=CARTESIAN_POINT ( 'NONE',  ( 1.713317409674999903, 1516.660388280709867, 213.7298676393670291 ) ) ;
#25518=B_SPLINE_SURFACE_WITH_KNOTS ( 'NONE', 5, 5, ( 
 ( #45578, #20331, #45026, #28750, #94845, #11410, #18121, #18665, #79720 ),
 ( #54535, #88669, #11947, #46128, #52317, #86440, #9731, #78039, #21958 ),
 ( #81334, #4648, #108197, #23075, #12495, #65666, #38786, #108752, #6294 ),
 ( #64027, #89749, #65117, #21415, #97609, #47753, #90287, #98698, #81888 ),
 ( #13568, #89202, #48318, #13021, #55626, #46677, #5191, #47208, #80809 ),
 ( #40441, #29841, #83001, #39346, #64579, #72962, #74617, #107100, #30941 ) ),
 .UNSPECIFIED., .F., .F., .F.,
 ( 6, 6 ),
 ( 6, 3, 6 ),
 ( 4.238752792103120726, 5.659133035216879826 ),
 ( 0.000000000000000000, 0.5000000000000000000, 1.002061266616879998 ),
 .UNSPECIFIED. ) ;
#25526=CARTESIAN_POINT ( 'NONE',  ( -0.01289782690309849988, 1516.939723362869927, 204.1155860834069813 ) ) ;
#25539=CARTESIAN_POINT ( 'NONE',  ( -12.20279397044791381, 1516.551704399887512, 191.9693043941118731 ) ) ;
#25540=CARTESIAN_POINT ( 'NONE',  ( 7.725990161824999980, 1517.181921232829836, 211.6070516194370157 ) ) ;
#25544=CARTESIAN_POINT ( 'NONE',  ( 6.938478784765000462, 1516.719999691880048, 208.3679751968140010 ) ) ;
#25561=CARTESIAN_POINT ( 'NONE',  ( -2.868433836634999512, 1517.020727862619879, 214.1341630384669941 ) ) ;
#25579=DIRECTION ( 'NONE',  ( 0.8236474686107853049, 0.5669078173018522460, 0.01484500364079610613 ) ) ;
#25601=CARTESIAN_POINT ( 'NONE',  ( -1.274602950971519988, 1516.603953730839976, 201.4109903819569922 ) ) ;
#25623=EDGE_CURVE ( 'NONE', #18936, #84966, #63611, .T. ) ;
#25631=DIRECTION ( 'NONE',  ( 0.000000000000000000, -1.000000000000000000, 6.123233995736769734E-17 ) ) ;
#25648=CARTESIAN_POINT ( 'NONE',  ( -1.906501101195560124E-08, 1517.020990152690047, 209.1218459511669892 ) ) ;
#25650=CARTESIAN_POINT ( 'NONE',  ( -15.90990259576500065, 1516.814170398969964, 224.3246417466669982 ) ) ;
#25656=CARTESIAN_POINT ( 'NONE',  ( -15.03014123622689979, 1513.722010161890012, 223.7517583984009946 ) ) ;
#25679=CARTESIAN_POINT ( 'NONE',  ( -1.715704529104999931, 1516.757508073510053, 205.8704515699670026 ) ) ;
#25728=CARTESIAN_POINT ( 'NONE',  ( 3.460101851884999746, 1516.812923327049930, 213.1504765548870068 ) ) ;
#25732=EDGE_LOOP ( 'NONE', ( #73133, #17550, #68180, #81637, #5603, #6573, #100267, #7842 ) ) ;
#25752=EDGE_CURVE ( 'NONE', #89980, #56739, #68961, .T. ) ;
#25758=DIRECTION ( 'NONE',  ( -0.4999999999998399614, 0.7071067811867740582, -0.4999999999998399614 ) ) ;
#25773=CARTESIAN_POINT ( 'NONE',  ( 7.709681268295000223, 1516.559109716219837, 206.2491454149069909 ) ) ;
#25782=CARTESIAN_POINT ( 'NONE',  ( -16.19963475833718647, 1512.859148089886276, 220.4046715791462532 ) ) ;
#25786=CARTESIAN_POINT ( 'NONE',  ( 2.881222757585000238, 1516.891731298979948, 211.5992195760969707 ) ) ;
#25808=CARTESIAN_POINT ( 'NONE',  ( 3.644878262961745108, 1516.661627594595529, 215.6772027093610120 ) ) ;
#25813=CARTESIAN_POINT ( 'NONE',  ( 2.869693458934999608, 1517.070197312179971, 203.3343689375869872 ) ) ;
#25814=CARTESIAN_POINT ( 'NONE',  ( -1.709766532154999963, 1516.959716008189844, 209.1345041580460133 ) ) ;
#25817=CARTESIAN_POINT ( 'NONE',  ( 4.487065301914353377, 1511.405768592958111, 217.4750366866610420 ) ) ;
#25837=CARTESIAN_POINT ( 'NONE',  ( 1.514120138310384167, 1516.566819146330090, 216.8317291170628209 ) ) ;
#25849=CARTESIAN_POINT ( 'NONE',  ( -15.83297151926499602, 1514.812393650459853, 224.4015772493669942 ) ) ;
#25856=CARTESIAN_POINT ( 'NONE',  ( 2.864326087304999824, 1516.826109302209943, 206.6287721023469999 ) ) ;
#25876=CIRCLE ( 'NONE', #74204, 1.000060826959960236 ) ;
#25881=CARTESIAN_POINT ( 'NONE',  ( -12.43458797219282808, 1513.190411469892297, 192.3969053724739808 ) ) ;
#25889=DIRECTION ( 'NONE',  ( 0.000000000000000000, -1.000000000000000000, 6.123233995736769734E-17 ) ) ;
#25907=CARTESIAN_POINT ( 'NONE',  ( -2.294209667535000108, 1516.603620185149794, 203.3509623682169831 ) ) ;
#25919=ORIENTED_EDGE ( 'NONE', *, *, #55366, .F. ) ;
#25930=CARTESIAN_POINT ( 'NONE',  ( -2.864972154145000172, 1516.859514182039902, 212.0024388992169975 ) ) ;
#25935=CARTESIAN_POINT ( 'NONE',  ( 7.381112317704999981, 1512.341575225269935, 202.3461611114969969 ) ) ;
#25941=CARTESIAN_POINT ( 'NONE',  ( 16.43125155181079933, 1512.939392325030667, 197.4646673575076363 ) ) ;
#25944=CARTESIAN_POINT ( 'NONE',  ( -8.152189559000989405, 1511.505225070767210, 212.9862058279672681 ) ) ;
#25950=CARTESIAN_POINT ( 'NONE',  ( 3.251888829344999898, 1516.793978928989873, 206.6294022811970024 ) ) ;
#25956=CARTESIAN_POINT ( 'NONE',  ( 7.641777858334999785, 1513.965983108860200, 215.0411262584869974 ) ) ;
#25962=CARTESIAN_POINT ( 'NONE',  ( 5.385523159618170297, 1511.435001054559962, 217.7746220610370074 ) ) ;
#25964=CARTESIAN_POINT ( 'NONE',  ( -2.869693497065000098, 1517.070197312179971, 214.9093229647470196 ) ) ;
#25968=CARTESIAN_POINT ( 'NONE',  ( 3.462948796544999652, 1516.956048353049937, 211.4063724288770061 ) ) ;
#25978=CARTESIAN_POINT ( 'NONE',  ( -7.552141952424999971, 1510.542924508009946, 212.9021323590669965 ) ) ;
#25981=DIRECTION ( 'NONE',  ( 1.000000000000000000, 0.000000000000000000, 0.000000000000000000 ) ) ;
#25986=CARTESIAN_POINT ( 'NONE',  ( 7.712490952985000980, 1516.666407245520077, 204.5049844236870058 ) ) ;
#26025=ORIENTED_EDGE ( 'NONE', *, *, #80964, .T. ) ;
#26027=CARTESIAN_POINT ( 'NONE',  ( 6.929954890342334473, 1516.587827493819759, 206.2351373589867762 ) ) ;
#26045=CARTESIAN_POINT ( 'NONE',  ( 7.501250477999354516, 1510.704533481359476, 203.0986210076053169 ) ) ;
#26065=CARTESIAN_POINT ( 'NONE',  ( 5.784008635194999748, 1516.911981270829983, 214.1231845985469988 ) ) ;
#26075=CARTESIAN_POINT ( 'NONE',  ( -1.712644754285000070, 1516.636036526019780, 204.1262224792070015 ) ) ;
#26087=CARTESIAN_POINT ( 'NONE',  ( 8.788316489185000080, 1511.741868877540128, 202.8695794779170001 ) ) ;
#26092=CARTESIAN_POINT ( 'NONE',  ( -0.7353365779029981120, 1516.995911393979895, 212.0011643880069698 ) ) ;
#26096=CARTESIAN_POINT ( 'NONE',  ( 7.713648834184999359, 1516.710624944440042, 208.3691743819339877 ) ) ;
#26113=CARTESIAN_POINT ( 'NONE',  ( 2.489617538345000103, 1516.665179208830068, 214.1178407578070164 ) ) ;
#26116=CARTESIAN_POINT ( 'NONE',  ( -2.872836660654999985, 1517.158319634930194, 216.8472181024670249 ) ) ;
#26118=CARTESIAN_POINT ( 'NONE',  ( 7.722580314247720068, 1517.051704408590012, 209.5565402419049974 ) ) ;
#26127=FACE_OUTER_BOUND ( 'NONE', #25732, .T. ) ;
#26136=CARTESIAN_POINT ( 'NONE',  ( 7.260305599174779800, 1509.032998980356297, 202.6015522927725669 ) ) ;
#26150=VECTOR ( 'NONE', #4967, 1000.000000000000114 ) ;
#26156=CARTESIAN_POINT ( 'NONE',  ( -1.810518240848369986, 1516.538255842539911, 201.4127107417070022 ) ) ;
#26202=CARTESIAN_POINT ( 'NONE',  ( 3.462835627365000057, 1517.038650117239968, 210.2415636864969883 ) ) ;
#26220=CARTESIAN_POINT ( 'NONE',  ( -2.493697079054999932, 1516.977201124959947, 208.0034927161370035 ) ) ;
#26238=CARTESIAN_POINT ( 'NONE',  ( 3.446329775655000205, 1516.812046502680005, 206.2422037788969931 ) ) ;
#26249=PLANE ( 'NONE',  #77115 ) ;
#26278=APPLICATION_CONTEXT ( 'automotive_design' ) ;
#26288=CARTESIAN_POINT ( 'NONE',  ( 7.722536764694999611, 1517.050041317280147, 213.7387458049869906 ) ) ;
#26329=CARTESIAN_POINT ( 'NONE',  ( 2.477986732234999767, 1516.922519270759949, 205.8529865360470126 ) ) ;
#26338=CARTESIAN_POINT ( 'NONE',  ( -16.52740844507182416, 1514.201209519881331, 223.4276059376695400 ) ) ;
#26343=CARTESIAN_POINT ( 'NONE',  ( -6.933587693644999383, 1516.542957540330008, 210.8312046333570038 ) ) ;
#26370=CARTESIAN_POINT ( 'NONE',  ( 7.321627508978070686, 1508.611138448550037, 203.6086236178030333 ) ) ;
#26375=CARTESIAN_POINT ( 'NONE',  ( -2.873958889724999910, 1516.588006113850042, 202.1873174023370154 ) ) ;
#26376=CARTESIAN_POINT ( 'NONE',  ( 2.879318417774999972, 1516.995911393979895, 209.8571825100049750 ) ) ;
#26379=CARTESIAN_POINT ( 'NONE',  ( 3.965270473948547814, 1511.478973222888044, 217.3060377250480713 ) ) ;
#26380=EDGE_LOOP ( 'NONE', ( #14121, #91669, #55313, #8849 ) ) ;
#26389=CARTESIAN_POINT ( 'NONE',  ( -16.95839816991464843, 1517.034034369547498, 195.0103398635659744 ) ) ;
#26400=ORIENTED_EDGE ( 'NONE', *, *, #86549, .T. ) ;
#26411=FACE_OUTER_BOUND ( 'NONE', #61363, .T. ) ;
#26415=CARTESIAN_POINT ( 'NONE',  ( -16.25489180516500198, 1512.123798513659949, 221.6559977385670095 ) ) ;
#26420=CARTESIAN_POINT ( 'NONE',  ( 6.933616821004999764, 1516.548716157039962, 206.8295387017270173 ) ) ;
#26435=CARTESIAN_POINT ( 'NONE',  ( -2.933667460025000118, 1512.215430505229961, 201.2384290929069834 ) ) ;
#26468=CARTESIAN_POINT ( 'NONE',  ( -1.711311266675000109, 1516.591755933730155, 203.3510257909670145 ) ) ;
#26471=CARTESIAN_POINT ( 'NONE',  ( 15.83297148113499730, 1514.812393650459853, 193.8421146529669841 ) ) ;
#26474=PLANE ( 'NONE',  #104916 ) ;
#26494=CARTESIAN_POINT ( 'NONE',  ( 2.299014030735000436, 1516.811292230880099, 211.9858893885470081 ) ) ;
#26497=CARTESIAN_POINT ( 'NONE',  ( 6.259132986314999592, 1514.370494773840164, 201.3780798503470066 ) ) ;
#26503=CARTESIAN_POINT ( 'NONE',  ( -7.951263648584999899, 1511.644799026709961, 215.1357399413169844 ) ) ;
#26504=CARTESIAN_POINT ( 'NONE',  ( 16.19963472355905054, 1512.859148090011331, 197.8390203186946223 ) ) ;
#26507=CARTESIAN_POINT ( 'NONE',  ( -2.485205687335000135, 1517.181921232829836, 216.8478361320569832 ) ) ;
#26515=CARTESIAN_POINT ( 'NONE',  ( 4.995994787574999485, 1516.665179208830068, 206.6322283937570035 ) ) ;
#26520=CARTESIAN_POINT ( 'NONE',  ( -5.513243736250649896, 1508.551565959790196, 201.9548213322269987 ) ) ;
#26534=CARTESIAN_POINT ( 'NONE',  ( 4.620008207075000151, 1516.777260590120022, 214.8964555921769772 ) ) ;
#26540=CARTESIAN_POINT ( 'NONE',  ( 2.494020282435000180, 1516.876240617270014, 211.4047611534970201 ) ) ;
#26558=CARTESIAN_POINT ( 'NONE',  ( -0.7560907659159991079, 1516.770163853809890, 204.1215159365669933 ) ) ;
#26591=ORIENTED_EDGE ( 'NONE', *, *, #55688, .F. ) ;
#26635=CARTESIAN_POINT ( 'NONE',  ( -5.773668852974999766, 1516.734985836460055, 213.1604834329569940 ) ) ;
#26640=CARTESIAN_POINT ( 'NONE',  ( 6.937965660314999283, 1516.732530461250008, 204.1161457306970135 ) ) ;
#26651=CARTESIAN_POINT ( 'NONE',  ( -0.4403324739431219714, 1517.051704035390003, 216.6089087266339845 ) ) ;
#26653=CARTESIAN_POINT ( 'NONE',  ( 2.492443650904999863, 1516.793978928989873, 212.3737347995770222 ) ) ;
#26658=CARTESIAN_POINT ( 'NONE',  ( -2.493697079054999932, 1516.977201124959947, 208.0034927161370035 ) ) ;
#26675=CARTESIAN_POINT ( 'NONE',  ( -2.869693497065000098, 1517.070197312179971, 214.9093229647470196 ) ) ;
#26680=CARTESIAN_POINT ( 'NONE',  ( 2.872836622524999939, 1517.158319634930194, 201.3964737998670103 ) ) ;
#26687=CARTESIAN_POINT ( 'NONE',  ( 8.720950440807788695, 1511.461696079649982, 203.5356427006819899 ) ) ;
#26708=CARTESIAN_POINT ( 'NONE',  ( 9.638115859579080791, 1516.551188146539971, 214.4931927712729873 ) ) ;
#26718=CARTESIAN_POINT ( 'NONE',  ( -1.336491736407680042, 1516.593294715569982, 201.4112694980950096 ) ) ;
#26725=EDGE_CURVE ( 'NONE', #63057, #37652, #107867, .T. ) ;
#26728=ORIENTED_EDGE ( 'NONE', *, *, #21887, .F. ) ;
#26751=CARTESIAN_POINT ( 'NONE',  ( -1.906499846882070084E-08, 1517.051704408389924, 209.1218459511669892 ) ) ;
#26769=CARTESIAN_POINT ( 'NONE',  ( 5.788691325514999875, 1517.157901477309906, 210.2449475486469908 ) ) ;
#26778=CARTESIAN_POINT ( 'NONE',  ( -14.98757063811820167, 1513.799047786500068, 223.8171003904659813 ) ) ;
#26785=CARTESIAN_POINT ( 'NONE',  ( -3.267039729984999585, 1517.012231669750008, 208.3862772893259887 ) ) ;
#26787=CARTESIAN_POINT ( 'NONE',  ( -6.036759191025518057, 1509.035273823006037, 216.5824821671302800 ) ) ;
#26802=CARTESIAN_POINT ( 'NONE',  ( 3.253141137235000091, 1516.858171774179937, 205.8542424163969997 ) ) ;
#26805=CARTESIAN_POINT ( 'NONE',  ( -3.879787126964284294, 1516.685805519419546, 202.7020868552936292 ) ) ;
#26825=CARTESIAN_POINT ( 'NONE',  ( 1.133516965105000107, 1516.713079096360161, 213.7319258036569920 ) ) ;
#26832=( BOUNDED_CURVE ( )  B_SPLINE_CURVE ( 3, ( #101446, #108219, #41581, #6316 ),
 .UNSPECIFIED., .F., .F. ) 
 B_SPLINE_CURVE_WITH_KNOTS ( ( 4, 4 ),
 ( 2.354951092798057921, 3.925058725375623947 ),
 .UNSPECIFIED. ) 
 CURVE ( )  GEOMETRIC_REPRESENTATION_ITEM ( )  RATIONAL_B_SPLINE_CURVE ( ( 1.000000000000000000, 0.8049001529565240620, 0.8049001529565240620, 1.000000000000000000 ) ) 
 REPRESENTATION_ITEM ( '' )  );
#26856=CARTESIAN_POINT ( 'NONE',  ( 1.135185044044999980, 1516.778853242349896, 212.5689744308569971 ) ) ;
#26898=CARTESIAN_POINT ( 'NONE',  ( -7.042712267680692584, 1516.564738270622684, 211.7005065504913262 ) ) ;
#26903=CARTESIAN_POINT ( 'NONE',  ( 6.546039395294999785, 1516.565291103010168, 206.8289057630870218 ) ) ;
#26916=CARTESIAN_POINT ( 'NONE',  ( -0.7355686809059980291, 1517.012231669750008, 212.3888856620870058 ) ) ;
#26918=VECTOR ( 'NONE', #899, 1000.000000000000114 ) ;
#26936=VECTOR ( 'NONE', #7757, 1000.000000000000000 ) ;
#26940=CARTESIAN_POINT ( 'NONE',  ( 6.769661272017690301, 1509.032013615249980, 201.8557649540310024 ) ) ;
#26945=CARTESIAN_POINT ( 'NONE',  ( -7.331812124104999384, 1516.906641539930206, 202.5676945058570197 ) ) ;
#26946=CARTESIAN_POINT ( 'NONE',  ( 4.623892060624999800, 1517.066898074209803, 209.8584071487349831 ) ) ;
#26987=CARTESIAN_POINT ( 'NONE',  ( -15.37702286096500082, 1512.655881406860090, 222.6262963000669970 ) ) ;
#26991=CARTESIAN_POINT ( 'NONE',  ( 5.770883563884999568, 1516.603620185149794, 206.8276363026970159 ) ) ;
#27008=CARTESIAN_POINT ( 'NONE',  ( -2.475398974845000044, 1511.813148765560072, 201.5364415457169969 ) ) ;
#27034=CARTESIAN_POINT ( 'NONE',  ( -5.984345136421869604, 1508.551704613440052, 216.1343701918329998 ) ) ;
#27046=CARTESIAN_POINT ( 'NONE',  ( -2.877113108595000135, 1516.697242742309982, 204.1252037719370094 ) ) ;
#27048=CARTESIAN_POINT ( 'NONE',  ( 16.11449818973499859, 1514.335759350750095, 194.1182033692670075 ) ) ;
#27059=ORIENTED_EDGE ( 'NONE', *, *, #56436, .T. ) ;
#27071=CARTESIAN_POINT ( 'NONE',  ( -7.708770045145000083, 1516.524310051880093, 211.4128934593470035 ) ) ;
#27075=CARTESIAN_POINT ( 'NONE',  ( 6.242053746214999421, 1513.743447518349967, 201.5518632705069706 ) ) ;
#27084=CARTESIAN_POINT ( 'NONE',  ( -7.329930051325000306, 1516.881930554049859, 216.8399805996670011 ) ) ;
#27086=VECTOR ( 'NONE', #38514, 1000.000000000000000 ) ;
#27092=CARTESIAN_POINT ( 'NONE',  ( 4.996642160164999957, 1516.697242742309982, 206.2447328616370044 ) ) ;
#27097=CARTESIAN_POINT ( 'NONE',  ( -7.320053526199809646, 1508.610509074409947, 203.0404548948610000 ) ) ;
#27107=CARTESIAN_POINT ( 'NONE',  ( -3.257220640824999958, 1517.040132827679827, 214.9086836491569841 ) ) ;
#27109=CARTESIAN_POINT ( 'NONE',  ( 5.652025608424629866, 1510.855104182140167, 216.7229383695649858 ) ) ;
#27111=CARTESIAN_POINT ( 'NONE',  ( 1.715704490974999885, 1516.757508073510053, 212.3732403323669757 ) ) ;
#27128=CARTESIAN_POINT ( 'NONE',  ( -4.038637500854999729, 1516.734985836460055, 203.3481771172569950 ) ) ;
#27157=( BOUNDED_CURVE ( )  B_SPLINE_CURVE ( 3, ( #60098, #42730, #61225, #110478 ),
 .UNSPECIFIED., .F., .F. ) 
 B_SPLINE_CURVE_WITH_KNOTS ( ( 4, 4 ),
 ( 4.286339096376821090, 4.712350959133279282 ),
 .UNSPECIFIED. ) 
 CURVE ( )  GEOMETRIC_REPRESENTATION_ITEM ( )  RATIONAL_B_SPLINE_CURVE ( ( 1.000000000000000000, 0.9849332539716901813, 0.9849332539716901813, 1.000000000000000000 ) ) 
 REPRESENTATION_ITEM ( '' )  );
#27177=CARTESIAN_POINT ( 'NONE',  ( -4.490619237334504632, 1508.909942010301620, 205.6342535026303437 ) ) ;
#27181=CARTESIAN_POINT ( 'NONE',  ( 7.513187920566976707, 1510.663752934522563, 203.1583860890702908 ) ) ;
#27202=CARTESIAN_POINT ( 'NONE',  ( -4.610938249504999753, 1516.815231249920089, 213.1623732742069990 ) ) ;
#27203=CARTESIAN_POINT ( 'NONE',  ( 2.930838039564999775, 1510.983859056260144, 216.6855341620170350 ) ) ;
#27207=CARTESIAN_POINT ( 'NONE',  ( -2.295485539174999978, 1516.651306816259876, 204.1261199623870368 ) ) ;
#27219=PLANE ( 'NONE',  #49681 ) ;
#27222=CARTESIAN_POINT ( 'NONE',  ( 6.949574947644999945, 1517.102359858469754, 212.3809477691169718 ) ) ;
#27228=CARTESIAN_POINT ( 'NONE',  ( -0.7533003905399979772, 1516.992029636990083, 208.3816250717139837 ) ) ;
#27229=ORIENTED_EDGE ( 'NONE', *, *, #3822, .T. ) ;
#27242=CARTESIAN_POINT ( 'NONE',  ( 6.944231748164999551, 1516.882690742909972, 215.6753703478370028 ) ) ;
#27245=CARTESIAN_POINT ( 'NONE',  ( -7.329930051325000306, 1516.881930554049859, 216.8399805996670011 ) ) ;
#27247=CARTESIAN_POINT ( 'NONE',  ( 7.329930013194999816, 1516.881930554049859, 201.4037113026670056 ) ) ;
#27252=CARTESIAN_POINT ( 'NONE',  ( 7.444284895405609781, 1510.876154134890157, 202.8741411524250111 ) ) ;
#27260=CARTESIAN_POINT ( 'NONE',  ( 7.012921545624998920, 1508.551704408389924, 214.6352815241970120 ) ) ;
#27312=CARTESIAN_POINT ( 'NONE',  ( -6.554764199473687825, 1516.786099426707551, 201.4062207776168236 ) ) ;
#27318=ORIENTED_EDGE ( 'NONE', *, *, #103453, .F. ) ;
#27321=CARTESIAN_POINT ( 'NONE',  ( 1.717139084115000047, 1516.949031626070109, 210.2396860569670025 ) ) ;
#27333=ORIENTED_EDGE ( 'NONE', *, *, #63222, .F. ) ;
#27335=CARTESIAN_POINT ( 'NONE',  ( -0.01012492377659850000, 1516.989863902050047, 207.9939175986969815 ) ) ;
#27352=CARTESIAN_POINT ( 'NONE',  ( 5.771797426184999580, 1516.647618671360078, 206.2459958378869942 ) ) ;
#27355=CARTESIAN_POINT ( 'NONE',  ( -3.644878300669852855, 1516.661627594551419, 202.5664891927213489 ) ) ;
#27359=EDGE_CURVE ( 'NONE', #38027, #17126, #29139, .T. ) ;
#27361=ADVANCED_FACE ( 'NONE', ( #100837 ), #67283, .T. ) ;
#27373=CARTESIAN_POINT ( 'NONE',  ( 1.713317409674999903, 1516.660388280709867, 213.7298676393670291 ) ) ;
#27399=CARTESIAN_POINT ( 'NONE',  ( 3.459156578084999989, 1516.769879638719885, 213.7318425517769924 ) ) ;
#27440=CARTESIAN_POINT ( 'NONE',  ( -8.652776130911478347, 1511.435001053830092, 214.5073691320910143 ) ) ;
#27443=CARTESIAN_POINT ( 'NONE',  ( -0.7579844201469989606, 1516.883361325900069, 206.8353730456769881 ) ) ;
#27455=CARTESIAN_POINT ( 'NONE',  ( 6.561995960394999550, 1517.083030555940013, 212.3803205491769859 ) ) ;
#27475=CARTESIAN_POINT ( 'NONE',  ( 5.513199790315740145, 1509.038617475689989, 201.6090956973179971 ) ) ;
#27476=EDGE_CURVE ( 'NONE', #71414, #64503, #17995, .T. ) ;
#27478=EDGE_CURVE ( 'NONE', #94274, #22497, #86027, .T. ) ;
#27483=CARTESIAN_POINT ( 'NONE',  ( -5.006329619514999330, 1516.755758396839838, 202.5714564999769891 ) ) ;
#27484=CARTESIAN_POINT ( 'NONE',  ( -0.7374509209069979310, 1516.978425811520083, 210.2554991112269818 ) ) ;
#27499=LINE ( 'NONE', #44322, #90654 ) ;
#27512=CARTESIAN_POINT ( 'NONE',  ( -5.649719788644999241, 1514.243099272629934, 216.7708803706970002 ) ) ;
#27519=ORIENTED_EDGE ( 'NONE', *, *, #108317, .T. ) ;
#27523=DIRECTION ( 'NONE',  ( -0.06162841671618445039, -0.9961946980917499861, 0.06162841671618458916 ) ) ;
#27529=DIRECTION ( 'NONE',  ( 0.001619481661242269796, -0.06184550950381718926, -0.9980844203940678616 ) ) ;
#27535=CARTESIAN_POINT ( 'NONE',  ( 2.477373605864999995, 1516.891731298979948, 206.2406231745169976 ) ) ;
#27587=CARTESIAN_POINT ( 'NONE',  ( 6.549762446985000430, 1516.729202374750002, 204.5030968636170030 ) ) ;
#27611=CARTESIAN_POINT ( 'NONE',  ( -2.865588722415000067, 1516.890356958860139, 212.3900816908670208 ) ) ;
#27617=EDGE_CURVE ( 'NONE', #89576, #29868, #9711, .T. ) ;
#27631=ORIENTED_EDGE ( 'NONE', *, *, #31043, .T. ) ;
#27632=CARTESIAN_POINT ( 'NONE',  ( -4.044321718124999521, 1517.001127920769704, 206.8363583507369867 ) ) ;
#27633=VERTEX_POINT ( 'NONE', #78021 ) ;
#27651=CARTESIAN_POINT ( 'NONE',  ( 0.7553264358530019651, 1516.745833913490060, 214.8974710475970085 ) ) ;
#27654=CARTESIAN_POINT ( 'NONE',  ( 5.424122834273520155, 1511.219705715099963, 216.9885700916489952 ) ) ;
#27656=CARTESIAN_POINT ( 'NONE',  ( -4.028307778284999863, 1516.797038924770050, 212.3881954442970255 ) ) ;
#27674=CARTESIAN_POINT ( 'NONE',  ( 6.550389432124999800, 1516.755758396839838, 204.1155163507169732 ) ) ;
#27714=CARTESIAN_POINT ( 'NONE',  ( -1.906499758064230099E-08, 1508.551704408389924, 216.1347675157070114 ) ) ;
#27716=CARTESIAN_POINT ( 'NONE',  ( 2.485205649205000089, 1517.181921232829836, 201.3958557702769951 ) ) ;
#27724=CARTESIAN_POINT ( 'NONE',  ( -4.545982247914895247, 1508.783371651612924, 205.6342535022036202 ) ) ;
#27730=CARTESIAN_POINT ( 'NONE',  ( -7.703229056714999246, 1511.126521646420088, 214.5635183388470182 ) ) ;
#27746=CARTESIAN_POINT ( 'NONE',  ( -2.287084308194999860, 1517.068517094990057, 214.1351209316169957 ) ) ;
#27747=CARTESIAN_POINT ( 'NONE',  ( 3.611462603544999705, 1511.572472350439739, 217.1939399984370027 ) ) ;
#27753=CARTESIAN_POINT ( 'NONE',  ( 6.551643386774999023, 1516.807958722750072, 203.3403553877570005 ) ) ;
#27769=CARTESIAN_POINT ( 'NONE',  ( 4.624099291334999862, 1516.962555622980062, 212.3771868965270073 ) ) ;
#27773=CARTESIAN_POINT ( 'NONE',  ( 4.987078422726499483, 1508.551704408389924, 205.6342535031670025 ) ) ;
#27776=CARTESIAN_POINT ( 'NONE',  ( -5.781585816274999345, 1516.939646076049939, 209.1342929058909874 ) ) ;
#27779=CARTESIAN_POINT ( 'NONE',  ( -7.717505791104999346, 1516.857914730730045, 201.4043401791270185 ) ) ;
#27792=CARTESIAN_POINT ( 'NONE',  ( -6.940473372275000052, 1516.833525648419936, 215.6778681647369922 ) ) ;
#27797=FACE_OUTER_BOUND ( 'NONE', #87106, .T. ) ;
#27802=CARTESIAN_POINT ( 'NONE',  ( 15.90990511613090241, 1514.921193439799936, 193.9190475034619965 ) ) ;
#27806=CARTESIAN_POINT ( 'NONE',  ( 8.379224430868440265, 1511.478393686179970, 203.5654043840270049 ) ) ;
#27836=CARTESIAN_POINT ( 'NONE',  ( -1.747411913067469902, 1516.543067334039961, 201.4125847483680047 ) ) ;
#27843=VERTEX_POINT ( 'NONE', #89727 ) ;
#27869=CARTESIAN_POINT ( 'NONE',  ( -3.801734883709992019, 1509.034509900240437, 213.6092049266663651 ) ) ;
#27880=CARTESIAN_POINT ( 'NONE',  ( -3.253301419385000504, 1516.790374942449944, 210.2573062871869922 ) ) ;
#27882=CARTESIAN_POINT ( 'NONE',  ( -15.55634920516500053, 1516.551704408390151, 193.5654967650670244 ) ) ;
#27895=CARTESIAN_POINT ( 'NONE',  ( 7.323390407215000231, 1516.613712827999962, 207.9924597298270044 ) ) ;
#27913=CARTESIAN_POINT ( 'NONE',  ( -7.725990199955000470, 1517.181921232829836, 206.6366402828969910 ) ) ;
#27915=LINE ( 'NONE', #61538, #72284 ) ;
#27918=CARTESIAN_POINT ( 'NONE',  ( 4.858360384088095785, 1508.551704408384467, 212.6094383991669758 ) ) ;
#27923=DIRECTION ( 'NONE',  ( 0.5224574779879248565, 0.7067418228238977473, -0.4770263929449307105 ) ) ;
#27931=CARTESIAN_POINT ( 'NONE',  ( 6.559798056295000457, 1516.987478262539980, 213.7368632980669929 ) ) ;
#27999=CARTESIAN_POINT ( 'NONE',  ( -6.563595907815000352, 1517.154223579619838, 206.8322214998769937 ) ) ;
#28001=CARTESIAN_POINT ( 'NONE',  ( -7.012921583638330070, 1508.551704408389924, 203.6084103760139783 ) ) ;
#28009=CARTESIAN_POINT ( 'NONE',  ( -3.446329813785000251, 1516.812046502680005, 212.0014881234369852 ) ) ;
#28031=CARTESIAN_POINT ( 'NONE',  ( 5.513258746607349714, 1508.551704615640119, 202.1093796504439979 ) ) ;
#28036=CARTESIAN_POINT ( 'NONE',  ( 3.258474578945000033, 1517.083030555940013, 202.5598499717069956 ) ) ;
#28037=CARTESIAN_POINT ( 'NONE',  ( -1.701850495234999983, 1516.908147884120126, 210.2591426210370003 ) ) ;
#28038=ORIENTED_EDGE ( 'NONE', *, *, #21447, .T. ) ;
#28042=CARTESIAN_POINT ( 'NONE',  ( 4.364191681395142908, 1509.032014410904821, 213.2377288302579359 ) ) ;
#28058=CARTESIAN_POINT ( 'NONE',  ( -7.653848905685000759, 1514.071098020770023, 202.5580345204870127 ) ) ;
#28074=CARTESIAN_POINT ( 'NONE',  ( 14.83035613263499997, 1514.570049710740022, 225.4041969180670151 ) ) ;
#28083=CARTESIAN_POINT ( 'NONE',  ( -0.7578858299649979813, 1516.872851364150165, 206.6414186775969881 ) ) ;
#28101=CARTESIAN_POINT ( 'NONE',  ( 4.590060377064090424, 1517.051704403100075, 201.3992656192910147 ) ) ;
#28118=EDGE_CURVE ( 'NONE', #78578, #54193, #51037, .T. ) ;
#28120=EDGE_CURVE ( 'NONE', #29671, #68939, #103065, .T. ) ;
#28136=AXIS2_PLACEMENT_3D ( 'NONE', #32495, #85081, #110292 ) ;
#28138=CARTESIAN_POINT ( 'NONE',  ( -0.01289782690309849988, 1516.939723362869927, 204.1155860834069813 ) ) ;
#28160=CARTESIAN_POINT ( 'NONE',  ( 3.267603515704999850, 1516.858171774179937, 212.3749871074670068 ) ) ;
#28172=CARTESIAN_POINT ( 'NONE',  ( -8.640072926265000675, 1511.773927532309926, 215.2821261476370012 ) ) ;
#28173=CARTESIAN_POINT ( 'NONE',  ( 16.78766063793228014, 1513.436209039135292, 196.1310004108296141 ) ) ;
#28183=CARTESIAN_POINT ( 'NONE',  ( -5.013274999515000552, 1517.068517094990057, 206.8347616620369820 ) ) ;
#28188=CARTESIAN_POINT ( 'NONE',  ( -7.167024603737270461, 1508.551565959610116, 203.6086025299220239 ) ) ;
#28201=CARTESIAN_POINT ( 'NONE',  ( 2.292307230374999616, 1516.548716157039962, 216.0554627912370051 ) ) ;
#28203=CARTESIAN_POINT ( 'NONE',  ( 5.469699236675529264, 1510.954290761809943, 216.7857353825710049 ) ) ;
#28205=CARTESIAN_POINT ( 'NONE',  ( 4.624099291334999862, 1516.962555622980062, 212.3771868965270073 ) ) ;
#28223=CARTESIAN_POINT ( 'NONE',  ( 1.121950743945000051, 1517.123342927159911, 204.1084165760470057 ) ) ;
#28240=ORIENTED_EDGE ( 'NONE', *, *, #61786, .F. ) ;
#28252=ADVANCED_FACE ( 'NONE', ( #91239 ), #96589, .T. ) ;
#28267=CARTESIAN_POINT ( 'NONE',  ( 1.126138108584999964, 1517.208444099459939, 201.3951612445669923 ) ) ;
#28272=CARTESIAN_POINT ( 'NONE',  ( 7.589847736954999924, 1511.982868782460173, 206.7094295734470109 ) ) ;
#28304=CARTESIAN_POINT ( 'NONE',  ( -7.713117841115000317, 1516.690345681169902, 214.1262880092169780 ) ) ;
#28305=CARTESIAN_POINT ( 'NONE',  ( 2.711770194995000161, 1512.058324472099912, 216.8053402088569896 ) ) ;
#28314=CARTESIAN_POINT ( 'NONE',  ( 2.479246847704999812, 1516.983612918759945, 205.0778556245070092 ) ) ;
#28320=ORIENTED_EDGE ( 'NONE', *, *, #69240, .T. ) ;
#28327=CARTESIAN_POINT ( 'NONE',  ( -6.546302780145000000, 1516.577434278289957, 211.6089493897669911 ) ) ;
#28332=CARTESIAN_POINT ( 'NONE',  ( -0.7402208985179988820, 1516.992029636990083, 209.8751463226419958 ) ) ;
#28346=CARTESIAN_POINT ( 'NONE',  ( -4.032397940005000514, 1516.981965530290154, 214.9074288837770155 ) ) ;
#28347=CARTESIAN_POINT ( 'NONE',  ( -7.708815826551380646, 1516.526058373149908, 211.4663580544020078 ) ) ;
#28364=LINE ( 'NONE', #20487, #37416 ) ;
#28385=CARTESIAN_POINT ( 'NONE',  ( 15.55634916703500004, 1516.551704408390151, 224.6781951372670108 ) ) ;
#28420=DIRECTION ( 'NONE',  ( 0.000000000000000000, -1.000000000000000000, 6.123233995736769734E-17 ) ) ;
#28431=CARTESIAN_POINT ( 'NONE',  ( -1.119592219845000125, 1516.958737650239982, 210.2577447559170025 ) ) ;
#28439=ORIENTED_EDGE ( 'NONE', *, *, #17844, .T. ) ;
#28442=CARTESIAN_POINT ( 'NONE',  ( 2.872836622524999939, 1517.158319634930194, 201.3964737998670103 ) ) ;
#28449=CARTESIAN_POINT ( 'NONE',  ( 2.480427254505000345, 1516.872851364150165, 208.3639601402670110 ) ) ;
#28467=CARTESIAN_POINT ( 'NONE',  ( -2.299014068865000038, 1516.811292230880099, 206.2578025137869986 ) ) ;
#28474=B_SPLINE_CURVE_WITH_KNOTS ( 'NONE', 3,
 ( #67867, #75706, #94136, #100872, #85738, #43751, #24706, #103078, #9036, #52164, #33130, #34790, #17407, #101978, #86295, #68977, #24164, #76247, #93035, #77357, #16308, #33675, #25264, #50510, #115, #41550, #60574, #26379, #7386, #659, #51604, #58354, #25817, #110395, #94694, #9579, #109311, #32596, #92478, #59466, #15748, #84087, #109853, #67318, #93576, #16851, #53836, #11796, #71183 ),
 .UNSPECIFIED., .F., .F.,
 ( 4, 2, 1, 2, 2, 2, 1, 1, 2, 2, 2, 2, 1, 1, 1, 2, 2, 2, 2, 1, 1, 1, 2, 2, 2, 1, 1, 2, 2, 4 ),
 ( 0.000000000000000000, 0.06249999999985297872, 0.09374999999977946807, 0.1093749999998712974, 0.1249999999999631406, 0.1874999999995866362, 0.2187499999993044175, 0.2343749999991634470, 0.2421874999990958899, 0.2499999999990283328, 0.3749999999982073229, 0.4374999999977968179, 0.4687499999975917042, 0.4843749999974626963, 0.4921874999973949727, 0.4960937499973809839, 0.4999999999973669396, 0.6249999999980714316, 0.6874999999984235943, 0.7187499999985956789, 0.7343749999986817212, 0.7421874999987244648, 0.7460937499987384536, 0.7499999999987524424, 0.8124999999990795141, 0.8437499999992470467, 0.8593749999993267608, 0.8671874999993630651, 0.8749999999993993693, 1.000000000000000000 ),
 .UNSPECIFIED. ) ;
#28485=CARTESIAN_POINT ( 'NONE',  ( 0.7543881828220019292, 1516.727502608469877, 215.6727161143369926 ) ) ;
#28554=CARTESIAN_POINT ( 'NONE',  ( -4.625359562974999506, 1517.025470194390209, 206.6416589153869836 ) ) ;
#28574=ORIENTED_EDGE ( 'NONE', *, *, #74145, .T. ) ;
#28577=VERTEX_POINT ( 'NONE', #5452 ) ;
#28586=CARTESIAN_POINT ( 'NONE',  ( 7.166260505965389882, 1508.551565390810083, 203.0889814045920048 ) ) ;
#28592=CARTESIAN_POINT ( 'NONE',  ( -0.01289782690309849988, 1516.939723362869927, 204.1155860834069813 ) ) ;
#28596=CARTESIAN_POINT ( 'NONE',  ( 5.513435558552499671, 1508.783371651585412, 201.6678281800477350 ) ) ;
#28616=CARTESIAN_POINT ( 'NONE',  ( -7.869279002454999450, 1514.500328598799797, 202.7397161129169945 ) ) ;
#28631=CARTESIAN_POINT ( 'NONE',  ( 14.74158144963499950, 1513.636261293280086, 225.1273934092670288 ) ) ;
#28640=CARTESIAN_POINT ( 'NONE',  ( 6.546001350565000543, 1516.557392317769882, 207.4118413833070065 ) ) ;
#28661=CARTESIAN_POINT ( 'NONE',  ( -2.892503416934999905, 1511.980236064749988, 201.3440512220070104 ) ) ;
#28697=CARTESIAN_POINT ( 'NONE',  ( 2.868433798504999910, 1517.020727862619879, 204.1095288638669842 ) ) ;
#28704=ORIENTED_EDGE ( 'NONE', *, *, #29001, .T. ) ;
#28712=PLANE ( 'NONE',  #45447 ) ;
#28716=CARTESIAN_POINT ( 'NONE',  ( 4.042417777704999438, 1516.904492006980036, 212.5700528489170154 ) ) ;
#28724=ORIENTED_EDGE ( 'NONE', *, *, #52443, .F. ) ;
#28725=ORIENTED_EDGE ( 'NONE', *, *, #73545, .T. ) ;
#28726=CARTESIAN_POINT ( 'NONE',  ( -8.308248955145000281, 1512.693483295319993, 216.2230634388170074 ) ) ;
#28738=CARTESIAN_POINT ( 'NONE',  ( -6.563254928984999736, 1517.139039350860003, 206.6385234782069915 ) ) ;
#28750=CARTESIAN_POINT ( 'NONE',  ( -6.044713241076149934, 1511.753217516670247, 200.8247887982400073 ) ) ;
#28751=CARTESIAN_POINT ( 'NONE',  ( 15.24750708283499989, 1514.857962383129916, 194.6708682431670070 ) ) ;
#28756=CARTESIAN_POINT ( 'NONE',  ( -5.003220765204999587, 1516.983995446890049, 216.0685944891870065 ) ) ;
#28758=CARTESIAN_POINT ( 'NONE',  ( 5.395039045001690070, 1511.384172056590160, 217.2813686725590117 ) ) ;
#28760=CARTESIAN_POINT ( 'NONE',  ( -6.546951720715000533, 1516.606339319019980, 211.9964348928969855 ) ) ;
#28764=CARTESIAN_POINT ( 'NONE',  ( 3.822978225239960004, 1508.729442836390035, 213.6787569587939970 ) ) ;
#28781=CARTESIAN_POINT ( 'NONE',  ( -2.491188396525000126, 1516.733363207009916, 205.0947945262969938 ) ) ;
#28798=EDGE_CURVE ( 'NONE', #27843, #85013, #93860, .T. ) ;
#28812=( BOUNDED_CURVE ( )  B_SPLINE_CURVE ( 3, ( #26087, #94973, #86563, #42354 ),
 .UNSPECIFIED., .F., .F. ) 
 B_SPLINE_CURVE_WITH_KNOTS ( ( 4, 4 ),
 ( 1.282864256331062158, 2.438226007407914953 ),
 .UNSPECIFIED. ) 
 CURVE ( )  GEOMETRIC_REPRESENTATION_ITEM ( )  RATIONAL_B_SPLINE_CURVE ( ( 1.000000000000000000, 0.8918208900698291197, 0.8918208900698291197, 1.000000000000000000 ) ) 
 REPRESENTATION_ITEM ( '' )  );
#28818=EDGE_CURVE ( 'NONE', #10547, #97701, #38251, .T. ) ;
#28823=CARTESIAN_POINT ( 'NONE',  ( -13.51662157586499902, 1512.620989416249813, 192.6780328270669997 ) ) ;
#28826=CARTESIAN_POINT ( 'NONE',  ( 7.717505752974999744, 1516.857914730730045, 201.4043401791270185 ) ) ;
#28862=CARTESIAN_POINT ( 'NONE',  ( 2.294209629405000062, 1516.603620185149794, 214.8927295341169952 ) ) ;
#28863=CARTESIAN_POINT ( 'NONE',  ( 2.950959321895000098, 1512.115618635729788, 217.0053894627469901 ) ) ;
#28870=CARTESIAN_POINT ( 'NONE',  ( -1.134358008724999811, 1516.744381837270112, 205.0932347109869909 ) ) ;
#28875=ORIENTED_EDGE ( 'NONE', *, *, #89043, .T. ) ;
#28882=CARTESIAN_POINT ( 'NONE',  ( 7.336844642415000450, 1517.106845464700200, 212.5753907958570039 ) ) ;
#28888=CARTESIAN_POINT ( 'NONE',  ( -2.873919040654999701, 1516.940252185109784, 209.1351185066319829 ) ) ;
#28894=ORIENTED_EDGE ( 'NONE', *, *, #17134, .F. ) ;
#28899=CARTESIAN_POINT ( 'NONE',  ( 7.552141914295000369, 1510.542924508009946, 205.3415595432570058 ) ) ;
#28903=CARTESIAN_POINT ( 'NONE',  ( -7.715625241105000143, 1516.786099423779888, 215.6766101314970001 ) ) ;
#28904=CARTESIAN_POINT ( 'NONE',  ( -7.812463265990185590, 1516.551704358176721, 211.9845609180970030 ) ) ;
#28910=ORIENTED_EDGE ( 'NONE', *, *, #110424, .T. ) ;
#28911=AXIS2_PLACEMENT_3D ( 'NONE', #103940, #69260, #105052 ) ;
#28915=CARTESIAN_POINT ( 'NONE',  ( 8.247029077068420477, 1511.494703458840149, 203.4175148351339999 ) ) ;
#28948=ORIENTED_EDGE ( 'NONE', *, *, #28118, .T. ) ;
#28950=CARTESIAN_POINT ( 'NONE',  ( 13.27508835580430002, 1512.548660307860018, 224.4065169982920054 ) ) ;
#28972=ORIENTED_EDGE ( 'NONE', *, *, #8680, .F. ) ;
#28989=CARTESIAN_POINT ( 'NONE',  ( -2.863787893864999656, 1516.788317650260069, 210.8382387120070121 ) ) ;
#28997=FACE_OUTER_BOUND ( 'NONE', #48554, .T. ) ;
#28999=CARTESIAN_POINT ( 'NONE',  ( 4.616272296565000488, 1517.030858226499959, 201.7868885755270014 ) ) ;
#29001=EDGE_CURVE ( 'NONE', #55385, #3290, #101004, .T. ) ;
#29008=ADVANCED_FACE ( 'NONE', ( #76937 ), #42777, .T. ) ;
#29011=ORIENTED_EDGE ( 'NONE', *, *, #6667, .T. ) ;
#29014=CARTESIAN_POINT ( 'NONE',  ( 8.788316489185000080, 1511.741868877540128, 202.8695794779170001 ) ) ;
#29022=CARTESIAN_POINT ( 'NONE',  ( -1.717084749545000122, 1516.819260244609950, 206.6456753351970121 ) ) ;
#29040=CARTESIAN_POINT ( 'NONE',  ( 7.333070134885000257, 1516.955859323880077, 214.9008457440070003 ) ) ;
#29047=CARTESIAN_POINT ( 'NONE',  ( 3.793219999985080193, 1517.051709179919953, 202.4207530290020145 ) ) ;
#29072=CARTESIAN_POINT ( 'NONE',  ( 15.17646693133499980, 1516.904916668740043, 193.1856145293670011 ) ) ;
#29073=ORIENTED_EDGE ( 'NONE', *, *, #22093, .F. ) ;
#29094=VERTEX_POINT ( 'NONE', #107082 ) ;
#29095=CARTESIAN_POINT ( 'NONE',  ( -6.827653043921440457, 1508.551704612109916, 215.5772713760989916 ) ) ;
#29105=CARTESIAN_POINT ( 'NONE',  ( 0.7352271172030020452, 1516.963431999339946, 207.4067364850470199 ) ) ;
#29125=CARTESIAN_POINT ( 'NONE',  ( 13.16131580973219428, 1513.520094851659223, 225.9095696691143473 ) ) ;
#29139=B_SPLINE_CURVE_WITH_KNOTS ( 'NONE', 3,
 ( #102492, #58316, #25782, #41512, #8435, #109815, #15715, #76211, #69, #77322, #83492, #24666, #84050, #110356, #85700, #25226, #40949, #8996, #92438, #24126, #32558, #43167, #34752, #109274, #7889, #59429, #92996, #94657, #34201, #60535, #26338, #59980, #33633, #42060, #94098, #68940, #101938, #16272, #49916, #103041, #16814, #75126, #51014, #17369, #50474, #49363, #84598, #7349, #6788, #66734 ),
 .UNSPECIFIED., .F., .F.,
 ( 4, 2, 2, 1, 1, 2, 2, 2, 2, 1, 1, 1, 2, 2, 2, 2, 1, 1, 1, 2, 2, 2, 2, 1, 1, 1, 1, 2, 2, 2, 4 ),
 ( 0.000000000000000000, 0.1249999999980411503, 0.1874999999970687059, 0.2187499999965762942, 0.2343749999963234409, 0.2421874999961906860, 0.2499999999960579311, 0.3749999999936606265, 0.4374999999924693017, 0.4687499999918546822, 0.4843749999915473725, 0.4921874999913936621, 0.4960937499913433690, 0.4999999999912930204, 0.6249999999905073711, 0.6874999999901078018, 0.7187499999898824266, 0.7343749999897392078, 0.7421874999897040137, 0.7460937499896861391, 0.7499999999896681535, 0.8124999999891825420, 0.8437499999888987690, 0.8593749999887184687, 0.8671874999885907931, 0.8710937499885216262, 0.8730468749884923163, 0.8740234374885097468, 0.8749999999885270663, 0.9374999999942634776, 1.000000000000000000 ),
 .UNSPECIFIED. ) ;
#29143=CARTESIAN_POINT ( 'NONE',  ( -7.720650173434999708, 1516.977993847330026, 203.3422188780170075 ) ) ;
#29149=EDGE_LOOP ( 'NONE', ( #14804, #48563, #62722, #61911 ) ) ;
#29165=CARTESIAN_POINT ( 'NONE',  ( -6.610870935635000833, 1511.929989569670170, 201.7390943842370064 ) ) ;
#29181=CARTESIAN_POINT ( 'NONE',  ( 12.73246619883500053, 1512.053076656670100, 224.9511024890669830 ) ) ;
#29189=CARTESIAN_POINT ( 'NONE',  ( 4.026614479655000522, 1516.699825673279975, 207.4075116849170115 ) ) ;
#29200=EDGE_CURVE ( 'NONE', #72956, #323, #59485, .T. ) ;
#29210=CARTESIAN_POINT ( 'NONE',  ( 6.187521057617754394, 1510.844697586414213, 216.5810360690583138 ) ) ;
#29226=DIRECTION ( 'NONE',  ( -0.7063774289747313251, 0.04540766091858271930, -0.7063774289747313251 ) ) ;
#29244=CARTESIAN_POINT ( 'NONE',  ( 3.449777315724999571, 1516.974592746400049, 204.1104779853070283 ) ) ;
#29262=CARTESIAN_POINT ( 'NONE',  ( -3.252530653725000054, 1516.827328999679821, 212.0018028951869837 ) ) ;
#29266=VERTEX_POINT ( 'NONE', #33663 ) ;
#29272=CARTESIAN_POINT ( 'NONE',  ( -6.402238504554999210, 1513.914017980350081, 216.7093358650170103 ) ) ;
#29273=CARTESIAN_POINT ( 'NONE',  ( 15.90990511613090241, 1514.921193439799936, 193.9190475034619965 ) ) ;
#29283=CARTESIAN_POINT ( 'NONE',  ( -2.300729664794999962, 1516.923170579120097, 207.4211391557370234 ) ) ;
#29299=CARTESIAN_POINT ( 'NONE',  ( -1.124894088365000044, 1517.194816588360027, 216.0733631026070043 ) ) ;
#29301=CARTESIAN_POINT ( 'NONE',  ( 5.550449858616669729, 1510.476657126699820, 216.6722583594520017 ) ) ;
#29304=CARTESIAN_POINT ( 'NONE',  ( -7.709681306425000713, 1516.559109716219837, 211.9945464874270158 ) ) ;
#29305=CARTESIAN_POINT ( 'NONE',  ( 3.487592428934999766, 1509.038615934169911, 204.6345961781970004 ) ) ;
#29315=FACE_OUTER_BOUND ( 'NONE', #110053, .T. ) ;
#29321=CARTESIAN_POINT ( 'NONE',  ( 3.253462060665000433, 1516.874084700499907, 205.6604858388269861 ) ) ;
#29329=CARTESIAN_POINT ( 'NONE',  ( -8.788316527315000570, 1511.741868877540128, 215.3741124244170067 ) ) ;
#29339=CARTESIAN_POINT ( 'NONE',  ( -11.88255532981709450, 1513.001579509954126, 192.5822564612562928 ) ) ;
#29345=FACE_OUTER_BOUND ( 'NONE', #19616, .T. ) ;
#29355=CARTESIAN_POINT ( 'NONE',  ( -11.35635716866499934, 1512.376261820769969, 192.9173751460670303 ) ) ;
#29362=CARTESIAN_POINT ( 'NONE',  ( 7.572192850525000019, 1511.308638870219966, 206.5572121486769959 ) ) ;
#29372=CARTESIAN_POINT ( 'NONE',  ( -7.735039587165000619, 1511.353635254350138, 212.6038253893969738 ) ) ;
#29382=CYLINDRICAL_SURFACE ( 'NONE', #25023, 0.9999999999999982236 ) ;
#29390=CARTESIAN_POINT ( 'NONE',  ( -3.255967424474999650, 1516.989560013210166, 214.1335248082570217 ) ) ;
#29391=CARTESIAN_POINT ( 'NONE',  ( 2.689982558025000081, 1512.192993275409890, 216.8079459747669944 ) ) ;
#29397=CARTESIAN_POINT ( 'NONE',  ( 5.774609621945000271, 1516.777260590120022, 204.5018377250270021 ) ) ;
#29413=CARTESIAN_POINT ( 'NONE',  ( 2.491188358395000080, 1516.733363207009916, 213.1488973760370129 ) ) ;
#29419=CARTESIAN_POINT ( 'NONE',  ( -7.716977042262949560, 1516.837731796779963, 209.4547301039729632 ) ) ;
#29421=CARTESIAN_POINT ( 'NONE',  ( -1.704170752255000032, 1516.927039499179955, 209.8797722570040207 ) ) ;
#29425=CARTESIAN_POINT ( 'NONE',  ( -5.513435837193367384, 1508.551704405448163, 201.9544627215969115 ) ) ;
#29433=CARTESIAN_POINT ( 'NONE',  ( 3.958634245108940242, 1508.551704408389924, 214.1089244000060035 ) ) ;
#29435=CARTESIAN_POINT ( 'NONE',  ( -5.778372601744999670, 1516.932669162149978, 216.0673360190369863 ) ) ;
#29436=CARTESIAN_POINT ( 'NONE',  ( -8.002723402924999618, 1516.551704408390151, 212.1748218667169965 ) ) ;
#29440=CARTESIAN_POINT ( 'NONE',  ( -1.129386240404999908, 1516.613712827999962, 201.7984555248870038 ) ) ;
#29476=CARTESIAN_POINT ( 'NONE',  ( 0.3076635671722720011, 1517.019662593890189, 201.4001056456369838 ) ) ;
#29488=VECTOR ( 'NONE', #7782, 1000.000000000000000 ) ;
#29506=ADVANCED_FACE ( 'NONE', ( #9025 ), #102743, .F. ) ;
#29526=CARTESIAN_POINT ( 'NONE',  ( 2.299983577604999940, 1516.861367446839949, 211.4044688825970013 ) ) ;
#29535=CARTESIAN_POINT ( 'NONE',  ( 7.329303077985000137, 1516.857992118400034, 201.7912917986770083 ) ) ;
#29557=CARTESIAN_POINT ( 'NONE',  ( 1.118353215965000036, 1516.977201124959947, 206.6281488911770055 ) ) ;
#29572=CARTESIAN_POINT ( 'NONE',  ( 1.710004548794999968, 1516.557392317769882, 215.6678473207969944 ) ) ;
#29606=ORIENTED_EDGE ( 'NONE', *, *, #55366, .T. ) ;
#29620=CARTESIAN_POINT ( 'NONE',  ( 7.613520793314999757, 1512.886889331459997, 214.7360521135969975 ) ) ;
#29646=CARTESIAN_POINT ( 'NONE',  ( 7.710966977635000497, 1516.608208975040043, 207.9930883710269711 ) ) ;
#29668=CARTESIAN_POINT ( 'NONE',  ( 11.28282561095590175, 1512.859148089919017, 225.3214806919623356 ) ) ;
#29671=VERTEX_POINT ( 'NONE', #64288 ) ;
#29686=CARTESIAN_POINT ( 'NONE',  ( -2.489617576474999705, 1516.665179208830068, 204.1258511445269903 ) ) ;
#29699=CARTESIAN_POINT ( 'NONE',  ( 6.009430605671457926, 1511.590044791216769, 217.9119306497679531 ) ) ;
#29707=CARTESIAN_POINT ( 'NONE',  ( -7.378505853204999632, 1513.311928781849929, 201.4764924376770239 ) ) ;
#29708=VERTEX_POINT ( 'NONE', #45833 ) ;
#29722=CARTESIAN_POINT ( 'NONE',  ( 14.21596110103500088, 1513.125294087170005, 224.5826807846669908 ) ) ;
#29729=CARTESIAN_POINT ( 'NONE',  ( -2.881548462575000080, 1516.909589401870107, 206.8382752989369919 ) ) ;
#29763=CIRCLE ( 'NONE', #22618, 5.000000000000000000 ) ;
#29775=LINE ( 'NONE', #12963, #37640 ) ;
#29788=CARTESIAN_POINT ( 'NONE',  ( 1.120543697654999837, 1517.073005577650065, 205.0775260448770041 ) ) ;
#29803=CARTESIAN_POINT ( 'NONE',  ( 4.045182479925000685, 1517.057265928030120, 210.8256255754569963 ) ) ;
#29817=CARTESIAN_POINT ( 'NONE',  ( -6.534620482165000688, 1514.642928591849795, 217.2407288984570073 ) ) ;
#29831=CARTESIAN_POINT ( 'NONE',  ( 5.770883563884999568, 1516.603620185149794, 206.8276363026970159 ) ) ;
#29841=CARTESIAN_POINT ( 'NONE',  ( -5.382074274746489806, 1511.451532973539770, 200.6334450727659942 ) ) ;
#29848=CARTESIAN_POINT ( 'NONE',  ( -0.7391220051939990654, 1517.130100026000036, 216.0715493048870144 ) ) ;
#29849=DIRECTION ( 'NONE',  ( 0.001614312349211209771, 0.06164810140419219736, -0.9980966414074828874 ) ) ;
#29852=CARTESIAN_POINT ( 'NONE',  ( -6.935133418554999096, 1516.613881697390070, 212.3834819030570031 ) ) ;
#29868=VERTEX_POINT ( 'NONE', #79725 ) ;
#29869=CARTESIAN_POINT ( 'NONE',  ( 2.866857893004999713, 1516.951766529250108, 205.0784797119270024 ) ) ;
#29885=CARTESIAN_POINT ( 'NONE',  ( -10.96015512746500065, 1512.830284628050094, 193.2119433744669834 ) ) ;
#29890=CARTESIAN_POINT ( 'NONE',  ( 7.012921545474999796, 1508.551704408389924, 203.6084103740869864 ) ) ;
#29895=EDGE_LOOP ( 'NONE', ( #48884, #23275, #92060, #18731 ) ) ;
#29901=CARTESIAN_POINT ( 'NONE',  ( -11.74136611096500005, 1511.863761374039996, 193.2704433220669955 ) ) ;
#29904=CARTESIAN_POINT ( 'NONE',  ( 4.615644804385000022, 1517.009964551830080, 202.1744681489270192 ) ) ;
#29908=CARTESIAN_POINT ( 'NONE',  ( 14.72576938353500076, 1512.123542805230272, 196.9321265835669976 ) ) ;
#29909=CARTESIAN_POINT ( 'NONE',  ( 8.104522033453514851, 1514.095142040210703, 216.4523148511033526 ) ) ;
#29913=CARTESIAN_POINT ( 'NONE',  ( 4.429773585409299663, 1508.551704408389924, 204.3196163324640224 ) ) ;
#29915=ORIENTED_EDGE ( 'NONE', *, *, #50102, .F. ) ;
#29919=CARTESIAN_POINT ( 'NONE',  ( -4.035490750763682577, 1516.630499594219145, 201.4102953026068121 ) ) ;
#29928=( NAMED_UNIT ( * ) PLANE_ANGLE_UNIT ( ) SI_UNIT ( $, .RADIAN. ) );
#29933=DIRECTION ( 'NONE',  ( 0.02616798426500965835, -0.9993150019883683122, 0.02616798426500970692 ) ) ;
#29943=CARTESIAN_POINT ( 'NONE',  ( 5.007588646914999941, 1516.804776704140068, 214.8970827629769644 ) ) ;
#29951=CARTESIAN_POINT ( 'NONE',  ( 7.711550677984999602, 1516.630499592039996, 205.0863552195469879 ) ) ;
#29965=CARTESIAN_POINT ( 'NONE',  ( -3.446942109845000157, 1516.842852731759876, 212.3891375753969726 ) ) ;
#29971=CARTESIAN_POINT ( 'NONE',  ( -7.710576472136819959, 1516.593294715559978, 210.4583376685390022 ) ) ;
#29972=CARTESIAN_POINT ( 'NONE',  ( 4.037050997585000189, 1516.939819969850078, 209.1086255745840106 ) ) ;
#29981=CARTESIAN_POINT ( 'NONE',  ( 7.588802682105000308, 1511.942942747529969, 206.8630203803070060 ) ) ;
#29984=CARTESIAN_POINT ( 'NONE',  ( 5.005700201405000271, 1516.732530461250008, 216.0598116305469887 ) ) ;
#29990=CARTESIAN_POINT ( 'NONE',  ( 4.034280915654999689, 1517.049325831759916, 202.1735242262370207 ) ) ;
#29993=CARTESIAN_POINT ( 'NONE',  ( -15.00522600296500819, 1511.839858410419993, 221.0503446609671414 ) ) ;
#30006=VERTEX_POINT ( 'NONE', #10859 ) ;
#30007=PLANE ( 'NONE',  #24830 ) ;
#30025=CARTESIAN_POINT ( 'NONE',  ( 12.92498206718109977, 1512.351864386150055, 224.3146316424329711 ) ) ;
#30068=CARTESIAN_POINT ( 'NONE',  ( -5.772978316675000166, 1516.659138130710289, 210.2536427808470023 ) ) ;
#30071=CARTESIAN_POINT ( 'NONE',  ( -4.995994825704999975, 1516.665179208830068, 211.6114635085770033 ) ) ;
#30078=CARTESIAN_POINT ( 'NONE',  ( -6.555393155154999540, 1516.809497469189864, 201.7937966518470034 ) ) ;
#30092=CARTESIAN_POINT ( 'NONE',  ( 6.951517132375000685, 1517.194816588360027, 210.2467400204669730 ) ) ;
#30097=CARTESIAN_POINT ( 'NONE',  ( 8.213194853374998772, 1511.437978678640093, 205.0621741365669948 ) ) ;
#30099=CARTESIAN_POINT ( 'NONE',  ( 3.251888829344999898, 1516.793978928989873, 206.6294022811970024 ) ) ;
#30116=CARTESIAN_POINT ( 'NONE',  ( -3.451033427095000050, 1517.025653221279981, 214.9083735325669977 ) ) ;
#30118=CARTESIAN_POINT ( 'NONE',  ( 7.711293535545939548, 1516.620679718459996, 207.9351109995780007 ) ) ;
#30120=CARTESIAN_POINT ( 'NONE',  ( -4.329791528864999961, 1515.051704408389924, 209.1218459511669892 ) ) ;
#30136=ORIENTED_EDGE ( 'NONE', *, *, #84024, .T. ) ;
#30175=CARTESIAN_POINT ( 'NONE',  ( -7.512716754807339470, 1509.034509426269778, 215.2632450604789938 ) ) ;
#30186=CARTESIAN_POINT ( 'NONE',  ( -2.493697079054999932, 1516.977201124959947, 208.0034927161370035 ) ) ;
#30210=CARTESIAN_POINT ( 'NONE',  ( 13.86354611765113454, 1513.912053484252510, 225.8081837123426965 ) ) ;
#30217=ORIENTED_EDGE ( 'NONE', *, *, #2105, .T. ) ;
#30218=CARTESIAN_POINT ( 'NONE',  ( 4.987078429521930367, 1508.551704408389924, 205.6342618271569904 ) ) ;
#30226=CARTESIAN_POINT ( 'NONE',  ( -3.487585887351170033, 1508.611352722540005, 204.4436967865070187 ) ) ;
#30228=CARTESIAN_POINT ( 'NONE',  ( -0.7553264739829980146, 1516.745833913490060, 203.3462208547369983 ) ) ;
#30238=CARTESIAN_POINT ( 'NONE',  ( -12.29919906773779914, 1512.135905030570029, 194.2944855735010208 ) ) ;
#30250=CARTESIAN_POINT ( 'NONE',  ( -7.468172886755000128, 1513.423632355020118, 202.6515140566669970 ) ) ;
#30268=CARTESIAN_POINT ( 'NONE',  ( 14.69977922143499960, 1513.518111364920060, 224.7800584559669801 ) ) ;
#30269=CARTESIAN_POINT ( 'NONE',  ( -15.90990259576500065, 1516.551704408390151, 220.0820010595669771 ) ) ;
#30275=CARTESIAN_POINT ( 'NONE',  ( -2.299983615734999987, 1516.861367446839949, 206.8392230197369770 ) ) ;
#30279=CIRCLE ( 'NONE', #92864, 1.000004583512053902 ) ;
#30294=VERTEX_POINT ( 'NONE', #110409 ) ;
#30318=LINE ( 'NONE', #63419, #108785 ) ;
#30326=CARTESIAN_POINT ( 'NONE',  ( -2.937955147957567181, 1512.266405701426038, 201.2341433539613718 ) ) ;
#30333=CARTESIAN_POINT ( 'NONE',  ( -2.298048961635000165, 1516.764084769670262, 205.6764383981169715 ) ) ;
#30335=ORIENTED_EDGE ( 'NONE', *, *, #33693, .T. ) ;
#30347=CARTESIAN_POINT ( 'NONE',  ( 4.625789976465000564, 1517.104192383289956, 210.2432295619669844 ) ) ;
#30377=CARTESIAN_POINT ( 'NONE',  ( 0.7374508827770021036, 1516.978425811520083, 207.9881927911069965 ) ) ;
#30396=CARTESIAN_POINT ( 'NONE',  ( -4.034280953785000179, 1517.049325831759916, 216.0701676760970145 ) ) ;
#30400=CARTESIAN_POINT ( 'NONE',  ( -4.609996619675000851, 1516.769879638719885, 212.5810025483170023 ) ) ;
#30414=DIRECTION ( 'NONE',  ( 0.000000000000000000, -0.9996573249755569268, 0.02617694830788849791 ) ) ;
#30421=CARTESIAN_POINT ( 'NONE',  ( -7.335901033725000353, 1517.068717944079935, 205.0869373723870126 ) ) ;
#30451=CARTESIAN_POINT ( 'NONE',  ( 8.463861902778212709, 1511.395344347295122, 204.2992659969390559 ) ) ;
#30461=CARTESIAN_POINT ( 'NONE',  ( -13.19864381506500095, 1513.023086264660151, 192.2692346079670074 ) ) ;
#30465=CARTESIAN_POINT ( 'NONE',  ( 0.7396922377450010355, 1517.135701590510052, 201.7845486201169933 ) ) ;
#30477=CARTESIAN_POINT ( 'NONE',  ( -5.004442077193687943, 1516.690345683714668, 201.4087281776068039 ) ) ;
#30494=EDGE_LOOP ( 'NONE', ( #11595, #34019, #5860, #46911, #36950 ) ) ;
#30500=CARTESIAN_POINT ( 'NONE',  ( 3.455377977254999955, 1516.627618683580067, 216.0573038954169931 ) ) ;
#30507=CARTESIAN_POINT ( 'NONE',  ( 3.254401403604999743, 1516.919782530640077, 205.0791161293069820 ) ) ;
#30509=CARTESIAN_POINT ( 'NONE',  ( 0.007128837152181529378, 1517.006509894990131, 209.8686634857439799 ) ) ;
#30517=CARTESIAN_POINT ( 'NONE',  ( 5.513435558243076073, 1508.731359867040283, 216.5668839540665260 ) ) ;
#30523=CARTESIAN_POINT ( 'NONE',  ( -4.997573825325000385, 1516.742629295279812, 212.5803724681170195 ) ) ;
#30528=CARTESIAN_POINT ( 'NONE',  ( -7.715319381269040377, 1516.774419107829999, 209.6761046150799928 ) ) ;
#30529=CARTESIAN_POINT ( 'NONE',  ( -4.995623491025000362, 1516.636036526019780, 210.8344906863870278 ) ) ;
#30545=CIRCLE ( 'NONE', #71687, 1.000000000000057732 ) ;
#30546=CARTESIAN_POINT ( 'NONE',  ( -4.615644842514999624, 1517.009964551830080, 216.0692237534070159 ) ) ;
#30551=CARTESIAN_POINT ( 'NONE',  ( -0.7533001734329990429, 1516.714320817460020, 201.7957737879569891 ) ) ;
#30582=CARTESIAN_POINT ( 'NONE',  ( -14.72577118585429901, 1514.214451951579804, 224.1399941292770279 ) ) ;
#30585=CARTESIAN_POINT ( 'NONE',  ( -0.008139190548902429725, 1516.932212683830130, 201.4023955549550067 ) ) ;
#30591=CARTESIAN_POINT ( 'NONE',  ( 13.46561924343290073, 1512.674009804170055, 224.4294812528409864 ) ) ;
#30633=CARTESIAN_POINT ( 'NONE',  ( -6.933587693644999383, 1516.542957540330008, 210.8312046333570038 ) ) ;
#30634=VECTOR ( 'NONE', #59112, 1000.000000000000114 ) ;
#30636=CARTESIAN_POINT ( 'NONE',  ( 2.299014030735000436, 1516.811292230880099, 211.9858893885470081 ) ) ;
#30642=CARTESIAN_POINT ( 'NONE',  ( -1.128757599205000073, 1516.608208975040043, 201.4108789544669946 ) ) ;
#30657=CARTESIAN_POINT ( 'NONE',  ( -2.284053509485000077, 1516.854133554269993, 210.2586600040969813 ) ) ;
#30663=CARTESIAN_POINT ( 'NONE',  ( 7.735039549035001016, 1511.353635254350138, 205.6398665129370045 ) ) ;
#30664=CARTESIAN_POINT ( 'NONE',  ( -7.727327152855000492, 1517.232977404109988, 207.4118332116069894 ) ) ;
#30666=DIRECTION ( 'NONE',  ( -0.001614263105669359660, 0.06164622090537578980, 0.9980967576356069015 ) ) ;
#30679=CARTESIAN_POINT ( 'NONE',  ( -7.326795561505000443, 1516.760434454289907, 214.9020780475669881 ) ) ;
#30681=CARTESIAN_POINT ( 'NONE',  ( 7.709564572731689935, 1516.554653292440207, 207.5021949886239838 ) ) ;
#30683=CARTESIAN_POINT ( 'NONE',  ( -7.006565531035000127, 1516.551704408390151, 197.1655329708669910 ) ) ;
#30706=CARTESIAN_POINT ( 'NONE',  ( -5.551188712105000533, 1510.480349266450048, 201.5713426081769910 ) ) ;
#30748=CARTESIAN_POINT ( 'NONE',  ( -2.299668004004999933, 1516.965971551240045, 208.0037412025070012 ) ) ;
#30759=CARTESIAN_POINT ( 'NONE',  ( -15.24308032758169951, 1512.436270050390021, 222.2069269479069931 ) ) ;
#30783=CARTESIAN_POINT ( 'NONE',  ( -3.487584143074780041, 1508.551704408389924, 204.1347675025799902 ) ) ;
#30785=CARTESIAN_POINT ( 'NONE',  ( 1.121950743945000051, 1517.123342927159911, 204.1084165760470057 ) ) ;
#30807=ORIENTED_EDGE ( 'NONE', *, *, #108264, .F. ) ;
#30875=CARTESIAN_POINT ( 'NONE',  ( -4.726464430697979502, 1511.395334939705208, 200.6898615724287822 ) ) ;
#30881=CARTESIAN_POINT ( 'NONE',  ( -7.336844680545000053, 1517.106845464700200, 205.6683011064770312 ) ) ;
#30896=CARTESIAN_POINT ( 'NONE',  ( 1.717139084115000047, 1516.949031626070109, 210.2396860569670025 ) ) ;
#30911=ORIENTED_EDGE ( 'NONE', *, *, #72659, .F. ) ;
#30922=CARTESIAN_POINT ( 'NONE',  ( -3.780286426965000057, 1510.542924508009946, 201.5697040178069983 ) ) ;
#30928=CARTESIAN_POINT ( 'NONE',  ( 4.997718238375000510, 1516.693851263360102, 207.9888968556769839 ) ) ;
#30933=ORIENTED_EDGE ( 'NONE', *, *, #11208, .F. ) ;
#30941=CARTESIAN_POINT ( 'NONE',  ( -5.550449896747339018, 1510.476657126699820, 201.5714335428820050 ) ) ;
#30944=CARTESIAN_POINT ( 'NONE',  ( -6.023224945624109594, 1510.704533469413036, 201.6205954506678495 ) ) ;
#30949=CARTESIAN_POINT ( 'NONE',  ( -1.126138146715000010, 1517.208444099459939, 216.8485306577670144 ) ) ;
#30951=DIRECTION ( 'NONE',  ( -0.06162841671618448508, -0.9961946980917499861, -0.06162841671618445039 ) ) ;
#30953=CARTESIAN_POINT ( 'NONE',  ( 2.587404269808366575, 1516.541469363555507, 216.8310653096392571 ) ) ;
#30954=CARTESIAN_POINT ( 'NONE',  ( -7.323034312095000331, 1516.609912606490070, 212.5765947784269940 ) ) ;
#30971=CARTESIAN_POINT ( 'NONE',  ( 4.997573787194999895, 1516.742629295279812, 205.6633194342169872 ) ) ;
#30999=CARTESIAN_POINT ( 'NONE',  ( 7.932497417486165325, 1511.860489184832204, 205.9801110084320896 ) ) ;
#31006=CARTESIAN_POINT ( 'NONE',  ( -7.522201478567969168, 1510.631883387999551, 215.0340703743040081 ) ) ;
#31009=CARTESIAN_POINT ( 'NONE',  ( -12.38551416666500060, 1511.900571936589813, 193.4278863644669855 ) ) ;
#31013=CARTESIAN_POINT ( 'NONE',  ( 7.716252052974999387, 1516.810037859429940, 202.1795012402670011 ) ) ;
#31016=CARTESIAN_POINT ( 'NONE',  ( 16.00554743903499855, 1513.636261293280086, 194.3802644824669983 ) ) ;
#31043=EDGE_CURVE ( 'NONE', #2720, #63057, #92763, .T. ) ;
#31048=CARTESIAN_POINT ( 'NONE',  ( 2.873958851594999864, 1516.588006113850042, 216.0563744999969913 ) ) ;
#31057=CARTESIAN_POINT ( 'NONE',  ( 6.547556931335000385, 1516.633288330999903, 205.8595812817970057 ) ) ;
#31059=CARTESIAN_POINT ( 'NONE',  ( 1.133653140995000141, 1516.978425811520083, 209.8592968530090275 ) ) ;
#31062=FACE_OUTER_BOUND ( 'NONE', #50306, .T. ) ;
#31072=CARTESIAN_POINT ( 'NONE',  ( -5.773668852974999766, 1516.734985836460055, 213.1604834329569940 ) ) ;
#31077=CARTESIAN_POINT ( 'NONE',  ( -7.713124426543250145, 1516.690597168669910, 209.9915660461619780 ) ) ;
#31078=CARTESIAN_POINT ( 'NONE',  ( -2.282301616165000269, 1516.836638729160086, 210.8392784184970026 ) ) ;
#31093=CARTESIAN_POINT ( 'NONE',  ( -6.554151464375000735, 1516.906641539930206, 216.4536580562070185 ) ) ;
#31098=CARTESIAN_POINT ( 'NONE',  ( 6.941100277744999936, 1516.858069504249897, 202.1782432786469883 ) ) ;
#31099=CARTESIAN_POINT ( 'NONE',  ( -14.92003716616500064, 1512.136030808819896, 221.5058330632670049 ) ) ;
#31125=CARTESIAN_POINT ( 'NONE',  ( -13.82860589446197075, 1517.051704408389924, 226.2317424102079144 ) ) ;
#31126=FACE_OUTER_BOUND ( 'NONE', #87821, .T. ) ;
#31134=CARTESIAN_POINT ( 'NONE',  ( 13.83393986337329906, 1512.951873711600001, 224.4212087918060092 ) ) ;
#31161=ADVANCED_FACE ( 'NONE', ( #46280 ), #80407, .T. ) ;
#31173=CARTESIAN_POINT ( 'NONE',  ( -3.445407572115000150, 1516.764084769670262, 211.4198948937369948 ) ) ;
#31177=CARTESIAN_POINT ( 'NONE',  ( 0.7572979362240020995, 1516.829948096479939, 212.5714934102470011 ) ) ;
#31186=CARTESIAN_POINT ( 'NONE',  ( -0.01171164408179850049, 1516.939568781210028, 202.5649949355269825 ) ) ;
#31196=DIRECTION ( 'NONE',  ( -1.000000000000000000, 0.000000000000000000, 0.000000000000000000 ) ) ;
#31198=CARTESIAN_POINT ( 'NONE',  ( -11.95631299936500014, 1516.551704408390151, 216.1284114631369846 ) ) ;
#31204=CARTESIAN_POINT ( 'NONE',  ( 7.726684687535000151, 1517.208444099459939, 210.2479840788170122 ) ) ;
#31210=CARTESIAN_POINT ( 'NONE',  ( 4.610079833424999940, 1516.713079096360161, 207.9883289669969884 ) ) ;
#31218=DIRECTION ( 'NONE',  ( 0.02616798426500965835, -0.9993150019883683122, 0.02616798426500970692 ) ) ;
#31229=CARTESIAN_POINT ( 'NONE',  ( 4.617490466775000080, 1516.685667699390024, 216.4467608883869900 ) ) ;
#31231=CARTESIAN_POINT ( 'NONE',  ( 7.709251280239639570, 1516.542689134859984, 207.3693600638700048 ) ) ;
#31260=CARTESIAN_POINT ( 'NONE',  ( -5.121512578775000435, 1511.279956263560052, 201.1879310057669841 ) ) ;
#31286=ORIENTED_EDGE ( 'NONE', *, *, #61646, .F. ) ;
#31295=CARTESIAN_POINT ( 'NONE',  ( -8.454424074398959377, 1511.603884447429891, 214.9855816549980148 ) ) ;
#31300=CARTESIAN_POINT ( 'NONE',  ( -6.951517170504999399, 1517.194816588360027, 207.9969518818670053 ) ) ;
#31305=ORIENTED_EDGE ( 'NONE', *, *, #4667, .F. ) ;
#31323=ORIENTED_EDGE ( 'NONE', *, *, #19892, .F. ) ;
#31327=CARTESIAN_POINT ( 'NONE',  ( 3.910153960660829764, 1508.551704408439946, 204.2884083744090162 ) ) ;
#31334=CARTESIAN_POINT ( 'NONE',  ( -2.296124889065000119, 1516.677239312369920, 204.5136991508470032 ) ) ;
#31345=CARTESIAN_POINT ( 'NONE',  ( -13.96132456265650035, 1513.058738973280015, 193.8412935603610094 ) ) ;
#31357=CARTESIAN_POINT ( 'NONE',  ( -7.651189275224999697, 1514.325389163589989, 203.4154480846970046 ) ) ;
#31376=CARTESIAN_POINT ( 'NONE',  ( 11.12931921225938225, 1512.151624459632103, 224.9062103328911633 ) ) ;
#31427=CARTESIAN_POINT ( 'NONE',  ( -4.607530503061391336, 1511.399179795973851, 200.7291179019183005 ) ) ;
#31435=CARTESIAN_POINT ( 'NONE',  ( 6.935457925184999262, 1516.627618683580067, 205.6664679548470076 ) ) ;
#31440=ORIENTED_EDGE ( 'NONE', *, *, #55688, .T. ) ;
#31448=CARTESIAN_POINT ( 'NONE',  ( -4.610079871555000430, 1516.713079096360161, 210.2553629353369899 ) ) ;
#31474=CARTESIAN_POINT ( 'NONE',  ( -2.291676311554999845, 1516.534976163889951, 201.8006522243570089 ) ) ;
#31475=CARTESIAN_POINT ( 'NONE',  ( 6.938478784765000462, 1516.719999691880048, 208.3679751968140010 ) ) ;
#31485=LINE ( 'NONE', #99783, #40578 ) ;
#31488=CARTESIAN_POINT ( 'NONE',  ( -4.987078454525000204, 1509.051704408389924, 209.1727295022979831 ) ) ;
#31493=CARTESIAN_POINT ( 'NONE',  ( -5.004475612664999851, 1517.026025493960105, 216.8437538584669824 ) ) ;
#31499=CARTESIAN_POINT ( 'NONE',  ( 5.785582913545000316, 1516.981965530290154, 213.1542438721070027 ) ) ;
#31516=CARTESIAN_POINT ( 'NONE',  ( -2.879642191334999879, 1516.812046502680005, 205.6755161564470313 ) ) ;
#31531=EDGE_CURVE ( 'NONE', #39742, #106739, #109585, .T. ) ;
#31545=CARTESIAN_POINT ( 'NONE',  ( -4.277761497305760940, 1517.051704409989952, 216.4479871024050226 ) ) ;
#31548=CARTESIAN_POINT ( 'NONE',  ( 8.501597980927209974, 1511.397677006128788, 204.1858220046408974 ) ) ;
#31565=CARTESIAN_POINT ( 'NONE',  ( 6.940473334145000450, 1516.833525648419936, 202.5658237375970145 ) ) ;
#31568=CARTESIAN_POINT ( 'NONE',  ( 16.44381310503499805, 1512.620989416239809, 195.6052243943669851 ) ) ;
#31572=CARTESIAN_POINT ( 'NONE',  ( -17.14950101167192642, 1517.051704408390151, 195.3930630967549007 ) ) ;
#31580=CARTESIAN_POINT ( 'NONE',  ( -7.691516692145000000, 1512.326491219019999, 211.8199587616570057 ) ) ;
#31599=CARTESIAN_POINT ( 'NONE',  ( 6.942973629204999497, 1516.833844030519913, 216.4505221401170161 ) ) ;
#31607=CARTESIAN_POINT ( 'NONE',  ( -2.492443689034999910, 1516.793978928989873, 205.8699571027569846 ) ) ;
#31609=CARTESIAN_POINT ( 'NONE',  ( 6.556850996575000146, 1516.939568781210028, 209.1101343261499892 ) ) ;
#31613=CARTESIAN_POINT ( 'NONE',  ( 6.580362910585000336, 1511.382498894339733, 216.4385679756969978 ) ) ;
#31623=CARTESIAN_POINT ( 'NONE',  ( -1.121383629864999953, 1517.104192383289956, 213.7476359466970166 ) ) ;
#31627=CARTESIAN_POINT ( 'NONE',  ( -7.708942735038510463, 1516.530904812869949, 211.0733318003030092 ) ) ;
#31628=CARTESIAN_POINT ( 'NONE',  ( -1.701850495234999983, 1516.908147884120126, 210.2591426210370003 ) ) ;
#31638=VECTOR ( 'NONE', #39637, 1000.000000000000000 ) ;
#31643=CARTESIAN_POINT ( 'NONE',  ( 2.291676273424999799, 1516.534976163889951, 216.4430396779769978 ) ) ;
#31648=CARTESIAN_POINT ( 'NONE',  ( 3.452917022905000355, 1517.089216728169959, 202.1725802860869976 ) ) ;
#31682=ORIENTED_EDGE ( 'NONE', *, *, #86900, .T. ) ;
#31694=CARTESIAN_POINT ( 'NONE',  ( 15.20279577643499991, 1516.814170398969964, 225.0317485278669949 ) ) ;
#31724=CARTESIAN_POINT ( 'NONE',  ( -5.771149113014999443, 1516.616791731099966, 211.6102065995370083 ) ) ;
#31727=CARTESIAN_POINT ( 'NONE',  ( 1.714334247185000049, 1516.699825673279975, 213.1484604498870112 ) ) ;
#31736=CARTESIAN_POINT ( 'NONE',  ( 0.7391219670640019057, 1517.130100026000036, 202.1721425974470208 ) ) ;
#31752=CARTESIAN_POINT ( 'NONE',  ( -0.7351098092479989576, 1516.977504706749869, 211.6135016956469883 ) ) ;
#31757=CARTESIAN_POINT ( 'NONE',  ( 7.933914926335000395, 1511.279956263560052, 204.0003333914669952 ) ) ;
#31758=CARTESIAN_POINT ( 'NONE',  ( -7.338753868364999988, 1517.184383877180153, 206.8309596656170015 ) ) ;
#31778=CARTESIAN_POINT ( 'NONE',  ( 2.873958851594999864, 1516.588006113850042, 216.0563744999969913 ) ) ;
#31780=CARTESIAN_POINT ( 'NONE',  ( 7.715537193931590210, 1516.782738493960096, 208.5984514415330011 ) ) ;
#31812=CARTESIAN_POINT ( 'NONE',  ( -3.927225904784999777, 1511.005930286190051, 201.4860115694070259 ) ) ;
#31839=VERTEX_POINT ( 'NONE', #84517 ) ;
#31845=CARTESIAN_POINT ( 'NONE',  ( -17.05938549526129577, 1517.051704405600049, 195.1949804090679947 ) ) ;
#31848=CARTESIAN_POINT ( 'NONE',  ( -8.797412869267919433, 1511.644547967860035, 215.2508032624510008 ) ) ;
#31853=CARTESIAN_POINT ( 'NONE',  ( -5.781585816274999345, 1516.939646076049939, 209.1342929058909874 ) ) ;
#31854=VECTOR ( 'NONE', #104005, 1000.000000000000000 ) ;
#31880=CARTESIAN_POINT ( 'NONE',  ( 3.803002571174680213, 1508.880967335730247, 204.6292016602320132 ) ) ;
#31888=CARTESIAN_POINT ( 'NONE',  ( -4.487358483189090030, 1509.034524749680031, 205.3201112091969947 ) ) ;
#31890=CARTESIAN_POINT ( 'NONE',  ( 2.479246847704999812, 1516.983612918759945, 205.0778556245070092 ) ) ;
#31892=CARTESIAN_POINT ( 'NONE',  ( 3.034964868304999897, 1517.051704408389924, 200.9398869892670234 ) ) ;
#31894=CARTESIAN_POINT ( 'NONE',  ( 15.02944345243210122, 1512.205851781539877, 196.5435174618820042 ) ) ;
#31899=CARTESIAN_POINT ( 'NONE',  ( -12.62550847681250055, 1512.222316757829958, 194.0651229827790019 ) ) ;
#31910=CARTESIAN_POINT ( 'NONE',  ( -7.636446066375000008, 1514.050458741980037, 203.1354708283169828 ) ) ;
#31913=DIRECTION ( 'NONE',  ( 0.02616798426500960631, -0.9993150019883683122, -0.02616798426500955774 ) ) ;
#31983=CARTESIAN_POINT ( 'NONE',  ( -3.806637153123912043, 1511.520884442064244, 200.9879143131876162 ) ) ;
#31989=CARTESIAN_POINT ( 'NONE',  ( 6.547556931335000385, 1516.633288330999903, 205.8595812817970057 ) ) ;
#31990=CIRCLE ( 'NONE', #46338, 0.9999999999999685807 ) ;
#31999=ORIENTED_EDGE ( 'NONE', *, *, #50256, .F. ) ;
#32004=CARTESIAN_POINT ( 'NONE',  ( 5.789394662204999875, 1517.164987839469859, 210.8286437561770299 ) ) ;
#32032=CARTESIAN_POINT ( 'NONE',  ( 2.290256263724999908, 1517.170721208160103, 202.1706708033170230 ) ) ;
#32033=CARTESIAN_POINT ( 'NONE',  ( -6.952166420425000659, 1517.213554313520035, 207.4130983078469797 ) ) ;
#32051=CARTESIAN_POINT ( 'NONE',  ( -2.291514335905000088, 1517.194972660189933, 216.8481778957070105 ) ) ;
#32058=CARTESIAN_POINT ( 'NONE',  ( 1.714334247185000049, 1516.699825673279975, 213.1484604498870112 ) ) ;
#32077=CARTESIAN_POINT ( 'NONE',  ( 4.997250153905000047, 1516.727068157269969, 205.8570671527170077 ) ) ;
#32109=CARTESIAN_POINT ( 'NONE',  ( 7.894434426187861398, 1512.053483454368461, 206.1275301515672709 ) ) ;
#32125=CARTESIAN_POINT ( 'NONE',  ( -4.036748876935000396, 1516.667393516340098, 202.1854475764570225 ) ) ;
#32128=CARTESIAN_POINT ( 'NONE',  ( 15.40521415373500069, 1513.907445464720013, 194.0960529043670135 ) ) ;
#32134=ORIENTED_EDGE ( 'NONE', *, *, #77, .T. ) ;
#32158=CARTESIAN_POINT ( 'NONE',  ( -7.715625241105000143, 1516.786099423779888, 215.6766101314970001 ) ) ;
#32159=CARTESIAN_POINT ( 'NONE',  ( -8.353227804513524646, 1511.405761256387450, 213.6090188832756667 ) ) ;
#32166=CARTESIAN_POINT ( 'NONE',  ( 0.7355686427760019797, 1517.012231669750008, 205.8548062402470009 ) ) ;
#32168=CARTESIAN_POINT ( 'NONE',  ( -5.786847777804999815, 1517.104497701820037, 208.3841784293060186 ) ) ;
#32173=CARTESIAN_POINT ( 'NONE',  ( 6.610870897525000345, 1511.929989569699956, 216.5045975180869959 ) ) ;
#32182=CARTESIAN_POINT ( 'NONE',  ( -4.998515195425000002, 1516.787536375099990, 213.1617432482970003 ) ) ;
#32186=CARTESIAN_POINT ( 'NONE',  ( 7.508704985436030377, 1508.884117426709963, 214.6350462372689947 ) ) ;
#32187=CARTESIAN_POINT ( 'NONE',  ( 5.789394662204999875, 1517.164987839469859, 210.8286437561770299 ) ) ;
#32194=CIRCLE ( 'NONE', #73279, 1.000060826959960236 ) ;
#32205=CARTESIAN_POINT ( 'NONE',  ( 3.454119916704999849, 1516.594591938570147, 216.8324563732270178 ) ) ;
#32210=CARTESIAN_POINT ( 'NONE',  ( -0.7538707734179979081, 1516.719999691880048, 202.1833671473370089 ) ) ;
#32211=CARTESIAN_POINT ( 'NONE',  ( -16.85261136226499801, 1513.023086264660151, 222.3204897471670165 ) ) ;
#32239=PLANE ( 'NONE',  #100362 ) ;
#32248=ORIENTED_EDGE ( 'NONE', *, *, #11107, .T. ) ;
#32284=EDGE_LOOP ( 'NONE', ( #45211, #57939, #106109 ) ) ;
#32286=CARTESIAN_POINT ( 'NONE',  ( 0.7576635334400020350, 1516.855632454399938, 211.9899581013969794 ) ) ;
#32290=CARTESIAN_POINT ( 'NONE',  ( -3.253462098795000035, 1516.874084700499907, 212.5832060635069922 ) ) ;
#32297=ADVANCED_FACE ( 'NONE', ( #93328 ), #24458, .F. ) ;
#32298=CARTESIAN_POINT ( 'NONE',  ( -4.618749106614999711, 1516.729202374750002, 202.5720834851169911 ) ) ;
#32315=CARTESIAN_POINT ( 'NONE',  ( 2.299983577604999940, 1516.861367446839949, 211.4044688825970013 ) ) ;
#32322=CARTESIAN_POINT ( 'NONE',  ( -0.01265822594359850006, 1516.959716008189844, 207.4120794380770292 ) ) ;
#32324=FACE_OUTER_BOUND ( 'NONE', #73470, .T. ) ;
#32342=CARTESIAN_POINT ( 'NONE',  ( 7.718134629434999283, 1516.881930554049859, 216.4517759834270123 ) ) ;
#32371=CARTESIAN_POINT ( 'NONE',  ( -4.522891097415000061, 1511.193640125469983, 201.2736662571170143 ) ) ;
#32411=CARTESIAN_POINT ( 'NONE',  ( -8.290649527490709048, 1511.656200769810084, 215.0711531565719952 ) ) ;
#32418=CARTESIAN_POINT ( 'NONE',  ( -0.007128875282218469743, 1517.006509894990131, 208.3750284165899984 ) ) ;
#32426=CARTESIAN_POINT ( 'NONE',  ( -15.10840968467219980, 1512.260118274579781, 221.8456817057260082 ) ) ;
#32444=EDGE_CURVE ( 'NONE', #69935, #108962, #32582, .T. ) ;
#32455=CARTESIAN_POINT ( 'NONE',  ( 3.447264348965000558, 1516.858765657450249, 205.6607986404769974 ) ) ;
#32459=CARTESIAN_POINT ( 'NONE',  ( 14.94819994016220122, 1513.870294662249989, 194.3661611336529802 ) ) ;
#32464=CARTESIAN_POINT ( 'NONE',  ( -13.27508839399100005, 1512.548660307890032, 193.8371749040339864 ) ) ;
#32477=CARTESIAN_POINT ( 'NONE',  ( -8.126234285584999384, 1514.923664147150021, 202.9950997886369635 ) ) ;
#32486=VECTOR ( 'NONE', #67101, 1000.000000000000000 ) ;
#32495=CARTESIAN_POINT ( 'NONE',  ( -4.487249792034999629, 1509.038615934239942, 209.1218459511669892 ) ) ;
#32496=CARTESIAN_POINT ( 'NONE',  ( 2.234923043937409926, 1512.341036938790012, 216.7210731156089878 ) ) ;
#32500=B_SPLINE_CURVE_WITH_KNOTS ( 'NONE', 3,
 ( #27440, #70042, #6374, #33765, #61623, #40520, #57896, #95755 ),
 .UNSPECIFIED., .F., .F.,
 ( 4, 2, 2, 4 ),
 ( 0.000000000000000000, 0.2500000000000000000, 0.5000000000000000000, 1.000000000000000000 ),
 .UNSPECIFIED. ) ;
#32533=ORIENTED_EDGE ( 'NONE', *, *, #50627, .F. ) ;
#32543=CARTESIAN_POINT ( 'NONE',  ( -2.942030012410809636, 1512.314860016870171, 201.2300683927209946 ) ) ;
#32549=CARTESIAN_POINT ( 'NONE',  ( -3.267603553834999897, 1516.858171774179937, 205.8687047948669999 ) ) ;
#32552=CARTESIAN_POINT ( 'NONE',  ( -3.052975934615000053, 1516.551704408390151, 201.1191225673069880 ) ) ;
#32558=CARTESIAN_POINT ( 'NONE',  ( -16.78435733967954846, 1513.560745840784421, 222.3626190331726491 ) ) ;
#32562=CARTESIAN_POINT ( 'NONE',  ( -7.708770045145000083, 1516.524310051880093, 211.4128934593470035 ) ) ;
#32567=DIRECTION ( 'NONE',  ( -0.02616795315378250830, -0.9993150033772694174, -0.02616796233621986045 ) ) ;
#32582=CIRCLE ( 'NONE', #41536, 7.500000000000000000 ) ;
#32592=CARTESIAN_POINT ( 'NONE',  ( 3.453544825624999870, 1517.106845464700200, 201.7850012896870169 ) ) ;
#32593=CARTESIAN_POINT ( 'NONE',  ( -3.269025173884999802, 1517.026534522949987, 208.0024068424170025 ) ) ;
#32596=CARTESIAN_POINT ( 'NONE',  ( 4.613666293552466158, 1511.398924905619651, 217.5165917695272242 ) ) ;
#32604=CARTESIAN_POINT ( 'NONE',  ( 7.613968465965000654, 1512.903985260039917, 203.5071921160869977 ) ) ;
#32605=CARTESIAN_POINT ( 'NONE',  ( -17.05938549526129577, 1517.051704405600049, 195.1949804090679947 ) ) ;
#32611=CARTESIAN_POINT ( 'NONE',  ( -6.942354311545000378, 1516.905946377369901, 216.8406094761369900 ) ) ;
#32613=CARTESIAN_POINT ( 'NONE',  ( 7.734617087614999775, 1516.863303996349941, 201.3001138717470155 ) ) ;
#32614=PLANE ( 'NONE',  #60729 ) ;
#32616=CARTESIAN_POINT ( 'NONE',  ( -3.255967424474999650, 1516.989560013210166, 214.1335248082570217 ) ) ;
#32633=CARTESIAN_POINT ( 'NONE',  ( 6.546951682585000043, 1516.606339319019980, 206.2472570094369928 ) ) ;
#32652=CARTESIAN_POINT ( 'NONE',  ( -14.63125512773061665, 1514.438041836527418, 192.7641272998755824 ) ) ;
#32667=CARTESIAN_POINT ( 'NONE',  ( -7.535878286259929837, 1510.580107401401165, 214.9399003442833305 ) ) ;
#32670=CARTESIAN_POINT ( 'NONE',  ( -15.09659340796500082, 1514.030803186779849, 193.4062324905669925 ) ) ;
#32675=CARTESIAN_POINT ( 'NONE',  ( 2.483322453895000059, 1517.139039350860003, 202.5585910412470128 ) ) ;
#32678=CARTESIAN_POINT ( 'NONE',  ( 15.78855998223499846, 1512.525301340730039, 195.5242935507669984 ) ) ;
#32709=CARTESIAN_POINT ( 'NONE',  ( -1.124894088365000044, 1517.194816588360027, 216.0733631026070043 ) ) ;
#32710=CARTESIAN_POINT ( 'NONE',  ( -8.412838876992196901, 1511.396718925154573, 213.7904301685088342 ) ) ;
#32718=CARTESIAN_POINT ( 'NONE',  ( -5.786837717054999608, 1517.040132827679827, 205.8646253294070050 ) ) ;
#32720=CARTESIAN_POINT ( 'NONE',  ( -2.292217048824999992, 1516.941178807709775, 209.1350424789999920 ) ) ;
#32732=CARTESIAN_POINT ( 'NONE',  ( -4.999456428534999830, 1516.830644417779922, 213.7431138541670066 ) ) ;
#32736=CARTESIAN_POINT ( 'NONE',  ( 6.648352156676600622, 1508.610125823030103, 216.2179235647060125 ) ) ;
#32737=CARTESIAN_POINT ( 'NONE',  ( 1.137296650804999976, 1516.908147884120126, 210.8236964273370120 ) ) ;
#32749=CARTESIAN_POINT ( 'NONE',  ( 12.13495036573499952, 1511.961073825299991, 225.2306057305669924 ) ) ;
#32751=PLANE ( 'NONE',  #3069 ) ;
#32755=CARTESIAN_POINT ( 'NONE',  ( 6.552897366944999469, 1516.858146885269889, 202.5651945608169910 ) ) ;
#32765=CARTESIAN_POINT ( 'NONE',  ( -11.75704297446499957, 1511.932705841380084, 218.3428388715770154 ) ) ;
#32826=CARTESIAN_POINT ( 'NONE',  ( -5.772727946874999461, 1516.691414181030041, 212.5791125756269935 ) ) ;
#32831=CARTESIAN_POINT ( 'NONE',  ( 1.124289655455000148, 1517.184063036290127, 202.5579304082170040 ) ) ;
#32843=LINE ( 'NONE', #31198, #59248 ) ;
#32844=CARTESIAN_POINT ( 'NONE',  ( -10.96015512746500065, 1516.551704408390151, 193.2119433744669834 ) ) ;
#32846=CARTESIAN_POINT ( 'NONE',  ( 7.338753830235000386, 1517.184383877180153, 211.4127322367170052 ) ) ;
#32852=CARTESIAN_POINT ( 'NONE',  ( 1.117840086735000016, 1516.949031626070109, 207.4047068479870006 ) ) ;
#32868=ADVANCED_FACE ( 'NONE', ( #87443 ), #10405, .T. ) ;
#32869=CARTESIAN_POINT ( 'NONE',  ( -0.7369042090349989804, 1517.080322339569875, 214.1333973382469935 ) ) ;
#32872=CARTESIAN_POINT ( 'NONE',  ( 4.036119644515000715, 1516.647924054489977, 216.4458205765370167 ) ) ;
#32909=CARTESIAN_POINT ( 'NONE',  ( -1.906501312376459942E-08, 1515.051704408389924, 213.4516374609670208 ) ) ;
#32932=CARTESIAN_POINT ( 'NONE',  ( 5.563540928143850373, 1516.551188145990182, 199.3082484782189852 ) ) ;
#32933=ORIENTED_EDGE ( 'NONE', *, *, #46780, .F. ) ;
#32944=CARTESIAN_POINT ( 'NONE',  ( -7.899414352548780549, 1511.275771545139833, 214.6924451503199975 ) ) ;
#32950=CARTESIAN_POINT ( 'NONE',  ( -6.562094107424999656, 1517.122674412569950, 208.3832410274270046 ) ) ;
#32959=CARTESIAN_POINT ( 'NONE',  ( -14.72576942166499947, 1512.123542805230272, 221.3115653187670091 ) ) ;
#32983=CARTESIAN_POINT ( 'NONE',  ( -4.621897862544999569, 1516.858533673840157, 204.5099662467769974 ) ) ;
#32986=CARTESIAN_POINT ( 'NONE',  ( 15.30997864848029977, 1512.715996828740117, 195.5972901532690003 ) ) ;
#33006=VERTEX_POINT ( 'NONE', #63239 ) ;
#33031=CARTESIAN_POINT ( 'NONE',  ( -15.17646696946499851, 1515.958428328729951, 225.0580773729669772 ) ) ;
#33041=EDGE_LOOP ( 'NONE', ( #85676, #104262, #6381, #70617, #82865, #106385, #97446, #99295 ) ) ;
#33057=CARTESIAN_POINT ( 'NONE',  ( 17.15254153798874981, 1516.551704399887512, 196.9190519997810611 ) ) ;
#33083=CARTESIAN_POINT ( 'NONE',  ( -1.136004312195000088, 1516.815173273089840, 206.2562091229970065 ) ) ;
#33098=CARTESIAN_POINT ( 'NONE',  ( 1.136547584984999970, 1516.839862955080207, 211.5998212856970042 ) ) ;
#33120=CARTESIAN_POINT ( 'NONE',  ( 5.018135791179288319, 1516.818301249119031, 214.7147315454415946 ) ) ;
#33125=ORIENTED_EDGE ( 'NONE', *, *, #28818, .F. ) ;
#33126=CARTESIAN_POINT ( 'NONE',  ( -7.718134667564999774, 1516.881930554049859, 201.7919159189069944 ) ) ;
#33127=CARTESIAN_POINT ( 'NONE',  ( -6.562094107424999656, 1517.122674412569950, 208.3832410274270046 ) ) ;
#33130=CARTESIAN_POINT ( 'NONE',  ( 3.112680624948092500, 1511.889619707009842, 217.0463476667217151 ) ) ;
#33147=CARTESIAN_POINT ( 'NONE',  ( -4.034908597844999889, 1517.068717944079935, 216.4577469658269990 ) ) ;
#33150=CARTESIAN_POINT ( 'NONE',  ( 1.739050608666847131, 1516.540855186845874, 216.8310492268561802 ) ) ;
#33151=CARTESIAN_POINT ( 'NONE',  ( -4.611879723454999969, 1516.858533673840157, 213.7437437946470027 ) ) ;
#33169=CARTESIAN_POINT ( 'NONE',  ( -1.715361130375000043, 1516.743010792419909, 205.6766444437269854 ) ) ;
#33193=DIRECTION ( 'NONE',  ( 0.7044160264027579110, -0.08715574274767008689, -0.7044160264027579110 ) ) ;
#33199=CARTESIAN_POINT ( 'NONE',  ( -1.906499846882070084E-08, 1517.051704408389924, 209.1218459511669892 ) ) ;
#33218=CARTESIAN_POINT ( 'NONE',  ( -1.131796848745000084, 1516.659138130710289, 203.3488676535569937 ) ) ;
#33221=CARTESIAN_POINT ( 'NONE',  ( 15.10381381093499975, 1513.853571676670072, 194.2467028014669950 ) ) ;
#33238=CARTESIAN_POINT ( 'NONE',  ( 13.07344732962040013, 1516.551188146170034, 192.4513774157680075 ) ) ;
#33241=FACE_OUTER_BOUND ( 'NONE', #90026, .T. ) ;
#33245=CARTESIAN_POINT ( 'NONE',  ( 6.126746143464999683, 1514.923664147150021, 200.9956116846470309 ) ) ;
#33253=CARTESIAN_POINT ( 'NONE',  ( -3.454172653555000139, 1517.122088787240045, 216.8462693643270143 ) ) ;
#33254=CARTESIAN_POINT ( 'NONE',  ( -8.143463389314709033, 1511.512554418091668, 212.9586518629134275 ) ) ;
#33260=ORIENTED_EDGE ( 'NONE', *, *, #110424, .F. ) ;
#33261=CARTESIAN_POINT ( 'NONE',  ( -4.042729840925000317, 1516.919782530640077, 205.8674445284970034 ) ) ;
#33262=ORIENTED_EDGE ( 'NONE', *, *, #76944, .F. ) ;
#33266=CARTESIAN_POINT ( 'NONE',  ( 7.668984210275000102, 1514.216129015430170, 215.2460172970970120 ) ) ;
#33273=CARTESIAN_POINT ( 'NONE',  ( 0.01306000193830150063, 1516.939762005280045, 213.7404293621069939 ) ) ;
#33278=CARTESIAN_POINT ( 'NONE',  ( 6.563254890855000134, 1517.139039350860003, 211.6051684241269868 ) ) ;
#33291=LINE ( 'NONE', #33848, #35753 ) ;
#33296=CARTESIAN_POINT ( 'NONE',  ( -2.874588960795000148, 1516.606339319019980, 202.5748942495170013 ) ) ;
#33320=PRODUCT_DEFINITION_FORMATION_WITH_SPECIFIED_SOURCE ( 'ANY', '', #48283, .NOT_KNOWN. ) ;
#33326=CARTESIAN_POINT ( 'NONE',  ( 5.551188674472009588, 1510.480349264700180, 216.6723492941099778 ) ) ;
#33352=CARTESIAN_POINT ( 'NONE',  ( 7.540791903005830576, 1510.557600718605045, 203.3531818223969765 ) ) ;
#33357=EDGE_CURVE ( 'NONE', #44161, #17382, #88275, .T. ) ;
#33360=FACE_BOUND ( 'NONE', #45368, .T. ) ;
#33366=ORIENTED_EDGE ( 'NONE', *, *, #84206, .T. ) ;
#33372=CARTESIAN_POINT ( 'NONE',  ( -6.935457963315000640, 1516.627618683580067, 212.5772239474869991 ) ) ;
#33377=CARTESIAN_POINT ( 'NONE',  ( -2.486474780875000512, 1516.560253536979872, 202.1879665292270261 ) ) ;
#33389=CARTESIAN_POINT ( 'NONE',  ( -3.487592467065220081, 1508.551704408389924, 204.1347675093749956 ) ) ;
#33391=CARTESIAN_POINT ( 'NONE',  ( 2.881548424445000034, 1516.909589401870107, 211.4054166033970148 ) ) ;
#33394=VECTOR ( 'NONE', #39950, 1000.000000000000000 ) ;
#33397=CARTESIAN_POINT ( 'NONE',  ( -3.462835665494999660, 1517.038650117239968, 208.0021282158369900 ) ) ;
#33399=DIRECTION ( 'NONE',  ( -1.000000000000000000, 0.000000000000000000, 0.000000000000000000 ) ) ;
#33411=CARTESIAN_POINT ( 'NONE',  ( -5.775236830874999505, 1516.804776704140068, 214.1294346171470124 ) ) ;
#33414=CARTESIAN_POINT ( 'NONE',  ( -5.002593397454999646, 1516.960844870249957, 215.6810146069769871 ) ) ;
#33459=CARTESIAN_POINT ( 'NONE',  ( -7.649034438594999763, 1514.243099272629934, 203.4721261815869866 ) ) ;
#33477=CARTESIAN_POINT ( 'NONE',  ( 7.722580339391510229, 1517.051704402239920, 213.7119063846940037 ) ) ;
#33485=CARTESIAN_POINT ( 'NONE',  ( -7.551708712715099026, 1510.523965798400013, 214.8518856309849809 ) ) ;
#33490=CARTESIAN_POINT ( 'NONE',  ( -6.949703372784999722, 1517.130100026000036, 208.3827239650380250 ) ) ;
#33499=CARTESIAN_POINT ( 'NONE',  ( -15.28055240982140006, 1513.058738973559912, 223.0831704950950041 ) ) ;
#33508=CARTESIAN_POINT ( 'NONE',  ( -5.513435596820279727, 1509.038615934079871, 216.6345961782780023 ) ) ;
#33523=CARTESIAN_POINT ( 'NONE',  ( -6.948321743994999800, 1517.049325831759916, 205.0875650164470017 ) ) ;
#33526=CARTESIAN_POINT ( 'NONE',  ( 15.31239853924400052, 1512.759354980439866, 195.5364289879649959 ) ) ;
#33569=CARTESIAN_POINT ( 'NONE',  ( 6.252266454184999489, 1511.741868877540128, 217.9101624594169948 ) ) ;
#33578=CARTESIAN_POINT ( 'NONE',  ( -2.478306858074999841, 1516.938330505699923, 212.5844667883370107 ) ) ;
#33612=CARTESIAN_POINT ( 'NONE',  ( 2.182463076968403026, 1517.051704408389924, 201.3992656178301104 ) ) ;
#33621=CARTESIAN_POINT ( 'NONE',  ( 4.996642160164999957, 1516.697242742309982, 206.2447328616370044 ) ) ;
#33633=CARTESIAN_POINT ( 'NONE',  ( -16.51878316591069051, 1514.214507862061282, 223.4467145224746503 ) ) ;
#33637=CARTESIAN_POINT ( 'NONE',  ( 6.951175128784999657, 1517.170721208160103, 211.4121022339570004 ) ) ;
#33663=CARTESIAN_POINT ( 'NONE',  ( 7.709487153813650018, 1516.551696783219995, 206.3620776923469862 ) ) ;
#33666=( BOUNDED_CURVE ( )  B_SPLINE_CURVE ( 3, ( #83790, #102238, #16010, #7627 ),
 .UNSPECIFIED., .F., .F. ) 
 B_SPLINE_CURVE_WITH_KNOTS ( ( 4, 4 ),
 ( 5.113530135711883418, 5.899158457943692646 ),
 .UNSPECIFIED. ) 
 CURVE ( )  GEOMETRIC_REPRESENTATION_ITEM ( )  RATIONAL_B_SPLINE_CURVE ( ( 1.000000000000000000, 0.9492236582716190307, 0.9492236582716190307, 1.000000000000000000 ) ) 
 REPRESENTATION_ITEM ( '' )  );
#33670=CARTESIAN_POINT ( 'NONE',  ( -4.616861546545000472, 1516.666407245520077, 201.4093549791169835 ) ) ;
#33671=CARTESIAN_POINT ( 'NONE',  ( -2.292217048824999992, 1516.941178807709775, 209.1350424789999920 ) ) ;
#33675=CARTESIAN_POINT ( 'NONE',  ( 3.747594548549652682, 1511.538158271216844, 217.2371947740062978 ) ) ;
#33692=VERTEX_POINT ( 'NONE', #29329 ) ;
#33693=EDGE_CURVE ( 'NONE', #42748, #100324, #59301, .T. ) ;
#33695=CARTESIAN_POINT ( 'NONE',  ( 2.086567662868722639, 1516.527846576654156, 216.8307085844099902 ) ) ;
#33696=CARTESIAN_POINT ( 'NONE',  ( 2.877744946244999991, 1516.723920667490120, 213.7309102736070088 ) ) ;
#33707=CARTESIAN_POINT ( 'NONE',  ( -9.500116237244998985, 1517.051704408389924, 222.5297078019669925 ) ) ;
#33715=CARTESIAN_POINT ( 'NONE',  ( -2.879956963085000154, 1516.827328999679821, 205.8693153165069702 ) ) ;
#33718=CARTESIAN_POINT ( 'NONE',  ( 7.454017752073605507, 1508.783371651613606, 214.6352815282469919 ) ) ;
#33732=CARTESIAN_POINT ( 'NONE',  ( 7.649034400464999273, 1514.243099272629934, 214.7715657207469917 ) ) ;
#33760=CARTESIAN_POINT ( 'NONE',  ( -7.722580350941189664, 1517.051704403100075, 204.5317855550379988 ) ) ;
#33764=CARTESIAN_POINT ( 'NONE',  ( 2.869693458934999608, 1517.070197312179971, 203.3343689375869872 ) ) ;
#33765=CARTESIAN_POINT ( 'NONE',  ( -8.742206007015797198, 1511.494976269418885, 214.8332494757211464 ) ) ;
#33768=CARTESIAN_POINT ( 'NONE',  ( 15.90990501073499885, 1514.921193539169963, 193.9190473980669935 ) ) ;
#33789=CARTESIAN_POINT ( 'NONE',  ( 5.371346801045000063, 1516.551704408390151, 199.4837300725270097 ) ) ;
#33794=CARTESIAN_POINT ( 'NONE',  ( 7.179127081225000317, 1513.978875661340226, 201.3127820188869919 ) ) ;
#33803=CARTESIAN_POINT ( 'NONE',  ( -2.872208748294999836, 1517.145312756229941, 216.4596396827270155 ) ) ;
#33804=CARTESIAN_POINT ( 'NONE',  ( -8.280691316095005305, 1511.427926070383592, 213.3861107695062458 ) ) ;
#33811=CARTESIAN_POINT ( 'NONE',  ( 2.476733476015000157, 1516.858326417339867, 206.6281461634669938 ) ) ;
#33818=CARTESIAN_POINT ( 'NONE',  ( 7.266995407845000088, 1512.686126173240154, 215.9029788489869759 ) ) ;
#33830=CARTESIAN_POINT ( 'NONE',  ( -7.325541825264999751, 1516.710692850270107, 214.1269169785269924 ) ) ;
#33835=CARTESIAN_POINT ( 'NONE',  ( 5.788097227154999302, 1517.099836525840146, 211.6039138304569747 ) ) ;
#33845=ADVANCED_FACE ( 'NONE', ( #73714 ), #107838, .F. ) ;
#33848=CARTESIAN_POINT ( 'NONE',  ( -1.906499580428539872E-08, 1509.038615934239942, 216.6345961781970288 ) ) ;
#33853=CARTESIAN_POINT ( 'NONE',  ( -3.456007423304999993, 1516.647534046129977, 202.5739645571870255 ) ) ;
#33873=CARTESIAN_POINT ( 'NONE',  ( -4.554954843304989787, 1508.731366866819826, 212.6094325583730154 ) ) ;
#33889=VERTEX_POINT ( 'NONE', #30582 ) ;
#33931=CARTESIAN_POINT ( 'NONE',  ( -7.323974644434999348, 1516.647924054489977, 213.1579656147470132 ) ) ;
#33937=CARTESIAN_POINT ( 'NONE',  ( 2.482067860225000366, 1517.099836525840146, 203.3337487049469985 ) ) ;
#33939=AXIS2_PLACEMENT_3D ( 'NONE', #33789, #57919, #42208 ) ;
#33942=ADVANCED_FACE ( 'NONE', ( #58006 ), #32239, .F. ) ;
#33947=CARTESIAN_POINT ( 'NONE',  ( -7.098163004017622235, 1512.239113741280107, 216.2722064511740996 ) ) ;
#33949=CARTESIAN_POINT ( 'NONE',  ( -11.02428140918887145, 1512.359593911811089, 193.2458125109432672 ) ) ;
#33957=CARTESIAN_POINT ( 'NONE',  ( 3.269184908365000197, 1516.940296199220029, 211.4060453336370244 ) ) ;
#33962=CARTESIAN_POINT ( 'NONE',  ( 7.719640903004999721, 1516.939452820819952, 209.1117431028050078 ) ) ;
#33978=CARTESIAN_POINT ( 'NONE',  ( 1.133516965105000107, 1516.713079096360161, 213.7319258036569920 ) ) ;
#33981=CARTESIAN_POINT ( 'NONE',  ( 4.035490712554999249, 1516.630499592039996, 216.8333966482170183 ) ) ;
#33983=ORIENTED_EDGE ( 'NONE', *, *, #102639, .T. ) ;
#34019=ORIENTED_EDGE ( 'NONE', *, *, #14901, .F. ) ;
#34045=ORIENTED_EDGE ( 'NONE', *, *, #66692, .T. ) ;
#34063=CARTESIAN_POINT ( 'NONE',  ( 2.873919002525000099, 1516.940252185109784, 209.1085733957019954 ) ) ;
#34073=CARTESIAN_POINT ( 'NONE',  ( -15.30763532073890154, 1512.674009804170055, 222.5874652136580210 ) ) ;
#34083=CARTESIAN_POINT ( 'NONE',  ( -7.112123039035762595, 1509.032357807246171, 215.8638904077538996 ) ) ;
#34094=CARTESIAN_POINT ( 'NONE',  ( -4.429741958790829770, 1508.551704408389924, 204.3196020111140001 ) ) ;
#34096=CARTESIAN_POINT ( 'NONE',  ( 2.284199363404999961, 1516.940296199220029, 205.8526610237369994 ) ) ;
#34150=CARTESIAN_POINT ( 'NONE',  ( -0.7356989727169980231, 1517.020847257979995, 212.5827121409169820 ) ) ;
#34183=CARTESIAN_POINT ( 'NONE',  ( -7.947250565765000552, 1514.433282224309778, 212.1193490295570143 ) ) ;
#34192=CARTESIAN_POINT ( 'NONE',  ( 2.283570633165000086, 1516.909589401870107, 206.2402975076569760 ) ) ;
#34200=ORIENTED_EDGE ( 'NONE', *, *, #89043, .F. ) ;
#34201=CARTESIAN_POINT ( 'NONE',  ( -16.55311987254050976, 1514.160701262670727, 223.3688575977173514 ) ) ;
#34205=CARTESIAN_POINT ( 'NONE',  ( 0.7579843820170020230, 1516.883361325900069, 211.4083188566570186 ) ) ;
#34211=CARTESIAN_POINT ( 'NONE',  ( 2.344512076345889984, 1516.526058371499857, 216.8306617650070223 ) ) ;
#34222=VECTOR ( 'NONE', #92958, 1000.000000000000114 ) ;
#34225=CARTESIAN_POINT ( 'NONE',  ( -6.541070373676360461, 1517.051704644259871, 205.4524592699869743 ) ) ;
#34228=CARTESIAN_POINT ( 'NONE',  ( 0.9370951295164038353, 1516.671995221453471, 216.5711338223802045 ) ) ;
#34233=CARTESIAN_POINT ( 'NONE',  ( 5.776491095245000373, 1516.858301627840092, 203.3390965304970166 ) ) ;
#34234=CARTESIAN_POINT ( 'NONE',  ( -0.7402208985179988820, 1516.992029636990083, 209.8751463226419958 ) ) ;
#34259=CARTESIAN_POINT ( 'NONE',  ( 0.8535652294838238507, 1516.694903845322870, 216.8350831329449306 ) ) ;
#34271=CARTESIAN_POINT ( 'NONE',  ( -16.53923917176500069, 1512.406775501100128, 221.4068228132670129 ) ) ;
#34278=CARTESIAN_POINT ( 'NONE',  ( 3.252530615595000452, 1516.827328999679821, 206.2418890071470230 ) ) ;
#34297=VECTOR ( 'NONE', #87633, 1000.000000000000000 ) ;
#34311=ADVANCED_FACE ( 'NONE', ( #104626 ), #26249, .F. ) ;
#34313=VECTOR ( 'NONE', #16215, 1000.000000000000114 ) ;
#34331=CARTESIAN_POINT ( 'NONE',  ( 5.776491095245000373, 1516.858301627840092, 203.3390965304970166 ) ) ;
#34336=CARTESIAN_POINT ( 'NONE',  ( -1.906499846882070084E-08, 1508.551704408389924, 216.6218459511670176 ) ) ;
#34355=CARTESIAN_POINT ( 'NONE',  ( 7.337793712495000342, 1517.145312756229941, 211.9940546803969994 ) ) ;
#34360=CARTESIAN_POINT ( 'NONE',  ( 6.648850764465000118, 1513.600111798339867, 201.6549557653970055 ) ) ;
#34361=ORIENTED_EDGE ( 'NONE', *, *, #6913, .F. ) ;
#34363=B_SPLINE_CURVE_WITH_KNOTS ( 'NONE', 3,
 ( #36573, #86971, #26504, #52295, #25941, #60700, #94823, #87543, #86420, #9710, #52845, #1327, #10831, #45003, #104883, #28173, #62360, #106531, #12471, #55051, #47185, #81864, #107630, #97045, #39323, #46654, #82435, #90820, #48292, #37676, #63465, #38763, #105997, #71325, #21392, #64006, #72400, #5165, #99205, #54511, #80786, #13546, #105439, #73494, #21935, #97584, #4093, #80234, #89179, #29273 ),
 .UNSPECIFIED., .F., .F.,
 ( 4, 2, 2, 1, 1, 2, 2, 2, 2, 1, 1, 1, 2, 2, 2, 2, 1, 1, 1, 2, 2, 2, 2, 1, 1, 1, 1, 2, 2, 2, 4 ),
 ( 0.000000000000000000, 0.1249999999980263010, 0.1874999999970458908, 0.2187499999965475395, 0.2343749999963077590, 0.2421874999962046471, 0.2499999999961015629, 0.3749999999939591100, 0.4374999999929196082, 0.4687499999924066851, 0.4843749999921764249, 0.4921874999920613503, 0.4960937499919773064, 0.4999999999918932625, 0.6249999999912395632, 0.6874999999909128245, 0.7187499999907493997, 0.7343749999906674653, 0.7421874999906323822, 0.7460937499905788695, 0.7499999999905252457, 0.8124999999901119097, 0.8437499999898635528, 0.8593749999897393188, 0.8671874999896397318, 0.8710937499896164171, 0.8730468749896052039, 0.8740234374895728964, 0.8749999999895405889, 0.9374999999947704055, 1.000000000000000000 ),
 .UNSPECIFIED. ) ;
#34365=EDGE_CURVE ( 'NONE', #12028, #72956, #75038, .T. ) ;
#34370=CARTESIAN_POINT ( 'NONE',  ( -3.260357166894999992, 1517.133889586189980, 216.8465783791270098 ) ) ;
#34371=CARTESIAN_POINT ( 'NONE',  ( -7.892149748326827030, 1512.076650117315467, 212.1052314332001743 ) ) ;
#34377=CARTESIAN_POINT ( 'NONE',  ( -4.625359562974999506, 1517.025470194390209, 206.6416589153869836 ) ) ;
#34383=CARTESIAN_POINT ( 'NONE',  ( 8.038901785834998037, 1514.330398624150121, 216.0318990019970045 ) ) ;
#34391=CARTESIAN_POINT ( 'NONE',  ( -3.449777353855000062, 1516.974592746400049, 214.1332139170270068 ) ) ;
#34396=CARTESIAN_POINT ( 'NONE',  ( 7.338753830235000386, 1517.184383877180153, 211.4127322367170052 ) ) ;
#34405=CARTESIAN_POINT ( 'NONE',  ( -7.583791944165000132, 1511.751588929339960, 211.4475770739170173 ) ) ;
#34409=CARTESIAN_POINT ( 'NONE',  ( 1.708092266164999984, 1516.523379810429788, 216.8305916180169959 ) ) ;
#34414=CARTESIAN_POINT ( 'NONE',  ( 2.288357407604999949, 1517.116049120239950, 203.3334095979369920 ) ) ;
#34431=ORIENTED_EDGE ( 'NONE', *, *, #20758, .T. ) ;
#34442=CARTESIAN_POINT ( 'NONE',  ( -7.330468918998392702, 1514.095142040229348, 217.2263680036883784 ) ) ;
#34456=CARTESIAN_POINT ( 'NONE',  ( 7.152679178757631817, 1516.546162712742898, 206.8624663984998904 ) ) ;
#34462=CARTESIAN_POINT ( 'NONE',  ( 5.614206143365000123, 1512.939243228069927, 214.7360521135969975 ) ) ;
#34468=EDGE_CURVE ( 'NONE', #19916, #36663, #22241, .T. ) ;
#34472=ORIENTED_EDGE ( 'NONE', *, *, #97405, .T. ) ;
#34495=CARTESIAN_POINT ( 'NONE',  ( -6.937338783705000012, 1516.706638732659940, 213.7399656364970042 ) ) ;
#34500=CARTESIAN_POINT ( 'NONE',  ( 2.869693458934999608, 1517.070197312179971, 203.3343689375869872 ) ) ;
#34512=CARTESIAN_POINT ( 'NONE',  ( 2.299014030735000436, 1516.811292230880099, 211.9858893885470081 ) ) ;
#34517=CARTESIAN_POINT ( 'NONE',  ( -6.563915562015000482, 1517.184063036290127, 207.9975562766469750 ) ) ;
#34531=B_SPLINE_CURVE_WITH_KNOTS ( 'NONE', 3,
 ( #9454, #60430, #43620, #1628, #35205, #69948, #69392, #103503, #26805, #95669, #27355, #55895, #98416, #106811, #71621, #47482, #55340, #56433, #21688, #91122, #46946, #97858 ),
 .UNSPECIFIED., .F., .F.,
 ( 4, 2, 2, 2, 2, 2, 2, 2, 2, 2, 4 ),
 ( 0.000000000000000000, 0.2500000000000149325, 0.3750000000000188183, 0.4375000000000142109, 0.4687500000000092704, 0.5000000000000043299, 0.6250000000000006661, 0.6875000000000005551, 0.7500000000000003331, 0.8750000000000002220, 1.000000000000000000 ),
 .UNSPECIFIED. ) ;
#34532=CARTESIAN_POINT ( 'NONE',  ( 7.333070134885000257, 1516.955859323880077, 214.9008457440070003 ) ) ;
#34535=CARTESIAN_POINT ( 'NONE',  ( -1.710012758625000018, 1517.232977404109988, 216.8491730849570160 ) ) ;
#34543=UNCERTAINTY_MEASURE_WITH_UNIT (LENGTH_MEASURE( 1.000000000000000082E-05 ), #96849, 'distance_accuracy_value', 'NONE');
#34555=CARTESIAN_POINT ( 'NONE',  ( 7.512750207965000371, 1509.038615934239942, 203.6084103740869864 ) ) ;
#34570=CARTESIAN_POINT ( 'NONE',  ( -2.656885837651520088, 1516.545501335879862, 201.4125211066549923 ) ) ;
#34575=EDGE_CURVE ( 'NONE', #76843, #63015, #57554, .T. ) ;
#34617=CARTESIAN_POINT ( 'NONE',  ( -6.556851034704999748, 1516.939568781210028, 209.1335575761840175 ) ) ;
#34619=EDGE_CURVE ( 'NONE', #598, #53542, #107634, .T. ) ;
#34628=CARTESIAN_POINT ( 'NONE',  ( -15.20279581456499862, 1514.921193718960012, 223.6175349654670299 ) ) ;
#34635=CARTESIAN_POINT ( 'NONE',  ( -1.133653179125000188, 1516.978425811520083, 208.3843950493249793 ) ) ;
#34637=CARTESIAN_POINT ( 'NONE',  ( -7.512705432632942326, 1509.036904577181758, 214.8970115796141158 ) ) ;
#34650=CARTESIAN_POINT ( 'NONE',  ( 4.027697225915000345, 1516.766397346390022, 206.2431526829570032 ) ) ;
#34660=CARTESIAN_POINT ( 'NONE',  ( 6.701092419766749408, 1517.051709179849922, 212.9150655973879793 ) ) ;
#34678=DIRECTION ( 'NONE',  ( -0.7071067811865475727, 1.631342908290929020E-16, -0.7071067811865475727 ) ) ;
#34697=CARTESIAN_POINT ( 'NONE',  ( -6.548821979184999975, 1516.688761843659904, 213.1592242262869945 ) ) ;
#34710=LINE ( 'NONE', #8394, #34222 ) ;
#34735=DIRECTION ( 'NONE',  ( 6.997424531968003289E-18, -1.000000000000000000, 0.000000000000000000 ) ) ;
#34738=CARTESIAN_POINT ( 'NONE',  ( -6.807912280453931153, 1516.613882035576353, 212.2734087009808945 ) ) ;
#34742=CARTESIAN_POINT ( 'NONE',  ( -2.299014068865000038, 1516.811292230880099, 206.2578025137869986 ) ) ;
#34743=B_SPLINE_CURVE_WITH_KNOTS ( 'NONE', 3,
 ( #7593, #75907, #82093, #39552, #110059, #98893, #23282, #66431, #100547, #73726, #22711, #56909, #52929, #61349, #16515, #26027, #77571, #69746, #93249, #93781, #34456, #52387, #87062, #60223, #18191, #94341, #17619, #17058, #50705, #84836, #103865, #60791 ),
 .UNSPECIFIED., .F., .F.,
 ( 4, 2, 1, 2, 2, 1, 1, 2, 2, 2, 2, 2, 2, 1, 2, 2, 2, 4 ),
 ( 0.000000000000000000, 0.2303738508824927089, 0.2447722165626507185, 0.2483718079826913450, 0.2501716036927140729, 0.2519713994027368287, 0.2591705822428356787, 0.2879673136032326330, 0.3455607763240182706, 0.4607477017655827178, 0.4895444331259781734, 0.4967436159660749140, 0.5003432073861219243, 0.5039427988061689900, 0.5183411644863570311, 0.5759346272071285133, 0.6911215526486663707, 0.9214954035317776126 ),
 .UNSPECIFIED. ) ;
#34752=CARTESIAN_POINT ( 'NONE',  ( -16.77415066853143344, 1513.652806713756945, 222.5401386658989225 ) ) ;
#34756=CARTESIAN_POINT ( 'NONE',  ( 2.493699768634999536, 1516.858326417339867, 211.5985794462469869 ) ) ;
#34781=CARTESIAN_POINT ( 'NONE',  ( 7.507423019669499986, 1508.880864719049896, 202.9817166117040017 ) ) ;
#34786=CARTESIAN_POINT ( 'NONE',  ( -5.781490582474999584, 1516.807958722750072, 202.5702025453269925 ) ) ;
#34787=CARTESIAN_POINT ( 'NONE',  ( 3.267039691854999983, 1517.012231669750008, 209.8574146130079896 ) ) ;
#34790=CARTESIAN_POINT ( 'NONE',  ( 3.141734923518147760, 1511.860489184966582, 217.0543433876719916 ) ) ;
#34822=CARTESIAN_POINT ( 'NONE',  ( -14.83698687666500149, 1514.217947259989842, 224.2462661523670135 ) ) ;
#34827=CARTESIAN_POINT ( 'NONE',  ( 1.118903270415000151, 1517.003078582959688, 206.2405205581369785 ) ) ;
#34843=CARTESIAN_POINT ( 'NONE',  ( 5.593955189962967367, 1510.491946825949526, 216.6725509186245802 ) ) ;
#34878=CARTESIAN_POINT ( 'NONE',  ( 1.708102589285000139, 1517.199196846569976, 202.5572672468869939 ) ) ;
#34901=CARTESIAN_POINT ( 'NONE',  ( 4.043990307595000111, 1516.983612918759945, 211.6010928179370012 ) ) ;
#34905=CARTESIAN_POINT ( 'NONE',  ( 6.834484283424999695, 1513.760531203560049, 201.6007729010970024 ) ) ;
#34912=CARTESIAN_POINT ( 'NONE',  ( -7.645353532535000163, 1513.311928781879942, 216.5003517853270125 ) ) ;
#34915=CARTESIAN_POINT ( 'NONE',  ( 7.329925222404999552, 1516.833976295079992, 216.8387248732070134 ) ) ;
#34921=CARTESIAN_POINT ( 'NONE',  ( -6.562635860634999929, 1517.111322026010157, 206.2508942643169974 ) ) ;
#34927=CARTESIAN_POINT ( 'NONE',  ( 7.585800431785000519, 1513.656171171930055, 215.2887577227170084 ) ) ;
#34935=CARTESIAN_POINT ( 'NONE',  ( -1.705466448594999962, 1517.120861839400050, 214.1360410720469929 ) ) ;
#34940=CARTESIAN_POINT ( 'NONE',  ( 1.717084711415000076, 1516.819260244609950, 211.5980165671369946 ) ) ;
#34951=EDGE_CURVE ( 'NONE', #20905, #36027, #88801, .T. ) ;
#34959=CARTESIAN_POINT ( 'NONE',  ( -2.295485539174999978, 1516.651306816259876, 204.1261199623870368 ) ) ;
#35018=CARTESIAN_POINT ( 'NONE',  ( 7.550503318189189628, 1510.480349263560129, 203.5706572562480119 ) ) ;
#35040=CARTESIAN_POINT ( 'NONE',  ( -0.7360974767499980365, 1517.045004075700035, 213.1642344714070134 ) ) ;
#35046=CARTESIAN_POINT ( 'NONE',  ( 5.001338628314999646, 1516.911981270829983, 203.3378372969070256 ) ) ;
#35049=CARTESIAN_POINT ( 'NONE',  ( -7.722579826676089887, 1517.051704428850144, 208.6871515679729896 ) ) ;
#35061=CARTESIAN_POINT ( 'NONE',  ( 3.461360093275000160, 1516.874084700499907, 212.3753080308970311 ) ) ;
#35068=CARTESIAN_POINT ( 'NONE',  ( 7.332063939445000678, 1516.939491476980038, 209.1111146381379911 ) ) ;
#35081=CARTESIAN_POINT ( 'NONE',  ( 0.4392564578464259739, 1517.051704408389924, 201.5953311768700189 ) ) ;
#35084=CARTESIAN_POINT ( 'NONE',  ( -1.705466448594999962, 1517.120861839400050, 214.1360410720469929 ) ) ;
#35087=CARTESIAN_POINT ( 'NONE',  ( 7.329925222404999552, 1516.833976295079992, 216.8387248732070134 ) ) ;
#35089=CARTESIAN_POINT ( 'NONE',  ( 5.004475574535000248, 1517.026025493960105, 201.3999380438669959 ) ) ;
#35093=EDGE_CURVE ( 'NONE', #39742, #89306, #37721, .T. ) ;
#35116=CARTESIAN_POINT ( 'NONE',  ( -8.324963436393932881, 1511.468585895425122, 214.5031578665083600 ) ) ;
#35124=CARTESIAN_POINT ( 'NONE',  ( -1.713660193710039970, 1516.545910801970194, 201.4125102895399948 ) ) ;
#35130=ORIENTED_EDGE ( 'NONE', *, *, #1154, .F. ) ;
#35148=CARTESIAN_POINT ( 'NONE',  ( -1.906499846882070084E-08, 1517.051704408389924, 201.3992656178269840 ) ) ;
#35167=CARTESIAN_POINT ( 'NONE',  ( -6.550870182235000172, 1516.727502608469877, 209.8762341530540141 ) ) ;
#35186=CARTESIAN_POINT ( 'NONE',  ( -5.788691363644999477, 1517.157901477309906, 207.9987443536870160 ) ) ;
#35202=CARTESIAN_POINT ( 'NONE',  ( 1.119717716265000051, 1517.038650117239968, 205.6590103047369951 ) ) ;
#35205=CARTESIAN_POINT ( 'NONE',  ( -4.752602823847894342, 1516.784510156630176, 203.3028915219003636 ) ) ;
#35254=CARTESIAN_POINT ( 'NONE',  ( 6.947377783174999877, 1517.009964551830080, 213.7374907746170152 ) ) ;
#35292=CARTESIAN_POINT ( 'NONE',  ( -5.651514362218461152, 1516.808499252805632, 214.0555898242563444 ) ) ;
#35296=CARTESIAN_POINT ( 'NONE',  ( 2.476450664134999702, 1516.843453247299749, 206.8221896160070230 ) ) ;
#35302=ORIENTED_EDGE ( 'NONE', *, *, #19892, .T. ) ;
#35309=CARTESIAN_POINT ( 'NONE',  ( 2.492443650904999863, 1516.793978928989873, 212.3737347995770222 ) ) ;
#35310=B_SPLINE_CURVE_WITH_KNOTS ( 'NONE', 5,
 ( #18404, #79452, #79995, #11152, #88937, #88396, #29047, #44760, #12228 ),
 .UNSPECIFIED., .F., .F.,
 ( 6, 3, 6 ),
 ( 0.8631819992775470185, 2.053866004900000153, 3.194082035662300090 ),
 .UNSPECIFIED. ) ;
#35339=CARTESIAN_POINT ( 'NONE',  ( 2.483322453895000059, 1517.139039350860003, 202.5585910412470128 ) ) ;
#35340=CARTESIAN_POINT ( 'NONE',  ( -4.618583430005000601, 1516.939762005280045, 209.1349059721700030 ) ) ;
#35343=CARTESIAN_POINT ( 'NONE',  ( 5.513435558552499671, 1508.603735221732222, 201.8522301334030544 ) ) ;
#35345=DIRECTION ( 'NONE',  ( 0.6742693640212139572, -4.299109996486529694E-13, 0.7384854939282339270 ) ) ;
#35346=EDGE_CURVE ( 'NONE', #49664, #7555, #35376, .T. ) ;
#35362=FACE_OUTER_BOUND ( 'NONE', #89831, .T. ) ;
#35376=LINE ( 'NONE', #33707, #2161 ) ;
#35378=CARTESIAN_POINT ( 'NONE',  ( -15.31485522056499882, 1513.484013041540038, 223.6897698068669911 ) ) ;
#35383=CARTESIAN_POINT ( 'NONE',  ( 2.864972116015000125, 1516.859514182039902, 206.2412530031170093 ) ) ;
#35401=CARTESIAN_POINT ( 'NONE',  ( -2.766744960634999639, 1511.930588878439949, 201.4376028569870130 ) ) ;
#35426=CARTESIAN_POINT ( 'NONE',  ( -5.513207816801510397, 1508.731180391289854, 216.5668095923579983 ) ) ;
#35435=CARTESIAN_POINT ( 'NONE',  ( 2.286446325635000054, 1517.042661899400173, 204.4961520670869959 ) ) ;
#35440=DIRECTION ( 'NONE',  ( 0.000000000000000000, -0.02617694830788830015, 0.9996573249755569268 ) ) ;
#35447=ORIENTED_EDGE ( 'NONE', *, *, #83922, .T. ) ;
#35458=CARTESIAN_POINT ( 'NONE',  ( -2.282915221395000138, 1516.876240617270014, 211.6158662526670184 ) ) ;
#35461=CARTESIAN_POINT ( 'NONE',  ( 7.641097577974999666, 1512.520476835130012, 202.3618328102370185 ) ) ;
#35467=CARTESIAN_POINT ( 'NONE',  ( -7.284055456385000404, 1511.816633140279919, 215.8034048803770020 ) ) ;
#35470=CARTESIAN_POINT ( 'NONE',  ( -2.872836660654999985, 1517.158319634930194, 216.8472181024670249 ) ) ;
#35477=CARTESIAN_POINT ( 'NONE',  ( 6.546302742015000398, 1516.577434278289957, 206.6347425125669872 ) ) ;
#35482=CARTESIAN_POINT ( 'NONE',  ( -6.455481540323650513, 1508.551704606160001, 202.2941615582640225 ) ) ;
#35493=CARTESIAN_POINT ( 'NONE',  ( 6.557909882634999299, 1516.908489800550115, 214.8995913655070069 ) ) ;
#35500=CARTESIAN_POINT ( 'NONE',  ( -7.708770045145000083, 1516.524310051880093, 211.4128934593470035 ) ) ;
#35507=CARTESIAN_POINT ( 'NONE',  ( -8.598884509784999963, 1512.314860040240092, 211.3567694112070114 ) ) ;
#35517=CARTESIAN_POINT ( 'NONE',  ( 6.937965660314999283, 1516.732530461250008, 204.1161457306970135 ) ) ;
#35527=DIRECTION ( 'NONE',  ( -0.9996573249754487911, 0.02617694831201757000, 1.257327575352784523E-11 ) ) ;
#35588=ORIENTED_EDGE ( 'NONE', *, *, #12098, .T. ) ;
#35593=CARTESIAN_POINT ( 'NONE',  ( -1.120543735785000106, 1517.073005577650065, 213.1661658574570026 ) ) ;
#35594=CARTESIAN_POINT ( 'NONE',  ( 3.853756123904999775, 1510.775363762149937, 216.6800758355570053 ) ) ;
#35598=CARTESIAN_POINT ( 'NONE',  ( 1.706797785944999868, 1517.164987839469859, 203.3324512698969784 ) ) ;
#35610=CARTESIAN_POINT ( 'NONE',  ( 7.724732408895000013, 1517.133889586189980, 212.3822030989969960 ) ) ;
#35616=CARTESIAN_POINT ( 'NONE',  ( -5.788691363644999477, 1517.157901477309906, 207.9987443536870160 ) ) ;
#35633=CARTESIAN_POINT ( 'NONE',  ( -6.939219520934999608, 1516.783701990830195, 214.9027072062869763 ) ) ;
#35636=CARTESIAN_POINT ( 'NONE',  ( 2.872700517194999748, 1516.559109716219837, 216.8315272385270021 ) ) ;
#35646=CARTESIAN_POINT ( 'NONE',  ( 7.395102123895940238, 1511.068351247050032, 202.7464954504410173 ) ) ;
#35658=CARTESIAN_POINT ( 'NONE',  ( 6.036759152895515790, 1509.035273823006037, 201.6612097352038120 ) ) ;
#35659=ORIENTED_EDGE ( 'NONE', *, *, #81716, .F. ) ;
#35725=CARTESIAN_POINT ( 'NONE',  ( 5.013429356055000063, 1517.123342927159911, 210.2437967141769946 ) ) ;
#35743=CARTESIAN_POINT ( 'NONE',  ( 6.935801261535000428, 1516.621991115350056, 207.9918434378369909 ) ) ;
#35753=VECTOR ( 'NONE', #25981, 1000.000000000000000 ) ;
#35761=CARTESIAN_POINT ( 'NONE',  ( 1.119439089684999944, 1517.026534522949987, 205.8528207963470038 ) ) ;
#35782=CARTESIAN_POINT ( 'NONE',  ( -6.936398393775000670, 1516.667393516340098, 213.1585948090369698 ) ) ;
#35793=VECTOR ( 'NONE', #73502, 1000.000000000000000 ) ;
#35806=CARTESIAN_POINT ( 'NONE',  ( -7.112124026466545068, 1509.032357789247726, 202.3798027825555153 ) ) ;
#35814=CARTESIAN_POINT ( 'NONE',  ( -4.029572678834999699, 1516.858649670339901, 213.1633184439769764 ) ) ;
#35818=EDGE_LOOP ( 'NONE', ( #56301, #8528, #74461, #103376 ) ) ;
#35827=DIRECTION ( 'NONE',  ( -8.596382804469569442E-17, 1.000000000000000000, 0.000000000000000000 ) ) ;
#35829=( NAMED_UNIT ( * ) SI_UNIT ( $, .STERADIAN. ) SOLID_ANGLE_UNIT ( ) );
#35834=CARTESIAN_POINT ( 'NONE',  ( 4.487249753905000027, 1509.038615934239942, 209.1727295022979831 ) ) ;
#35861=CARTESIAN_POINT ( 'NONE',  ( 4.995725969715000048, 1516.651306816259876, 206.8263604310569690 ) ) ;
#35874=CARTESIAN_POINT ( 'NONE',  ( -4.027051443935000030, 1516.733363207009916, 211.6130343286269806 ) ) ;
#35885=EDGE_CURVE ( 'NONE', #323, #28577, #80789, .T. ) ;
#35898=CARTESIAN_POINT ( 'NONE',  ( 6.120117875752820957, 1508.729257035799947, 201.6787668059709802 ) ) ;
#35902=CARTESIAN_POINT ( 'NONE',  ( -6.556651409415000131, 1516.858146885269889, 202.5689485651570010 ) ) ;
#35903=CARTESIAN_POINT ( 'NONE',  ( 4.044319887224999910, 1517.073005577650065, 210.2423896678870108 ) ) ;
#35933=ORIENTED_EDGE ( 'NONE', *, *, #39179, .T. ) ;
#35943=CARTESIAN_POINT ( 'NONE',  ( -16.21241003196499975, 1514.452905717119847, 224.0491558541669974 ) ) ;
#35947=CARTESIAN_POINT ( 'NONE',  ( -2.880592967115000125, 1516.859514182039902, 206.2568738160869941 ) ) ;
#35969=CARTESIAN_POINT ( 'NONE',  ( 16.67046851633390148, 1516.551188146170034, 222.1952932998519827 ) ) ;
#35989=CARTESIAN_POINT ( 'NONE',  ( -7.443079168794310085, 1508.729257029040127, 215.2419651647340118 ) ) ;
#35998=CARTESIAN_POINT ( 'NONE',  ( 3.255340926295000159, 1516.962555622980062, 204.4977466407669908 ) ) ;
#36022=CARTESIAN_POINT ( 'NONE',  ( -7.709681306425000713, 1516.559109716219837, 211.9945464874270158 ) ) ;
#36027=VERTEX_POINT ( 'NONE', #91987 ) ;
#36042=DIRECTION ( 'NONE',  ( 1.734723475976998196E-15, -1.000000000000000000, 0.000000000000000000 ) ) ;
#36046=CARTESIAN_POINT ( 'NONE',  ( 4.027697225915000345, 1516.766397346390022, 206.2431526829570032 ) ) ;
#36051=CARTESIAN_POINT ( 'NONE',  ( -6.032830782151830107, 1508.551567431860121, 201.9555811633020141 ) ) ;
#36057=DIRECTION ( 'NONE',  ( -0.7071093782156816498, -3.166819169022306488E-06, -0.7071041841407837980 ) ) ;
#36062=CARTESIAN_POINT ( 'NONE',  ( 2.875850094215000041, 1516.647618671360078, 214.8936433964170192 ) ) ;
#36065=CARTESIAN_POINT ( 'NONE',  ( 5.745732791923909843, 1511.535603804869879, 217.7226386876670006 ) ) ;
#36067=CARTESIAN_POINT ( 'NONE',  ( 1.716392741775000008, 1516.788317650260069, 211.9856338259669997 ) ) ;
#36084=CARTESIAN_POINT ( 'NONE',  ( -2.875850132345000087, 1516.647618671360078, 203.3500485059169876 ) ) ;
#36158=CARTESIAN_POINT ( 'NONE',  ( 3.458526497885000328, 1516.742629295279812, 214.1194197574270106 ) ) ;
#36159=CARTESIAN_POINT ( 'NONE',  ( 4.827505427815000694, 1511.354819475749991, 217.2927421938970269 ) ) ;
#36163=CARTESIAN_POINT ( 'NONE',  ( 2.480813884984999884, 1517.051603658920158, 204.1089070683270279 ) ) ;
#36166=CARTESIAN_POINT ( 'NONE',  ( -2.564633821555000193, 1511.308638870219966, 201.5496530815769916 ) ) ;
#36178=CARTESIAN_POINT ( 'NONE',  ( -2.864972154145000172, 1516.859514182039902, 212.0024388992169975 ) ) ;
#36184=CARTESIAN_POINT ( 'NONE',  ( 0.007128837152181529378, 1517.006509894990131, 209.8686634857439799 ) ) ;
#36198=CARTESIAN_POINT ( 'NONE',  ( -2.288357445734999995, 1517.116049120239950, 214.9102823043970147 ) ) ;
#36200=CARTESIAN_POINT ( 'NONE',  ( -7.722580352405000070, 1517.051704408389924, 209.1218459511669892 ) ) ;
#36201=CARTESIAN_POINT ( 'NONE',  ( 2.291047489114999891, 1516.524310051880093, 216.8306159772470210 ) ) ;
#36208=CARTESIAN_POINT ( 'NONE',  ( 8.553070074608509543, 1511.487400615810202, 203.5546195846039836 ) ) ;
#36234=CARTESIAN_POINT ( 'NONE',  ( -1.764278193548540097, 1516.541781377969983, 201.4126184223130167 ) ) ;
#36271=VERTEX_POINT ( 'NONE', #67916 ) ;
#36274=CARTESIAN_POINT ( 'NONE',  ( 1.133653140995000141, 1516.978425811520083, 209.8592968530090275 ) ) ;
#36275=CARTESIAN_POINT ( 'NONE',  ( 7.012921545474999796, 1508.551704408389924, 203.6084103740869864 ) ) ;
#36279=ORIENTED_EDGE ( 'NONE', *, *, #64845, .F. ) ;
#36289=CARTESIAN_POINT ( 'NONE',  ( -5.789394700334999477, 1517.164987839469859, 207.4150481461570052 ) ) ;
#36293=ORIENTED_EDGE ( 'NONE', *, *, #38046, .T. ) ;
#36299=LINE ( 'NONE', #71613, #100205 ) ;
#36305=CARTESIAN_POINT ( 'NONE',  ( 6.547556931335000385, 1516.633288330999903, 205.8595812817970057 ) ) ;
#36310=CARTESIAN_POINT ( 'NONE',  ( 4.545982209787698736, 1508.783371651607240, 212.6094383991669474 ) ) ;
#36322=CARTESIAN_POINT ( 'NONE',  ( 3.264778779384999829, 1516.727068157269969, 214.1190961241369735 ) ) ;
#36394=CARTESIAN_POINT ( 'NONE',  ( -5.931260097829800237, 1516.766044797163204, 213.7134053296210823 ) ) ;
#36397=CARTESIAN_POINT ( 'NONE',  ( -5.788436372295000076, 1517.116049120239950, 206.8334885244969712 ) ) ;
#36408=CARTESIAN_POINT ( 'NONE',  ( 3.461995158685000185, 1516.906233342200039, 211.9877574868770012 ) ) ;
#36418=CARTESIAN_POINT ( 'NONE',  ( 15.00581739583218521, 1514.742486326955941, 225.2136390995225383 ) ) ;
#36430=CARTESIAN_POINT ( 'NONE',  ( 7.443079130664420617, 1508.729257029040127, 203.0017267375970107 ) ) ;
#36434=CARTESIAN_POINT ( 'NONE',  ( -2.874588960795000148, 1516.606339319019980, 202.5748942495170013 ) ) ;
#36435=CARTESIAN_POINT ( 'NONE',  ( -2.868112169295000236, 1516.855632454399938, 209.8795095036720113 ) ) ;
#36439=CARTESIAN_POINT ( 'NONE',  ( 5.513435558552499671, 1509.038615934029849, 201.6090957240569992 ) ) ;
#36458=CARTESIAN_POINT ( 'NONE',  ( -6.479185156475000262, 1511.503799556569902, 201.7413190995169998 ) ) ;
#36476=CARTESIAN_POINT ( 'NONE',  ( 12.04512424413499971, 1511.810036768419877, 224.5882503546669682 ) ) ;
#36486=CARTESIAN_POINT ( 'NONE',  ( 6.546302742015000398, 1516.577434278289957, 206.6347425125669872 ) ) ;
#36489=DIRECTION ( 'NONE',  ( -1.000000000000000000, 0.000000000000000000, 0.000000000000000000 ) ) ;
#36532=DIRECTION ( 'NONE',  ( -0.02616798426500960631, 0.9993150019883682011, -0.02616798426500970345 ) ) ;
#36541=CARTESIAN_POINT ( 'NONE',  ( -0.7560907659159991079, 1516.770163853809890, 204.1215159365669933 ) ) ;
#36562=CARTESIAN_POINT ( 'NONE',  ( -4.027697264044999947, 1516.766397346390022, 212.0005392193770035 ) ) ;
#36572=CARTESIAN_POINT ( 'NONE',  ( -8.375502483594999603, 1512.383155430640045, 215.8646805558269932 ) ) ;
#36573=CARTESIAN_POINT ( 'NONE',  ( 15.90990255763500016, 1512.830284628050094, 198.1616908427670296 ) ) ;
#36584=CARTESIAN_POINT ( 'NONE',  ( 2.864043418315000089, 1516.811292230880099, 206.8228319013669818 ) ) ;
#36590=CARTESIAN_POINT ( 'NONE',  ( -6.081362942748859801, 1508.610509101569960, 201.8017925879439929 ) ) ;
#36602=CARTESIAN_POINT ( 'NONE',  ( 1.130607463874999885, 1516.632821972880038, 215.6700465578769865 ) ) ;
#36606=CARTESIAN_POINT ( 'NONE',  ( -2.864972154145000172, 1516.859514182039902, 212.0024388992169975 ) ) ;
#36626=CARTESIAN_POINT ( 'NONE',  ( 2.287084270065000258, 1517.068517094990057, 204.1085709707169826 ) ) ;
#36658=ADVANCED_FACE ( 'NONE', ( #66000 ), #83971, .T. ) ;
#36663=VERTEX_POINT ( 'NONE', #94753 ) ;
#36672=CARTESIAN_POINT ( 'NONE',  ( 6.942354273414999888, 1516.905946377369901, 201.4030824261969883 ) ) ;
#36685=CARTESIAN_POINT ( 'NONE',  ( -7.558229903455000454, 1510.775363762149937, 212.9756020941370309 ) ) ;
#36690=( NAMED_UNIT ( * ) SI_UNIT ( $, .STERADIAN. ) SOLID_ANGLE_UNIT ( ) );
#36699=VERTEX_POINT ( 'NONE', #28101 ) ;
#36703=CARTESIAN_POINT ( 'NONE',  ( -2.480813923114999930, 1517.051603658920158, 214.1347848340070072 ) ) ;
#36704=CARTESIAN_POINT ( 'NONE',  ( 2.698112791424999823, 1512.326491219019999, 216.8133626242469916 ) ) ;
#36711=CARTESIAN_POINT ( 'NONE',  ( -2.297085753945000253, 1516.718889242609976, 205.0950684461469962 ) ) ;
#36716=CARTESIAN_POINT ( 'NONE',  ( 4.616899834755000320, 1517.050041317280147, 201.3993091674070115 ) ) ;
#36726=CARTESIAN_POINT ( 'NONE',  ( 5.786837678925000006, 1517.040132827679827, 212.3790665729270017 ) ) ;
#36732=CARTESIAN_POINT ( 'NONE',  ( -2.292217048824999992, 1516.941178807709775, 209.1350424789999920 ) ) ;
#36739=DIRECTION ( 'NONE',  ( 0.4770263929449307105, 0.7067418228238977473, 0.5224574779879248565 ) ) ;
#36747=CARTESIAN_POINT ( 'NONE',  ( -4.615017365965000451, 1516.987478262539980, 215.6816440265270103 ) ) ;
#36758=CARTESIAN_POINT ( 'NONE',  ( 7.536818026188599973, 1511.326458810320219, 202.9508713580690085 ) ) ;
#36766=EDGE_CURVE ( 'NONE', #56739, #64419, #73433, .T. ) ;
#36787=CARTESIAN_POINT ( 'NONE',  ( -1.606066254855309960, 1516.556413965820184, 201.4122352545150250 ) ) ;
#36831=CARTESIAN_POINT ( 'NONE',  ( -7.332063977575000280, 1516.939491476980038, 209.1325772641960157 ) ) ;
#36844=CARTESIAN_POINT ( 'NONE',  ( 7.713648834184999359, 1516.710624944440042, 208.3691743819339877 ) ) ;
#36860=CARTESIAN_POINT ( 'NONE',  ( 6.933879402874999265, 1516.560253536979872, 206.6353711893569880 ) ) ;
#36864=ORIENTED_EDGE ( 'NONE', *, *, #62570, .F. ) ;
#36876=CARTESIAN_POINT ( 'NONE',  ( -7.713117841115000317, 1516.690345681169902, 214.1262880092169780 ) ) ;
#36899=CARTESIAN_POINT ( 'NONE',  ( -7.512705432752817991, 1509.036904581754015, 203.3466808530631909 ) ) ;
#36943=CARTESIAN_POINT ( 'NONE',  ( -2.881222795715000284, 1516.891731298979948, 206.6444723262370076 ) ) ;
#36950=ORIENTED_EDGE ( 'NONE', *, *, #105003, .T. ) ;
#36957=CARTESIAN_POINT ( 'NONE',  ( 0.7576635334400020350, 1516.855632454399938, 211.9899581013969794 ) ) ;
#36979=CARTESIAN_POINT ( 'NONE',  ( 7.266079630789520571, 1509.032014039220030, 202.3522229272149957 ) ) ;
#36986=CARTESIAN_POINT ( 'NONE',  ( 3.449777315724999571, 1516.974592746400049, 204.1104779853070283 ) ) ;
#36987=ORIENTED_EDGE ( 'NONE', *, *, #13146, .T. ) ;
#37009=CARTESIAN_POINT ( 'NONE',  ( -8.118882966355000619, 1514.642928591840018, 202.5872254880569869 ) ) ;
#37033=CARTESIAN_POINT ( 'NONE',  ( 7.708745647785000266, 1516.523379810429788, 207.4137536659370085 ) ) ;
#37052=CARTESIAN_POINT ( 'NONE',  ( -2.698112829555000314, 1512.326491219019999, 201.4303292780870152 ) ) ;
#37057=CARTESIAN_POINT ( 'NONE',  ( 17.05938516367379876, 1517.051704408300111, 223.0487112149370148 ) ) ;
#37059=VECTOR ( 'NONE', #21710, 1000.000000000000114 ) ;
#37084=DIRECTION ( 'NONE',  ( -0.6742693640212139572, -4.521919481779819710E-17, -0.7384854939282339270 ) ) ;
#37089=CARTESIAN_POINT ( 'NONE',  ( -4.039897316195000698, 1516.787536375099990, 204.1233307748069876 ) ) ;
#37103=ADVANCED_FACE ( 'NONE', ( #6745 ), #15671, .T. ) ;
#37112=CARTESIAN_POINT ( 'NONE',  ( 5.786527562335000319, 1517.025653221279981, 212.5728793591970032 ) ) ;
#37115=( BOUNDED_CURVE ( )  B_SPLINE_CURVE ( 3, ( #53974, #3012, #37134, #105447 ),
 .UNSPECIFIED., .F., .T. ) 
 B_SPLINE_CURVE_WITH_KNOTS ( ( 4, 4 ),
 ( 1.969431562482085677E-12, 0.4510268114855934263 ),
 .UNSPECIFIED. ) 
 CURVE ( )  GEOMETRIC_REPRESENTATION_ITEM ( )  RATIONAL_B_SPLINE_CURVE ( ( 1.000000000000000000, 0.9831196230105669898, 0.9831196230105669898, 1.000000000000000000 ) ) 
 REPRESENTATION_ITEM ( '' )  );
#37134=CARTESIAN_POINT ( 'NONE',  ( -4.151444337083049163, 1516.720891557477444, 217.8757000259121810 ) ) ;
#37138=CARTESIAN_POINT ( 'NONE',  ( 1.700259675955000160, 1516.898441858519845, 207.4036424686470070 ) ) ;
#37143=CARTESIAN_POINT ( 'NONE',  ( -5.513261715040130184, 1508.551704609589933, 202.1093729265590184 ) ) ;
#37160=CARTESIAN_POINT ( 'NONE',  ( -2.483322492024999661, 1517.139039350860003, 215.6851008610869940 ) ) ;
#37165=CARTESIAN_POINT ( 'NONE',  ( -1.701729858475000023, 1516.969638403840008, 212.0041719496170174 ) ) ;
#37169=ORIENTED_EDGE ( 'NONE', *, *, #57263, .F. ) ;
#37182=CARTESIAN_POINT ( 'NONE',  ( -3.264778817514999876, 1516.727068157269969, 204.1245957781970048 ) ) ;
#37219=CARTESIAN_POINT ( 'NONE',  ( 6.774723932182340036, 1511.035127054690065, 217.4331360664359920 ) ) ;
#37222=CARTESIAN_POINT ( 'NONE',  ( -11.28295023116499962, 1512.609537213029853, 192.8912262721669890 ) ) ;
#37227=CARTESIAN_POINT ( 'NONE',  ( 5.779627054084999216, 1516.977993847330026, 201.4011957967969977 ) ) ;
#37231=CARTESIAN_POINT ( 'NONE',  ( 7.621419120635000155, 1512.021995456199875, 206.5558387662869961 ) ) ;
#37237=LINE ( 'NONE', #89832, #109954 ) ;
#37240=CARTESIAN_POINT ( 'NONE',  ( -7.985842396434999380, 1511.355055856609852, 213.1582267177570031 ) ) ;
#37262=CARTESIAN_POINT ( 'NONE',  ( -1.706797824074999914, 1517.164987839469859, 214.9112406324369999 ) ) ;
#37263=CARTESIAN_POINT ( 'NONE',  ( 2.625066769795000088, 1511.873873588870083, 216.7407507270369820 ) ) ;
#37272=CARTESIAN_POINT ( 'NONE',  ( -5.009478105444999940, 1516.886345593249871, 204.5093386581970094 ) ) ;
#37286=CARTESIAN_POINT ( 'NONE',  ( 7.335900995594999863, 1517.068717944079935, 213.1567545299469657 ) ) ;
#37292=CARTESIAN_POINT ( 'NONE',  ( -4.031168805994999715, 1516.805675336850072, 209.8787446699039947 ) ) ;
#37305=CARTESIAN_POINT ( 'NONE',  ( 2.875850094215000041, 1516.647618671360078, 214.8936433964170192 ) ) ;
#37316=CARTESIAN_POINT ( 'NONE',  ( 7.482857888537069790, 1511.023286695659863, 202.9712329530480019 ) ) ;
#37368=ORIENTED_EDGE ( 'NONE', *, *, #98695, .T. ) ;
#37375=EDGE_CURVE ( 'NONE', #39203, #38027, #43548, .T. ) ;
#37385=CARTESIAN_POINT ( 'NONE',  ( -1.117840124865000062, 1516.949031626070109, 210.8389850543470061 ) ) ;
#37395=CARTESIAN_POINT ( 'NONE',  ( 2.872208710164999790, 1517.145312756229941, 201.7840522196070197 ) ) ;
#37402=CARTESIAN_POINT ( 'NONE',  ( 2.486220101774999858, 1516.939658295650133, 209.1086089184300079 ) ) ;
#37416=VECTOR ( 'NONE', #63115, 1000.000000000000114 ) ;
#37420=CARTESIAN_POINT ( 'NONE',  ( 6.933616821004999764, 1516.548716157039962, 206.8295387017270173 ) ) ;
#37438=CARTESIAN_POINT ( 'NONE',  ( -2.869693497065000098, 1517.070197312179971, 214.9093229647470196 ) ) ;
#37468=CARTESIAN_POINT ( 'NONE',  ( -4.491293135916502699, 1508.884207228266632, 212.6094329811311354 ) ) ;
#37503=CARTESIAN_POINT ( 'NONE',  ( -7.725990199955000470, 1517.181921232829836, 206.6366402828969910 ) ) ;
#37527=CARTESIAN_POINT ( 'NONE',  ( 11.56080089750725115, 1512.916366990813913, 225.4987921079732018 ) ) ;
#37545=CARTESIAN_POINT ( 'NONE',  ( 6.549762446985000430, 1516.729202374750002, 204.5030968636170030 ) ) ;
#37548=B_SPLINE_CURVE_WITH_KNOTS ( 'NONE', 5,
 ( #53495, #18744, #339, #10360, #102209, #94925 ),
 .UNSPECIFIED., .F., .F.,
 ( 6, 6 ),
 ( 0.000000000000000000, 1.000000000000000000 ),
 .UNSPECIFIED. ) ;
#37567=CARTESIAN_POINT ( 'NONE',  ( -7.521073069125000288, 1513.760531203550045, 202.2873616486669732 ) ) ;
#37568=ORIENTED_EDGE ( 'NONE', *, *, #108341, .T. ) ;
#37580=CARTESIAN_POINT ( 'NONE',  ( 14.10835366113500022, 1513.596256836700150, 225.7720208619669791 ) ) ;
#37586=CARTESIAN_POINT ( 'NONE',  ( -0.4346943098025670138, 1517.051704408590012, 216.8444262844809884 ) ) ;
#37589=CARTESIAN_POINT ( 'NONE',  ( -3.269184946495000244, 1516.940296199220029, 206.8376465686969823 ) ) ;
#37604=CARTESIAN_POINT ( 'NONE',  ( 9.813597453882589861, 1516.551188145990182, 214.6853868983759810 ) ) ;
#37609=CARTESIAN_POINT ( 'NONE',  ( 6.191282256226939396, 1510.848430436206854, 216.5799282118206008 ) ) ;
#37640=VECTOR ( 'NONE', #47146, 1000.000000000000114 ) ;
#37642=DIRECTION ( 'NONE',  ( -0.8236474686107853049, 0.5669078173018522460, -0.01484500364079620674 ) ) ;
#37644=CARTESIAN_POINT ( 'NONE',  ( -6.559168674874999105, 1516.960844870249957, 204.1192525727769862 ) ) ;
#37652=VERTEX_POINT ( 'NONE', #22161 ) ;
#37665=CARTESIAN_POINT ( 'NONE',  ( -1.119439127814999990, 1517.026534522949987, 212.3908711059869745 ) ) ;
#37667=AXIS2_PLACEMENT_3D ( 'NONE', #40760, #66548, #109625 ) ;
#37675=CARTESIAN_POINT ( 'NONE',  ( -6.096095868995000444, 1514.881364185380107, 217.1628748908970010 ) ) ;
#37676=CARTESIAN_POINT ( 'NONE',  ( 16.53526709313100795, 1514.188985849830942, 194.8337175523576548 ) ) ;
#37685=VERTEX_POINT ( 'NONE', #90493 ) ;
#37686=CARTESIAN_POINT ( 'NONE',  ( -0.01265822594359850006, 1516.959716008189844, 207.4120794380770292 ) ) ;
#37693=CARTESIAN_POINT ( 'NONE',  ( -7.166264985072499982, 1508.551567432899901, 203.0889892476990042 ) ) ;
#37707=CARTESIAN_POINT ( 'NONE',  ( 1.710004548794999968, 1516.557392317769882, 215.6678473207969944 ) ) ;
#37709=CARTESIAN_POINT ( 'NONE',  ( 5.567226347498220207, 1511.487400615810202, 217.6749160448409839 ) ) ;
#37711=CARTESIAN_POINT ( 'NONE',  ( -7.709032175815000443, 1516.534320418310244, 211.6070631641669877 ) ) ;
#37721=LINE ( 'NONE', #105483, #79047 ) ;
#37728=CARTESIAN_POINT ( 'NONE',  ( -2.296124889065000119, 1516.677239312369920, 204.5136991508470032 ) ) ;
#37742=EDGE_CURVE ( 'NONE', #108962, #20905, #34743, .T. ) ;
#37761=CARTESIAN_POINT ( 'NONE',  ( -4.987078460856490203, 1508.551704408389924, 212.6094383991630252 ) ) ;
#37774=CARTESIAN_POINT ( 'NONE',  ( -12.04512428226500020, 1511.810036768419877, 193.6554415476670101 ) ) ;
#37775=CARTESIAN_POINT ( 'NONE',  ( -9.258462901215001040, 1517.051704408389924, 221.5128288575669728 ) ) ;
#37776=EDGE_CURVE ( 'NONE', #64419, #90411, #102856, .T. ) ;
#37779=CARTESIAN_POINT ( 'NONE',  ( 2.291514297774999598, 1517.194972660189933, 201.3955140066269962 ) ) ;
#37783=CARTESIAN_POINT ( 'NONE',  ( 7.599227145645000903, 1512.341036949130057, 206.8869232832669809 ) ) ;
#37793=CARTESIAN_POINT ( 'NONE',  ( -7.635834400824999868, 1511.005930286180046, 213.0490718368869807 ) ) ;
#37804=ORIENTED_EDGE ( 'NONE', *, *, #87314, .F. ) ;
#37811=CARTESIAN_POINT ( 'NONE',  ( 2.487103419534999915, 1516.577434278289957, 215.6681487122470173 ) ) ;
#37812=CARTESIAN_POINT ( 'NONE',  ( 2.996785032205000032, 1512.020737142380085, 217.0152570523270015 ) ) ;
#37821=CARTESIAN_POINT ( 'NONE',  ( -2.490245952555000031, 1516.691389976299888, 204.5134284255869943 ) ) ;
#37834=CARTESIAN_POINT ( 'NONE',  ( 4.622842844184999578, 1516.901952101700090, 213.1523604828169880 ) ) ;
#37840=CARTESIAN_POINT ( 'NONE',  ( 2.873919002525000099, 1516.940252185109784, 209.1085733957019954 ) ) ;
#37851=EDGE_CURVE ( 'NONE', #27633, #78418, #78782, .T. ) ;
#37852=CARTESIAN_POINT ( 'NONE',  ( 5.614653816015000132, 1512.956339156650074, 203.5071921160869977 ) ) ;
#37855=CARTESIAN_POINT ( 'NONE',  ( 4.038637462725000127, 1516.734985836460055, 214.8955147850770118 ) ) ;
#37860=CARTESIAN_POINT ( 'NONE',  ( 5.778999773775000293, 1516.955859323880077, 201.7887757972170277 ) ) ;
#37867=CARTESIAN_POINT ( 'NONE',  ( 8.289603071667819734, 1511.655824793919919, 203.1726102367569808 ) ) ;
#37892=ADVANCED_FACE ( 'NONE', ( #51132 ), #24044, .F. ) ;
#37903=CARTESIAN_POINT ( 'NONE',  ( 13.08508097766669920, 1512.436270050390021, 224.3649262596819938 ) ) ;
#37936=CARTESIAN_POINT ( 'NONE',  ( -13.07344736774610183, 1516.551188146160030, 225.7923144865690119 ) ) ;
#37944=CARTESIAN_POINT ( 'NONE',  ( 0.7579262867720020225, 1516.927039499179955, 210.8260166843570005 ) ) ;
#37952=CARTESIAN_POINT ( 'NONE',  ( -3.454748846324999789, 1516.609912606490070, 201.7988116581369979 ) ) ;
#37961=VERTEX_POINT ( 'NONE', #12276 ) ;
#37971=CARTESIAN_POINT ( 'NONE',  ( -3.461995196814999787, 1516.906233342200039, 206.2559344154570056 ) ) ;
#37988=CARTESIAN_POINT ( 'NONE',  ( -5.000083865865000199, 1516.858456333729919, 214.1306941701269864 ) ) ;
#38027=VERTEX_POINT ( 'NONE', #41357 ) ;
#38046=EDGE_CURVE ( 'NONE', #9383, #17126, #6640, .T. ) ;
#38047=CARTESIAN_POINT ( 'NONE',  ( -7.266079668920959911, 1509.032014039220030, 215.8914689751280207 ) ) ;
#38057=CARTESIAN_POINT ( 'NONE',  ( -0.01265822594359850006, 1516.959716008189844, 207.4120794380770292 ) ) ;
#38062=CARTESIAN_POINT ( 'NONE',  ( 13.33054332923500063, 1520.551704408390151, 211.1218459511669892 ) ) ;
#38076=CARTESIAN_POINT ( 'NONE',  ( 14.47449472319151376, 1514.320576839395017, 225.5689061850603991 ) ) ;
#38083=ORIENTED_EDGE ( 'NONE', *, *, #57524, .F. ) ;
#38092=CARTESIAN_POINT ( 'NONE',  ( 4.031142351675000235, 1516.929569650079884, 204.1114229688670036 ) ) ;
#38096=ORIENTED_EDGE ( 'NONE', *, *, #34468, .T. ) ;
#38097=ORIENTED_EDGE ( 'NONE', *, *, #2105, .F. ) ;
#38112=CARTESIAN_POINT ( 'NONE',  ( -6.597706052855000003, 1512.335510084600173, 201.0409955017370010 ) ) ;
#38126=CARTESIAN_POINT ( 'NONE',  ( 15.02579302773500025, 1513.907445464710236, 224.5270601239670043 ) ) ;
#38133=CARTESIAN_POINT ( 'NONE',  ( -3.463767296015000330, 1517.014196759610059, 207.4190915607570105 ) ) ;
#38188=CARTESIAN_POINT ( 'NONE',  ( 1.703779605225000049, 1517.057265928030120, 205.0766634521770015 ) ) ;
#38228=CARTESIAN_POINT ( 'NONE',  ( -2.494020320564999782, 1516.876240617270014, 206.8389307488369866 ) ) ;
#38246=CARTESIAN_POINT ( 'NONE',  ( -3.452289220704999551, 1517.069378699710114, 215.6835323934670328 ) ) ;
#38250=CARTESIAN_POINT ( 'NONE',  ( -3.252530653725000054, 1516.827328999679821, 212.0018028951869837 ) ) ;
#38251=B_SPLINE_CURVE_WITH_KNOTS ( 'NONE', 5,
 ( #33389, #49129, #50234, #8743, #24982, #93308 ),
 .UNSPECIFIED., .F., .F.,
 ( 6, 6 ),
 ( 4.250950522270000143, 7.082025451739999866 ),
 .UNSPECIFIED. ) ;
#38266=ORIENTED_EDGE ( 'NONE', *, *, #60045, .F. ) ;
#38267=CARTESIAN_POINT ( 'NONE',  ( -4.040527342105000308, 1516.815231249920089, 204.5109077207270047 ) ) ;
#38295=CARTESIAN_POINT ( 'NONE',  ( 8.220025357896366458, 1511.455724274470640, 205.0451695456004870 ) ) ;
#38305=CARTESIAN_POINT ( 'NONE',  ( -13.32051257826499935, 1512.868709057579963, 192.3735960303669970 ) ) ;
#38314=CARTESIAN_POINT ( 'NONE',  ( 7.585404386385000031, 1511.813148765560072, 206.6464469953870093 ) ) ;
#38325=CARTESIAN_POINT ( 'NONE',  ( -8.370529003654999300, 1511.388520542559945, 213.6642613602169831 ) ) ;
#38344=CARTESIAN_POINT ( 'NONE',  ( -5.776491133374999976, 1516.858301627840092, 214.9045953718370185 ) ) ;
#38352=CARTESIAN_POINT ( 'NONE',  ( 6.549762446985000430, 1516.729202374750002, 204.5030968636170030 ) ) ;
#38368=CARTESIAN_POINT ( 'NONE',  ( 2.297085715815000206, 1516.718889242609976, 213.1486234561869821 ) ) ;
#38373=DIRECTION ( 'NONE',  ( 0.000000000000000000, 1.000000000000000000, -6.123233995736769734E-17 ) ) ;
#38374=CARTESIAN_POINT ( 'NONE',  ( -7.715452159899959916, 1516.779489719169987, 209.6579840536579979 ) ) ;
#38375=CARTESIAN_POINT ( 'NONE',  ( -7.713648872314999849, 1516.710624944440042, 209.8745175203999906 ) ) ;
#38390=CARTESIAN_POINT ( 'NONE',  ( 7.718134629434999283, 1516.881930554049859, 216.4517759834270123 ) ) ;
#38395=CARTESIAN_POINT ( 'NONE',  ( -5.780232115465000042, 1516.760434454289907, 201.7950504087270076 ) ) ;
#38396=CARTESIAN_POINT ( 'NONE',  ( -15.52404079726500008, 1511.843510977570077, 220.5312950707669870 ) ) ;
#38398=CARTESIAN_POINT ( 'NONE',  ( -14.72576942166499947, 1512.123542805230272, 221.3115653187670091 ) ) ;
#38427=CARTESIAN_POINT ( 'NONE',  ( -0.4998264653690069892, 1516.789754148840075, 201.4061250449829856 ) ) ;
#38431=CARTESIAN_POINT ( 'NONE',  ( 12.77505761545979901, 1512.281672892750066, 224.2544213742990280 ) ) ;
#38475=CARTESIAN_POINT ( 'NONE',  ( 0.7579843820170020230, 1516.883361325900069, 211.4083188566570186 ) ) ;
#38482=EDGE_CURVE ( 'NONE', #39998, #46912, #66870, .T. ) ;
#38483=CARTESIAN_POINT ( 'NONE',  ( -5.780232115465000042, 1516.760434454289907, 201.7950504087270076 ) ) ;
#38487=ORIENTED_EDGE ( 'NONE', *, *, #40792, .F. ) ;
#38499=CARTESIAN_POINT ( 'NONE',  ( 5.788691325514999875, 1517.157901477309906, 210.2449475486469908 ) ) ;
#38505=CARTESIAN_POINT ( 'NONE',  ( 7.567811368475000577, 1511.141271963160079, 206.0724820029969919 ) ) ;
#38506=CARTESIAN_POINT ( 'NONE',  ( 2.283570633165000086, 1516.909589401870107, 206.2402975076569760 ) ) ;
#38514=DIRECTION ( 'NONE',  ( -1.000000000000000000, 0.000000000000000000, 0.000000000000000000 ) ) ;
#38523=CARTESIAN_POINT ( 'NONE',  ( 6.944231748164999551, 1516.882690742909972, 215.6753703478370028 ) ) ;
#38526=CARTESIAN_POINT ( 'NONE',  ( 7.709052374754190140, 1516.535093240819833, 207.2584636299989995 ) ) ;
#38567=CARTESIAN_POINT ( 'NONE',  ( -3.330134203884999700, 1515.051704408389924, 213.4516374609670208 ) ) ;
#38568=EDGE_CURVE ( 'NONE', #65245, #3729, #59948, .T. ) ;
#38578=ORIENTED_EDGE ( 'NONE', *, *, #68769, .F. ) ;
#38593=CARTESIAN_POINT ( 'NONE',  ( -5.013429394184999666, 1517.123342927159911, 207.9998951881570122 ) ) ;
#38601=AXIS2_PLACEMENT_3D ( 'NONE', #40152, #13826, #31196 ) ;
#38612=CARTESIAN_POINT ( 'NONE',  ( -7.734617125744999377, 1516.863303996349941, 216.9435780305869912 ) ) ;
#38616=CARTESIAN_POINT ( 'NONE',  ( 14.30575996553655038, 1514.201209518706264, 225.6492543780247502 ) ) ;
#38635=CARTESIAN_POINT ( 'NONE',  ( -3.263521942484999716, 1516.676340709600026, 203.3494421577970002 ) ) ;
#38644=CARTESIAN_POINT ( 'NONE',  ( -14.56186263597409969, 1513.645442088330128, 194.0527955301810152 ) ) ;
#38657=CARTESIAN_POINT ( 'NONE',  ( -7.101217506704999849, 1512.693483295299984, 200.8135970150769936 ) ) ;
#38671=CARTESIAN_POINT ( 'NONE',  ( 14.56792383663499990, 1513.484013041540038, 224.4367011526669842 ) ) ;
#38677=CARTESIAN_POINT ( 'NONE',  ( -6.563595907815000352, 1517.154223579619838, 206.8322214998769937 ) ) ;
#38695=ORIENTED_EDGE ( 'NONE', *, *, #22655, .F. ) ;
#38717=CARTESIAN_POINT ( 'NONE',  ( 3.487592431178331953, 1508.551704408389469, 204.2634855480304452 ) ) ;
#38724=CARTESIAN_POINT ( 'NONE',  ( -3.547807590152150414, 1511.610022727348223, 201.0686036343854539 ) ) ;
#38728=LINE ( 'NONE', #72902, #103842 ) ;
#38732=CARTESIAN_POINT ( 'NONE',  ( 2.865911516645000212, 1516.906233342200039, 205.6598507734169914 ) ) ;
#38746=CARTESIAN_POINT ( 'NONE',  ( -5.000330033664999618, 1516.770163853809890, 209.8779366980180328 ) ) ;
#38757=ORIENTED_EDGE ( 'NONE', *, *, #5526, .F. ) ;
#38762=CARTESIAN_POINT ( 'NONE',  ( -6.439137473055000171, 1514.557408760799945, 217.0653694116970200 ) ) ;
#38763=CARTESIAN_POINT ( 'NONE',  ( 16.52212291317280446, 1514.209381233948534, 194.8043297302063195 ) ) ;
#38776=CARTESIAN_POINT ( 'NONE',  ( -7.338753868364999988, 1517.184383877180153, 206.8309596656170015 ) ) ;
#38786=CARTESIAN_POINT ( 'NONE',  ( -5.943999059570199250, 1511.034527886640262, 201.5415479481260093 ) ) ;
#38794=CARTESIAN_POINT ( 'NONE',  ( -5.002593397454999646, 1516.960844870249957, 215.6810146069769871 ) ) ;
#38797=CARTESIAN_POINT ( 'NONE',  ( 2.414383718323408257, 1516.533281679525544, 216.8308509075874611 ) ) ;
#38798=CARTESIAN_POINT ( 'NONE',  ( 2.491188358395000080, 1516.733363207009916, 213.1488973760370129 ) ) ;
#38813=AXIS2_PLACEMENT_3D ( 'NONE', #106033, #93870, #71918 ) ;
#38816=CARTESIAN_POINT ( 'NONE',  ( 2.479246847704999812, 1516.983612918759945, 205.0778556245070092 ) ) ;
#38822=DIRECTION ( 'NONE',  ( -1.000000000000000000, 0.000000000000000000, 0.000000000000000000 ) ) ;
#38830=VECTOR ( 'NONE', #53016, 1000.000000000000000 ) ;
#38848=LINE ( 'NONE', #75238, #98208 ) ;
#38849=CARTESIAN_POINT ( 'NONE',  ( -7.530701528224715169, 1510.600498159482868, 214.9792805877740420 ) ) ;
#38852=CARTESIAN_POINT ( 'NONE',  ( -12.73246623696499924, 1512.053076656670100, 193.2925894132669953 ) ) ;
#38855=CARTESIAN_POINT ( 'NONE',  ( 1.708747624254999931, 1517.213554313520035, 202.1696795498070003 ) ) ;
#38871=CARTESIAN_POINT ( 'NONE',  ( -7.583791944165000132, 1511.751588929339960, 211.4475770739170173 ) ) ;
#38889=CARTESIAN_POINT ( 'NONE',  ( 6.556651371285000529, 1516.858146885269889, 215.6747433371770057 ) ) ;
#38891=ORIENTED_EDGE ( 'NONE', *, *, #104881, .F. ) ;
#38897=CARTESIAN_POINT ( 'NONE',  ( -1.714334285315000095, 1516.699825673279975, 205.0952314524469955 ) ) ;
#38910=CARTESIAN_POINT ( 'NONE',  ( -6.547881413045000265, 1516.647534046129977, 212.5778533554070293 ) ) ;
#38917=CARTESIAN_POINT ( 'NONE',  ( -7.709047995734989556, 1516.534924556719943, 211.5762535550240102 ) ) ;
#38918=CARTESIAN_POINT ( 'NONE',  ( 1.717139084115000047, 1516.949031626070109, 210.2396860569670025 ) ) ;
#38928=CARTESIAN_POINT ( 'NONE',  ( 7.572192850525000019, 1511.308638870219966, 206.5572121486769959 ) ) ;
#38931=CARTESIAN_POINT ( 'NONE',  ( 0.01126491619350150110, 1516.939530130779985, 216.0663127125970107 ) ) ;
#38936=CARTESIAN_POINT ( 'NONE',  ( -3.454748846324999789, 1516.609912606490070, 201.7988116581369979 ) ) ;
#38942=CARTESIAN_POINT ( 'NONE',  ( 7.550412389219739673, 1510.476657126699820, 203.5713960734849763 ) ) ;
#38955=FACE_OUTER_BOUND ( 'NONE', #54913, .T. ) ;
#38964=CARTESIAN_POINT ( 'NONE',  ( -7.500000019064999357, 1516.934643012909874, 209.1218459511669892 ) ) ;
#38975=CARTESIAN_POINT ( 'NONE',  ( 12.72383573552339975, 1512.260118274589786, 224.2302556167890089 ) ) ;
#39015=CARTESIAN_POINT ( 'NONE',  ( -3.251394400264999707, 1516.757508073510053, 210.8375504612070017 ) ) ;
#39018=CARTESIAN_POINT ( 'NONE',  ( 3.267603515704999850, 1516.858171774179937, 212.3749871074670068 ) ) ;
#39024=CARTESIAN_POINT ( 'NONE',  ( -5.004442077115000664, 1516.690345681169902, 201.4087281291169802 ) ) ;
#39026=DIRECTION ( 'NONE',  ( 0.000000000000000000, -0.8237382389120454507, 0.5669702935375731112 ) ) ;
#39033=ORIENTED_EDGE ( 'NONE', *, *, #68675, .F. ) ;
#39038=CARTESIAN_POINT ( 'NONE',  ( -4.610079871555000430, 1516.713079096360161, 210.2553629353369899 ) ) ;
#39043=CARTESIAN_POINT ( 'NONE',  ( 7.635834362694999378, 1511.005930286180046, 205.1946200654369932 ) ) ;
#39045=CARTESIAN_POINT ( 'NONE',  ( -6.564578723344999922, 1517.199196846569976, 207.4137433428170141 ) ) ;
#39064=CARTESIAN_POINT ( 'NONE',  ( 4.618749068485000109, 1516.729202374750002, 215.6716084172169872 ) ) ;
#39066=CARTESIAN_POINT ( 'NONE',  ( 7.709271376012959642, 1516.543456561459834, 206.4978234970299980 ) ) ;
#39093=CARTESIAN_POINT ( 'NONE',  ( -3.611462641674999752, 1511.572472350439739, 201.0497519038969756 ) ) ;
#39098=EDGE_CURVE ( 'NONE', #19743, #69935, #34531, .T. ) ;
#39134=CARTESIAN_POINT ( 'NONE',  ( -7.444284933535620041, 1510.876154134890157, 215.3695507499089956 ) ) ;
#39140=CARTESIAN_POINT ( 'NONE',  ( 5.772978278544999675, 1516.659138130710289, 207.9900491214870044 ) ) ;
#39169=ORIENTED_EDGE ( 'NONE', *, *, #63840, .F. ) ;
#39170=CARTESIAN_POINT ( 'NONE',  ( 3.801734722905379726, 1509.034524749680031, 204.6344874870430317 ) ) ;
#39172=CARTESIAN_POINT ( 'NONE',  ( -1.906500024517750053E-08, 1508.551704408389924, 202.1089243866269953 ) ) ;
#39179=EDGE_CURVE ( 'NONE', #36663, #42670, #53195, .T. ) ;
#39181=CARTESIAN_POINT ( 'NONE',  ( 2.480813884984999884, 1517.051603658920158, 204.1089070683270279 ) ) ;
#39188=CARTESIAN_POINT ( 'NONE',  ( 4.487249753806469954, 1509.038615938009798, 205.6342535008409982 ) ) ;
#39190=CARTESIAN_POINT ( 'NONE',  ( -12.18971938666500066, 1512.123542805230272, 194.3960765485670095 ) ) ;
#39193=CARTESIAN_POINT ( 'NONE',  ( 6.141424742704666428, 1511.655929346004314, 217.9160887146131245 ) ) ;
#39202=CARTESIAN_POINT ( 'NONE',  ( -7.649034438594999763, 1514.243099272629934, 203.4721261815869866 ) ) ;
#39203=VERTEX_POINT ( 'NONE', #92640 ) ;
#39219=CARTESIAN_POINT ( 'NONE',  ( 15.05391205133499888, 1514.225267046429963, 225.1144834937670112 ) ) ;
#39251=CARTESIAN_POINT ( 'NONE',  ( 6.105460688195506691, 1510.769285161600010, 216.6036268165167940 ) ) ;
#39274=DIRECTION ( 'NONE',  ( 0.01802056537744943510, 0.000000000000000000, -0.9998376164275263323 ) ) ;
#39283=CARTESIAN_POINT ( 'NONE',  ( -4.487172950141123273, 1511.405761256467713, 200.7686181660011471 ) ) ;
#39291=CARTESIAN_POINT ( 'NONE',  ( -7.335901033725000353, 1517.068717944079935, 205.0869373723870126 ) ) ;
#39306=CARTESIAN_POINT ( 'NONE',  ( -3.447128498755000159, 1516.778853242349896, 210.2570310142770040 ) ) ;
#39320=ORIENTED_EDGE ( 'NONE', *, *, #18926, .T. ) ;
#39322=CARTESIAN_POINT ( 'NONE',  ( -5.649719788644999241, 1514.243099272629934, 216.7708803706970002 ) ) ;
#39323=CARTESIAN_POINT ( 'NONE',  ( 16.68633773671889742, 1513.912053497473607, 195.2582997944726060 ) ) ;
#39329=CARTESIAN_POINT ( 'NONE',  ( 5.551188673975000043, 1510.480349266450048, 216.6723492941569873 ) ) ;
#39335=CARTESIAN_POINT ( 'NONE',  ( 4.487358949475809489, 1509.034510030706997, 205.3201214368218359 ) ) ;
#39336=CARTESIAN_POINT ( 'NONE',  ( 7.323390407215000231, 1516.613712827999962, 207.9924597298270044 ) ) ;
#39344=LINE ( 'NONE', #66778, #100775 ) ;
#39346=CARTESIAN_POINT ( 'NONE',  ( -5.395039083132619595, 1511.384172056590160, 200.9623232297749666 ) ) ;
#39349=CARTESIAN_POINT ( 'NONE',  ( -7.734617125744999377, 1513.613303996360173, 216.9435780305869912 ) ) ;
#39355=CARTESIAN_POINT ( 'NONE',  ( 0.01073129396420149928, 1516.939491476980038, 216.4539099096770087 ) ) ;
#39359=CARTESIAN_POINT ( 'NONE',  ( -2.479246885834999858, 1516.983612918759945, 213.1658362778269691 ) ) ;
#39378=CARTESIAN_POINT ( 'NONE',  ( 4.029572640705000985, 1516.858649670339901, 205.0803734583570019 ) ) ;
#39414=CARTESIAN_POINT ( 'NONE',  ( -7.548036999711751349, 1510.518062821254716, 214.7935333685385615 ) ) ;
#39417=CARTESIAN_POINT ( 'NONE',  ( -14.46755554256499998, 1513.509764667529907, 193.9550704101670249 ) ) ;
#39421=CARTESIAN_POINT ( 'NONE',  ( -4.617490504904999682, 1516.685667699390024, 201.7969310139470167 ) ) ;
#39424=CARTESIAN_POINT ( 'NONE',  ( 16.11904262073499794, 1512.169992403149990, 197.6534206206669921 ) ) ;
#39451=CARTESIAN_POINT ( 'NONE',  ( 7.316722005465000400, 1511.382498894329956, 202.5414830215270001 ) ) ;
#39461=CARTESIAN_POINT ( 'NONE',  ( -6.941100315875000426, 1516.858069504249897, 216.0654486236869900 ) ) ;
#39469=CARTESIAN_POINT ( 'NONE',  ( -1.135185082175000026, 1516.778853242349896, 205.6747174714770097 ) ) ;
#39471=CARTESIAN_POINT ( 'NONE',  ( 3.261652286895000419, 1516.939580991450157, 209.1085619926769823 ) ) ;
#39485=CARTESIAN_POINT ( 'NONE',  ( -4.609673279564999504, 1516.754149861460064, 212.3872530880769887 ) ) ;
#39490=CARTESIAN_POINT ( 'NONE',  ( -7.710086906866910006, 1516.574598972179956, 210.5804421991259971 ) ) ;
#39491=CARTESIAN_POINT ( 'NONE',  ( -1.119592219845000125, 1516.958737650239982, 210.2577447559170025 ) ) ;
#39504=DIRECTION ( 'NONE',  ( 0.000000000000000000, -1.000000000000000000, 6.123233995736769734E-17 ) ) ;
#39505=AXIS2_PLACEMENT_3D ( 'NONE', #105248, #86786, #61608 ) ;
#39506=CARTESIAN_POINT ( 'NONE',  ( -0.7391220051939990654, 1517.130100026000036, 216.0715493048870144 ) ) ;
#39511=CARTESIAN_POINT ( 'NONE',  ( 3.453544825624999870, 1517.106845464700200, 201.7850012896870169 ) ) ;
#39526=DIRECTION ( 'NONE',  ( 0.000000000000000000, 6.123233995736769734E-17, 1.000000000000000000 ) ) ;
#39538=DIRECTION ( 'NONE',  ( 0.9996573249755569268, -0.02617694830788839730, 1.602875797835060866E-18 ) ) ;
#39547=CARTESIAN_POINT ( 'NONE',  ( 12.49443849680770136, 1512.179780174510142, 224.0980365015450104 ) ) ;
#39552=CARTESIAN_POINT ( 'NONE',  ( 6.100701914535983761, 1516.739200664758528, 204.7580812289224355 ) ) ;
#39559=DIRECTION ( 'NONE',  ( -0.7063774289747313251, 0.04540766091858271930, -0.7063774289747313251 ) ) ;
#39588=CARTESIAN_POINT ( 'NONE',  ( 1.717432448265000078, 1516.836638729160086, 211.4041475482669910 ) ) ;
#39592=CARTESIAN_POINT ( 'NONE',  ( -1.702406023195000007, 1516.999105586269934, 212.3918307515370145 ) ) ;
#39598=CARTESIAN_POINT ( 'NONE',  ( -2.872700555325000238, 1516.559109716219837, 201.4121646638069763 ) ) ;
#39614=CARTESIAN_POINT ( 'NONE',  ( -3.447128498755000159, 1516.778853242349896, 210.2570310142770040 ) ) ;
#39620=CARTESIAN_POINT ( 'NONE',  ( 7.549016763624999626, 1510.423579818979988, 204.6938642082269837 ) ) ;
#39622=CARTESIAN_POINT ( 'NONE',  ( 1.700259675955000160, 1516.898441858519845, 207.4036424686470070 ) ) ;
#39637=DIRECTION ( 'NONE',  ( 0.000000000000000000, -6.123233995736769734E-17, -1.000000000000000000 ) ) ;
#39639=CARTESIAN_POINT ( 'NONE',  ( -3.259101837015000225, 1517.102359858469754, 216.0714209178769920 ) ) ;
#39647=CARTESIAN_POINT ( 'NONE',  ( 7.722580313994999557, 1517.051704397749972, 213.7119064319370239 ) ) ;
#39690=FACE_OUTER_BOUND ( 'NONE', #47725, .T. ) ;
#39695=EDGE_LOOP ( 'NONE', ( #108215, #93011, #32933, #20457 ) ) ;
#39711=CARTESIAN_POINT ( 'NONE',  ( -6.564578723344999922, 1517.199196846569976, 207.4137433428170141 ) ) ;
#39723=CARTESIAN_POINT ( 'NONE',  ( -5.513435590433334532, 1508.551704408459500, 216.2634855482666012 ) ) ;
#39733=ORIENTED_EDGE ( 'NONE', *, *, #72659, .T. ) ;
#39742=VERTEX_POINT ( 'NONE', #57300 ) ;
#39748=CARTESIAN_POINT ( 'NONE',  ( -6.559798094425000059, 1516.987478262539980, 204.5068286042669854 ) ) ;
#39758=DIRECTION ( 'NONE',  ( 0.7071067811865490160, 0.000000000000000000, 0.7071067811865461294 ) ) ;
#39760=CARTESIAN_POINT ( 'NONE',  ( -14.02477542606970040, 1513.114148093550057, 193.8538915311939661 ) ) ;
#39772=EDGE_LOOP ( 'NONE', ( #107485, #30911, #50088, #55230, #54741 ) ) ;
#39832=PRESENTATION_STYLE_ASSIGNMENT (( #57210 ) ) ;
#39839=CARTESIAN_POINT ( 'NONE',  ( -4.076752252616049788, 1511.455710048287301, 200.9017954071260021 ) ) ;
#39847=CARTESIAN_POINT ( 'NONE',  ( -4.623788007495000407, 1516.947419719950176, 205.6726967363569827 ) ) ;
#39861=CARTESIAN_POINT ( 'NONE',  ( -3.449647478144999724, 1516.829948096479939, 209.8791439064560223 ) ) ;
#39887=CARTESIAN_POINT ( 'NONE',  ( -5.005071046424999892, 1516.710692850270107, 201.7963041449669959 ) ) ;
#39888=CARTESIAN_POINT ( 'NONE',  ( 4.028611221114998919, 1516.744381837270112, 207.9874879615069858 ) ) ;
#39900=CARTESIAN_POINT ( 'NONE',  ( -5.671687354363034395, 1510.518062792044475, 201.5738089661925017 ) ) ;
#39906=CARTESIAN_POINT ( 'NONE',  ( -7.716878941104999612, 1516.833976295079992, 216.4517711926369827 ) ) ;
#39912=CARTESIAN_POINT ( 'NONE',  ( 7.724423394095000894, 1517.122088787240045, 212.5760185856570104 ) ) ;
#39916=CARTESIAN_POINT ( 'NONE',  ( 3.802992195031519973, 1508.880967439349888, 213.6144902172630111 ) ) ;
#39931=CARTESIAN_POINT ( 'NONE',  ( 0.7360974386200019870, 1517.045004075700035, 205.0794574309270217 ) ) ;
#39950=DIRECTION ( 'NONE',  ( 0.000000000000000000, -1.000000000000000000, 6.123233995736769734E-17 ) ) ;
#39966=CARTESIAN_POINT ( 'NONE',  ( -14.83035617076499868, 1514.570049710740022, 192.8394949842669917 ) ) ;
#39972=CARTESIAN_POINT ( 'NONE',  ( 2.290256263724999908, 1517.170721208160103, 202.1706708033170230 ) ) ;
#39975=CARTESIAN_POINT ( 'NONE',  ( 15.78436436263500120, 1512.151624459629829, 197.9925267198669872 ) ) ;
#39979=CARTESIAN_POINT ( 'NONE',  ( 3.958649409925110163, 1508.551704408389924, 204.1347675188470134 ) ) ;
#39987=CARTESIAN_POINT ( 'NONE',  ( -7.780733106055000903, 1512.320675624280057, 211.9528311838369916 ) ) ;
#39998=VERTEX_POINT ( 'NONE', #7815 ) ;
#40006=CARTESIAN_POINT ( 'NONE',  ( 2.292307230374999616, 1516.548716157039962, 216.0554627912370051 ) ) ;
#40013=CARTESIAN_POINT ( 'NONE',  ( -2.298048961635000165, 1516.764084769670262, 205.6764383981169715 ) ) ;
#40015=CARTESIAN_POINT ( 'NONE',  ( 7.332063939445000678, 1516.939491476980038, 209.1111146381379911 ) ) ;
#40019=CARTESIAN_POINT ( 'NONE',  ( 6.013893971085000345, 1511.644799026709961, 217.0731095806869746 ) ) ;
#40029=CARTESIAN_POINT ( 'NONE',  ( 1.713317409674999903, 1516.660388280709867, 213.7298676393670291 ) ) ;
#40035=CARTESIAN_POINT ( 'NONE',  ( 0.7559394982620020187, 1516.972341476009888, 210.2438793621770117 ) ) ;
#40040=VERTEX_POINT ( 'NONE', #3025 ) ;
#40049=AXIS2_PLACEMENT_3D ( 'NONE', #15048, #91227, #66057 ) ;
#40050=CARTESIAN_POINT ( 'NONE',  ( 4.036119644515000715, 1516.647924054489977, 216.4458205765370167 ) ) ;
#40055=CARTESIAN_POINT ( 'NONE',  ( 6.554151426245000245, 1516.906641539930206, 201.7900338461269882 ) ) ;
#40057=CARTESIAN_POINT ( 'NONE',  ( -15.07517731296499974, 1511.972232048389969, 221.4259079178670220 ) ) ;
#40075=CARTESIAN_POINT ( 'NONE',  ( 3.330134165755000097, 1515.051704408389924, 213.4516374609670208 ) ) ;
#40091=CARTESIAN_POINT ( 'NONE',  ( 12.89209530779459989, 1512.335564144490036, 224.3027625489149841 ) ) ;
#40123=VERTEX_POINT ( 'NONE', #80807 ) ;
#40130=CARTESIAN_POINT ( 'NONE',  ( 7.725372132234999967, 1517.158319634930194, 211.9946825927569876 ) ) ;
#40133=CARTESIAN_POINT ( 'NONE',  ( 2.878693249144999466, 1516.766397346390022, 213.1495431961470217 ) ) ;
#40141=CARTESIAN_POINT ( 'NONE',  ( 3.452917022905000355, 1517.089216728169959, 202.1725802860869976 ) ) ;
#40143=B_SPLINE_SURFACE_WITH_KNOTS ( 'NONE', 5, 5, ( 
 ( #29908, #98773, #62464, #54061, #20950, #39975, #24796, #14210, #5269 ),
 ( #101510, #65745, #66857, #48396, #99862, #39424, #74150, #84176, #24263 ),
 ( #15305, #57361, #90924, #57898, #82539, #91485, #59001, #99308, #100966 ),
 ( #5835, #58443, #92571, #14765, #66313, #49497, #15842, #108281, #41636 ),
 ( #83622, #56787, #32678, #93129, #31568, #50047, #7474, #75791, #6919 ),
 ( #47830, #92033, #23159, #48952, #81963, #41075, #83083, #23713, #67410 ),
 ( #6376, #73601, #107731, #109943, #31016, #65196, #22582, #40522, #75253 ),
 ( #74700, #33221, #108831, #32128, #100430, #109402, #27048, #1296, #84722 ),
 ( #51144, #52809, #60107, #750, #9137, #70190, #76338, #26471, #33768 ) ),
 .UNSPECIFIED., .F., .F., .F.,
 ( 6, 3, 6 ),
 ( 6, 3, 6 ),
 ( 9.902195898180000455, 12.38020728900000123, 16.40090783169999966 ),
 ( 0.000000000000000000, 0.5000000000000000000, 1.000000000000000000 ),
 .UNSPECIFIED. ) ;
#40152=CARTESIAN_POINT ( 'NONE',  ( -1.906499846882070084E-08, 1508.551704408389924, 209.1218459511669892 ) ) ;
#40158=CARTESIAN_POINT ( 'NONE',  ( 6.950833530105000158, 1517.156142772249950, 211.6057959108269984 ) ) ;
#40164=CARTESIAN_POINT ( 'NONE',  ( 7.622960486734998931, 1511.191277613550028, 205.7361320510769929 ) ) ;
#40165=CARTESIAN_POINT ( 'NONE',  ( -0.7579844201469989606, 1516.883361325900069, 206.8353730456769881 ) ) ;
#40172=CARTESIAN_POINT ( 'NONE',  ( -5.614653854145000622, 1512.956339156650074, 203.5071921160869977 ) ) ;
#40183=CARTESIAN_POINT ( 'NONE',  ( -1.709384611084999950, 1517.224900789629828, 216.4615953054470197 ) ) ;
#40185=CARTESIAN_POINT ( 'NONE',  ( 7.708854789774719940, 1516.527547774869845, 206.9824925634590045 ) ) ;
#40255=CARTESIAN_POINT ( 'NONE',  ( 4.995623452895000760, 1516.636036526019780, 207.4092012159470073 ) ) ;
#40280=CARTESIAN_POINT ( 'NONE',  ( 4.159863633235049818, 1508.728286123109910, 204.6953547332600181 ) ) ;
#40281=CARTESIAN_POINT ( 'NONE',  ( -8.753854093810092607, 1516.720891557477444, 204.9704016331489811 ) ) ;
#40285=EDGE_CURVE ( 'NONE', #42643, #76367, #94399, .T. ) ;
#40288=CARTESIAN_POINT ( 'NONE',  ( -4.364191184633019915, 1509.032029208890208, 205.0059634122790158 ) ) ;
#40290=CARTESIAN_POINT ( 'NONE',  ( -4.040527342105000308, 1516.815231249920089, 204.5109077207270047 ) ) ;
#40293=CARTESIAN_POINT ( 'NONE',  ( 15.08187215528230141, 1512.240709848920005, 196.4484943621689865 ) ) ;
#40300=CARTESIAN_POINT ( 'NONE',  ( -13.31081197707080044, 1512.571279492550048, 193.8315606877860091 ) ) ;
#40316=VECTOR ( 'NONE', #62000, 1000.000000000000000 ) ;
#40327=AXIS2_PLACEMENT_3D ( 'NONE', #43342, #77490, #36042 ) ;
#40363=EDGE_LOOP ( 'NONE', ( #23491, #45192, #67559, #18498 ) ) ;
#40381=CARTESIAN_POINT ( 'NONE',  ( -3.000855178852367633, 1512.041030487102034, 201.2259107305448822 ) ) ;
#40386=CARTESIAN_POINT ( 'NONE',  ( 7.322709686834999232, 1516.596789218710001, 205.8608388005369818 ) ) ;
#40392=ORIENTED_EDGE ( 'NONE', *, *, #106560, .T. ) ;
#40400=CARTESIAN_POINT ( 'NONE',  ( 3.463767257884999839, 1517.014196759610059, 210.8246003415769962 ) ) ;
#40422=CARTESIAN_POINT ( 'NONE',  ( -3.487592467065220081, 1508.551704408389924, 204.1347675093749956 ) ) ;
#40424=CARTESIAN_POINT ( 'NONE',  ( 6.186741257861129384, 1516.987734611904671, 213.4228617371842063 ) ) ;
#40429=CARTESIAN_POINT ( 'NONE',  ( 7.329303077985000137, 1516.857992118400034, 201.7912917986770083 ) ) ;
#40430=CARTESIAN_POINT ( 'NONE',  ( -0.7559395363919990674, 1516.972341476009888, 207.9998125401569951 ) ) ;
#40441=CARTESIAN_POINT ( 'NONE',  ( -5.384056492903469326, 1511.434805660039956, 200.4695677088149921 ) ) ;
#40448=CARTESIAN_POINT ( 'NONE',  ( -5.003848160104999998, 1517.005755693489846, 216.4561742428970206 ) ) ;
#40453=CARTESIAN_POINT ( 'NONE',  ( -1.120543735785000106, 1517.073005577650065, 213.1661658574570026 ) ) ;
#40474=CARTESIAN_POINT ( 'NONE',  ( -2.492130661305000050, 1516.778761582560037, 205.6761608547170113 ) ) ;
#40503=CARTESIAN_POINT ( 'NONE',  ( 7.445037983834265738, 1508.731359867039373, 203.6084103738589022 ) ) ;
#40516=CARTESIAN_POINT ( 'NONE',  ( -7.065869411249059873, 1517.051704406860154, 205.0465358202790185 ) ) ;
#40519=CARTESIAN_POINT ( 'NONE',  ( -2.292307268505000106, 1516.548716157039962, 202.1882291110970300 ) ) ;
#40520=CARTESIAN_POINT ( 'NONE',  ( -8.788663597526685578, 1511.593711396709296, 215.1384066147768976 ) ) ;
#40522=CARTESIAN_POINT ( 'NONE',  ( 16.51584604633499964, 1514.088841912139969, 194.6296875079669917 ) ) ;
#40537=CARTESIAN_POINT ( 'NONE',  ( -7.683494276754999852, 1512.058324472099912, 211.8336161652269993 ) ) ;
#40557=CARTESIAN_POINT ( 'NONE',  ( -3.258474617075000079, 1517.083030555940013, 215.6838419306269827 ) ) ;
#40559=EDGE_CURVE ( 'NONE', #9383, #39203, #81760, .T. ) ;
#40566=CARTESIAN_POINT ( 'NONE',  ( -5.786527600464999033, 1517.025653221279981, 205.6708125431369751 ) ) ;
#40568=CARTESIAN_POINT ( 'NONE',  ( -2.486220139904999904, 1516.939658295650133, 209.1350829839039989 ) ) ;
#40571=CARTESIAN_POINT ( 'NONE',  ( 6.597706014745000402, 1512.335510084630187, 217.2026964005870013 ) ) ;
#40574=CARTESIAN_POINT ( 'NONE',  ( 5.513435558228538369, 1508.611350403035431, 216.4436907933061320 ) ) ;
#40578=VECTOR ( 'NONE', #57282, 1000.000000000000000 ) ;
#40580=CARTESIAN_POINT ( 'NONE',  ( 5.008848199894999631, 1516.858456333729919, 214.1219297979669989 ) ) ;
#40585=CARTESIAN_POINT ( 'NONE',  ( -7.713601987141389671, 1516.708834472129865, 209.9201896328700059 ) ) ;
#40586=CARTESIAN_POINT ( 'NONE',  ( 1.135898785685000023, 1516.958737650239982, 210.2414381519470226 ) ) ;
#40602=CARTESIAN_POINT ( 'NONE',  ( -5.003220765204999587, 1516.983995446890049, 216.0685944891870065 ) ) ;
#40607=CARTESIAN_POINT ( 'NONE',  ( 5.777745395274999751, 1516.908489800550115, 202.5639360494670029 ) ) ;
#40608=CARTESIAN_POINT ( 'NONE',  ( -15.73511544386499850, 1514.703592237370003, 224.4575895832670085 ) ) ;
#40663=CARTESIAN_POINT ( 'NONE',  ( -4.987078454554999318, 1508.551704408389924, 205.6342535004969818 ) ) ;
#40674=CARTESIAN_POINT ( 'NONE',  ( -8.126234285584999384, 1514.923664147150021, 202.9950997886369635 ) ) ;
#40684=CARTESIAN_POINT ( 'NONE',  ( -7.709032175815000443, 1516.534320418310244, 211.6070631641669877 ) ) ;
#40688=CARTESIAN_POINT ( 'NONE',  ( -4.028630622785000170, 1516.812923327049930, 212.5819478221170016 ) ) ;
#40695=CARTESIAN_POINT ( 'NONE',  ( -6.943602691585000208, 1516.858069504249897, 202.1807456543569685 ) ) ;
#40696=CARTESIAN_POINT ( 'NONE',  ( -8.648691763575000024, 1514.216922324319739, 203.4721261815869866 ) ) ;
#40711=CARTESIAN_POINT ( 'NONE',  ( 7.726331925474999807, 1517.194972660189933, 211.4133602680070112 ) ) ;
#40716=CARTESIAN_POINT ( 'NONE',  ( -4.625693903144999730, 1517.042661899400173, 206.8353996064669786 ) ) ;
#40723=B_SPLINE_CURVE_WITH_KNOTS ( 'NONE', 5,
 ( #52166, #18517, #103654, #28042, #54382, #43753 ),
 .UNSPECIFIED., .F., .F.,
 ( 6, 6 ),
 ( 0.000000000000000000, 1.000000000000000000 ),
 .UNSPECIFIED. ) ;
#40734=CARTESIAN_POINT ( 'NONE',  ( 15.55634916703500004, 1516.551704408390151, 193.5654967650670244 ) ) ;
#40735=CARTESIAN_POINT ( 'NONE',  ( 4.618119666265000589, 1516.706638732659940, 216.0591847158069925 ) ) ;
#40760=CARTESIAN_POINT ( 'NONE',  ( -1.906499846882070084E-08, 1517.051704408389924, 209.1218459511669892 ) ) ;
#40769=CARTESIAN_POINT ( 'NONE',  ( -14.44303134326499993, 1516.995662938509895, 225.7915129991669971 ) ) ;
#40790=CARTESIAN_POINT ( 'NONE',  ( -6.252266492314999979, 1511.741868877540128, 200.3335294429169835 ) ) ;
#40792=EDGE_CURVE ( 'NONE', #98390, #36271, #96834, .T. ) ;
#40798=LINE ( 'NONE', #74977, #3629 ) ;
#40802=CARTESIAN_POINT ( 'NONE',  ( -7.518184220077429814, 1510.874996213040049, 215.1349743772009901 ) ) ;
#40807=CARTESIAN_POINT ( 'NONE',  ( 6.556850996575000146, 1516.939568781210028, 209.1101343261499892 ) ) ;
#40816=CARTESIAN_POINT ( 'NONE',  ( -14.86137038355130002, 1512.142158944850053, 221.4605574290570189 ) ) ;
#40844=CARTESIAN_POINT ( 'NONE',  ( -4.802232148216890373, 1508.551704408389924, 204.6920728333849979 ) ) ;
#40846=CARTESIAN_POINT ( 'NONE',  ( -3.265407155974999753, 1516.754149861460064, 204.5121726906670006 ) ) ;
#40849=CARTESIAN_POINT ( 'NONE',  ( 15.10400614679230102, 1513.569700116999911, 194.6305253545030212 ) ) ;
#40853=CARTESIAN_POINT ( 'NONE',  ( -13.23930721601690053, 1512.526687531830021, 193.8438098916049910 ) ) ;
#40920=EDGE_CURVE ( 'NONE', #71147, #12190, #28364, .T. ) ;
#40934=CARTESIAN_POINT ( 'NONE',  ( -4.993716309010864940, 1511.400001115550822, 200.6009875924737855 ) ) ;
#40939=CARTESIAN_POINT ( 'NONE',  ( 4.997250153905000047, 1516.727068157269969, 205.8570671527170077 ) ) ;
#40949=CARTESIAN_POINT ( 'NONE',  ( -16.78936288871751614, 1513.473960729824284, 222.1909530149808631 ) ) ;
#40953=CARTESIAN_POINT ( 'NONE',  ( 2.881548424445000034, 1516.909589401870107, 211.4054166033970148 ) ) ;
#40960=EDGE_LOOP ( 'NONE', ( #76010, #17823, #39169 ) ) ;
#40979=CARTESIAN_POINT ( 'NONE',  ( -0.7538707734179979081, 1516.719999691880048, 202.1833671473370089 ) ) ;
#40980=CARTESIAN_POINT ( 'NONE',  ( -7.726684725664999753, 1517.208444099459939, 207.9957078235169945 ) ) ;
#40998=CARTESIAN_POINT ( 'NONE',  ( 7.717505752974999744, 1516.857914730730045, 216.8393517232070167 ) ) ;
#41004=CARTESIAN_POINT ( 'NONE',  ( -0.4346943098025670138, 1517.051704408590012, 216.8444262844809884 ) ) ;
#41005=CARTESIAN_POINT ( 'NONE',  ( -6.548821979184999975, 1516.688761843659904, 213.1592242262869945 ) ) ;
#41008=CARTESIAN_POINT ( 'NONE',  ( 4.492644271869690620, 1508.880967335730247, 212.9248485414070160 ) ) ;
#41023=CARTESIAN_POINT ( 'NONE',  ( 0.7355686427760019797, 1517.012231669750008, 205.8548062402470009 ) ) ;
#41031=DIRECTION ( 'NONE',  ( 1.000000000000000000, 0.000000000000000000, 0.000000000000000000 ) ) ;
#41045=CARTESIAN_POINT ( 'NONE',  ( -14.09480582055672926, 1514.058997558268629, 192.5091585815071937 ) ) ;
#41063=CARTESIAN_POINT ( 'NONE',  ( -7.540337791715355564, 1510.559702728800175, 214.8951611895496399 ) ) ;
#41066=CARTESIAN_POINT ( 'NONE',  ( -15.05391208946500115, 1514.225267046429963, 193.1292084085670240 ) ) ;
#41072=CARTESIAN_POINT ( 'NONE',  ( 5.003220727074999985, 1516.983995446890049, 202.1750974131470286 ) ) ;
#41075=CARTESIAN_POINT ( 'NONE',  ( 16.52887561823499851, 1513.466724478469814, 194.9208948791670082 ) ) ;
#41103=ORIENTED_EDGE ( 'NONE', *, *, #65451, .T. ) ;
#41109=CARTESIAN_POINT ( 'NONE',  ( -1.124289693584999972, 1517.184063036290127, 215.6857614941170027 ) ) ;
#41110=CARTESIAN_POINT ( 'NONE',  ( -7.951444182101831792, 1511.804172066088313, 212.3302999886905980 ) ) ;
#41115=CARTESIAN_POINT ( 'NONE',  ( -6.561686461364999445, 1517.069378699710114, 205.6695567495270041 ) ) ;
#41117=CARTESIAN_POINT ( 'NONE',  ( -5.011551406145000165, 1517.080322339569875, 208.3849417611969841 ) ) ;
#41123=ORIENTED_EDGE ( 'NONE', *, *, #86544, .F. ) ;
#41129=CARTESIAN_POINT ( 'NONE',  ( -7.711550716115000093, 1516.630499592039996, 213.1573366827869904 ) ) ;
#41133=CARTESIAN_POINT ( 'NONE',  ( 7.012524221607120190, 1508.551704613440052, 215.1061910685279770 ) ) ;
#41135=CARTESIAN_POINT ( 'NONE',  ( 5.788691325514999875, 1517.157901477309906, 210.2449475486469908 ) ) ;
#41156=CARTESIAN_POINT ( 'NONE',  ( -3.260357166894999992, 1517.133889586189980, 216.8465783791270098 ) ) ;
#41161=CARTESIAN_POINT ( 'NONE',  ( 1.708102589285000139, 1517.199196846569976, 202.5572672468869939 ) ) ;
#41162=CARTESIAN_POINT ( 'NONE',  ( -16.48353621536499958, 1512.679339245399888, 220.7760042011669839 ) ) ;
#41174=LINE ( 'NONE', #32765, #57449 ) ;
#41184=CARTESIAN_POINT ( 'NONE',  ( -3.487585252374380218, 1508.551704408389924, 213.9544597463709863 ) ) ;
#41239=CARTESIAN_POINT ( 'NONE',  ( -2.477373643995000485, 1516.891731298979948, 212.0030687278169808 ) ) ;
#41243=CARTESIAN_POINT ( 'NONE',  ( -4.997250192034999650, 1516.727068157269969, 212.3866247496169990 ) ) ;
#41251=CARTESIAN_POINT ( 'NONE',  ( -0.7538707734179979081, 1516.719999691880048, 202.1833671473370089 ) ) ;
#41266=CARTESIAN_POINT ( 'NONE',  ( -2.476170635034999901, 1516.819260244609950, 210.8389306816469855 ) ) ;
#41272=CARTESIAN_POINT ( 'NONE',  ( -0.01319654689839849966, 1516.941178807709775, 206.8296289214069930 ) ) ;
#41283=DIRECTION ( 'NONE',  ( 0.000000000000000000, 6.123233995736769734E-17, 1.000000000000000000 ) ) ;
#41289=CARTESIAN_POINT ( 'NONE',  ( 6.946748518954999341, 1516.983995446890049, 214.1250666973070054 ) ) ;
#41292=CARTESIAN_POINT ( 'NONE',  ( -2.290256301855000398, 1517.170721208160103, 216.0730210990169837 ) ) ;
#41335=ORIENTED_EDGE ( 'NONE', *, *, #83922, .F. ) ;
#41340=LINE ( 'NONE', #67109, #71096 ) ;
#41357=CARTESIAN_POINT ( 'NONE',  ( -15.90990259576500065, 1512.830284628050094, 220.0820010595669771 ) ) ;
#41373=CARTESIAN_POINT ( 'NONE',  ( 3.255809864005000165, 1516.837969789639828, 208.3644199470059846 ) ) ;
#41408=CARTESIAN_POINT ( 'NONE',  ( 3.253462060665000433, 1516.874084700499907, 205.6604858388269861 ) ) ;
#41430=CARTESIAN_POINT ( 'NONE',  ( -7.641777896465000275, 1513.965983108850196, 203.2025656438369765 ) ) ;
#41498=CARTESIAN_POINT ( 'NONE',  ( -7.012921583605000286, 1508.551704408389924, 214.6352815282469919 ) ) ;
#41504=CARTESIAN_POINT ( 'NONE',  ( -1.716392779905000054, 1516.788317650260069, 206.2580580763669786 ) ) ;
#41512=CARTESIAN_POINT ( 'NONE',  ( -16.37694617458279822, 1512.916366990779579, 220.6826468655462463 ) ) ;
#41516=CARTESIAN_POINT ( 'NONE',  ( 4.043990307595000111, 1516.983612918759945, 211.6010928179370012 ) ) ;
#41536=AXIS2_PLACEMENT_3D ( 'NONE', #64175, #39504, #73678 ) ;
#41546=CARTESIAN_POINT ( 'NONE',  ( -2.485846037024999955, 1516.545806094630279, 201.8003900583769905 ) ) ;
#41547=CARTESIAN_POINT ( 'NONE',  ( -5.013429394184999666, 1517.123342927159911, 207.9998951881570122 ) ) ;
#41550=CARTESIAN_POINT ( 'NONE',  ( 3.858606800919823332, 1511.506734315490121, 217.2722139618800838 ) ) ;
#41567=CARTESIAN_POINT ( 'NONE',  ( -2.290886304614999869, 1517.184383877180153, 216.4605998004670084 ) ) ;
#41571=CARTESIAN_POINT ( 'NONE',  ( 1.353280373286737559, 1516.590829936330465, 216.8323578617266207 ) ) ;
#41572=CARTESIAN_POINT ( 'NONE',  ( 7.334957356574999920, 1517.030858226499959, 213.7381182667970165 ) ) ;
#41581=CARTESIAN_POINT ( 'NONE',  ( -3.915802145044672944, 1515.051704408389696, 204.7920544193108014 ) ) ;
#41590=CARTESIAN_POINT ( 'NONE',  ( -0.01327408612949850138, 1516.939877939420057, 205.6663500982469941 ) ) ;
#41633=CARTESIAN_POINT ( 'NONE',  ( 2.482067860225000366, 1517.099836525840146, 203.3337487049469985 ) ) ;
#41636=CARTESIAN_POINT ( 'NONE',  ( 16.61115974343499957, 1513.007288725360013, 197.1622553098669925 ) ) ;
#41660=CARTESIAN_POINT ( 'NONE',  ( 7.951263610455001185, 1511.644799026709961, 203.1079519610169939 ) ) ;
#41668=CARTESIAN_POINT ( 'NONE',  ( 3.454748808194999743, 1516.609912606490070, 216.4448802441970088 ) ) ;
#41675=CARTESIAN_POINT ( 'NONE',  ( 6.547881374914999775, 1516.647534046129977, 205.6658385469270058 ) ) ;
#41676=EDGE_LOOP ( 'NONE', ( #33366, #82674, #59448, #93292 ) ) ;
#41680=CARTESIAN_POINT ( 'NONE',  ( 7.194888332885001070, 1513.142795523620180, 216.4219129324669950 ) ) ;
#41688=CARTESIAN_POINT ( 'NONE',  ( 7.722536764694999611, 1517.050041317280147, 213.7387458049869906 ) ) ;
#41690=CARTESIAN_POINT ( 'NONE',  ( 6.253177251166829542, 1511.742575854359984, 217.9101135377649996 ) ) ;
#41691=CARTESIAN_POINT ( 'NONE',  ( 6.766101877248090091, 1508.878901734200099, 216.3823889200130282 ) ) ;
#41692=CARTESIAN_POINT ( 'NONE',  ( -2.476450702264999748, 1516.843453247299749, 211.4215022863270121 ) ) ;
#41704=CARTESIAN_POINT ( 'NONE',  ( 12.38551412853500011, 1511.900571936589813, 224.8158055378670213 ) ) ;
#41705=CARTESIAN_POINT ( 'NONE',  ( -0.7403206051589980019, 1517.139320148880188, 216.8467205834170102 ) ) ;
#41711=CARTESIAN_POINT ( 'NONE',  ( -4.036748876935000396, 1516.667393516340098, 202.1854475764570225 ) ) ;
#41728=DIRECTION ( 'NONE',  ( 0.8236474686107853049, 0.5669078173018522460, 0.01484500364079610613 ) ) ;
#41787=CARTESIAN_POINT ( 'NONE',  ( 5.011367946795000528, 1516.974592746400049, 212.5716232859570027 ) ) ;
#41793=CARTESIAN_POINT ( 'NONE',  ( -6.944231786295000042, 1516.882690742909972, 202.5683215544970039 ) ) ;
#41794=CARTESIAN_POINT ( 'NONE',  ( -7.565982892814109739, 1517.051704408389924, 208.6835997737739774 ) ) ;
#41803=ADVANCED_FACE ( 'NONE', ( #52238 ), #86366, .T. ) ;
#41810=CARTESIAN_POINT ( 'NONE',  ( 6.563595869685000750, 1517.154223579619838, 211.4114704024570131 ) ) ;
#41812=VECTOR ( 'NONE', #84288, 1000.000000000000227 ) ;
#41816=CARTESIAN_POINT ( 'NONE',  ( 2.868112131164999745, 1516.855632454399938, 208.3641823986619954 ) ) ;
#41824=B_SPLINE_SURFACE_WITH_KNOTS ( 'NONE', 5, 5, ( 
 ( #69549, #103669, #61157, #46540, #81206, #12903, #88531, #53289, #11815 ),
 ( #96932, #87993, #87427, #54936, #89065, #11280, #45985, #36458, #63892 ),
 ( #72290, #3436, #3987, #38112, #21278, #20741, #29165, #72832, #20200 ),
 ( #38657, #95817, #62819, #106423, #54398, #47082, #79586, #12350, #104773 ),
 ( #2891, #80675, #29707, #98007, #44895, #80117, #62248, #70657, #105884 ),
 ( #63354, #106966, #55486, #89612, #37567, #4523, #10723, #30250, #71768 ),
 ( #19085, #97471, #79044, #2346, #28058, #96373, #19652, #53856, #45444 ),
 ( #37009, #71202, #105323, #28616, #5057, #74494, #108622, #31910, #41430 ),
 ( #32477, #65541, #66649, #56027, #83966, #99649, #22940, #31357, #39202 ) ),
 .UNSPECIFIED., .F., .F., .F.,
 ( 6, 3, 6 ),
 ( 6, 3, 6 ),
 ( 3.580107477790000381, 6.558749095509999627, 9.700153431640000434 ),
 ( 0.000000000000000000, 0.5000000000000000000, 1.000000000000000000 ),
 .UNSPECIFIED. ) ;
#41832=CARTESIAN_POINT ( 'NONE',  ( 4.039897278065000208, 1516.787536375099990, 214.1203611275269907 ) ) ;
#41835=CARTESIAN_POINT ( 'NONE',  ( -1.124894088365000044, 1517.194816588360027, 216.0733631026070043 ) ) ;
#41908=B_SPLINE_CURVE_WITH_KNOTS ( 'NONE', 5,
 ( #21028, #4265, #81492, #11558, #22120, #47365, #29993, #45735, #38398 ),
 .UNSPECIFIED., .F., .F.,
 ( 6, 3, 6 ),
 ( 0.000000000000000000, 0.5000000000000000000, 1.000000000000000000 ),
 .UNSPECIFIED. ) ;
#41915=CARTESIAN_POINT ( 'NONE',  ( -8.322537005615968653, 1511.435455886209866, 214.5074547685709945 ) ) ;
#41921=CARTESIAN_POINT ( 'NONE',  ( 3.449647440015000122, 1516.829948096479939, 208.3645479958780129 ) ) ;
#41930=CARTESIAN_POINT ( 'NONE',  ( -3.415238448984999842, 1511.801704408389924, 213.5367417060670050 ) ) ;
#41937=ORIENTED_EDGE ( 'NONE', *, *, #102190, .F. ) ;
#41942=ORIENTED_EDGE ( 'NONE', *, *, #47515, .F. ) ;
#41945=ORIENTED_EDGE ( 'NONE', *, *, #71588, .T. ) ;
#41955=CARTESIAN_POINT ( 'NONE',  ( 3.254401403604999743, 1516.919782530640077, 205.0791161293069820 ) ) ;
#42006=CARTESIAN_POINT ( 'NONE',  ( 7.723480079395000253, 1517.086065052259983, 213.1573821953169841 ) ) ;
#42050=CARTESIAN_POINT ( 'NONE',  ( 1.702405985064999960, 1516.999105586269934, 205.8518611507970206 ) ) ;
#42060=CARTESIAN_POINT ( 'NONE',  ( -16.48452152037296159, 1514.266850646888997, 223.5216240896907038 ) ) ;
#42065=CARTESIAN_POINT ( 'NONE',  ( 5.788436334164999586, 1517.116049120239950, 211.4102033778369787 ) ) ;
#42089=CARTESIAN_POINT ( 'NONE',  ( 2.935376380067538982, 1516.592453103030493, 216.0331898163414621 ) ) ;
#42095=CARTESIAN_POINT ( 'NONE',  ( 2.484577657225000014, 1517.170512887980067, 201.7834339727070017 ) ) ;
#42096=CARTESIAN_POINT ( 'NONE',  ( 7.332063939445000678, 1516.939491476980038, 209.1111146381379911 ) ) ;
#42118=CARTESIAN_POINT ( 'NONE',  ( -3.801724533410361317, 1509.034510030706087, 204.6344869826262709 ) ) ;
#42120=CARTESIAN_POINT ( 'NONE',  ( -3.449777353855000062, 1516.974592746400049, 214.1332139170270068 ) ) ;
#42136=ORIENTED_EDGE ( 'NONE', *, *, #37776, .F. ) ;
#42137=CARTESIAN_POINT ( 'NONE',  ( 1.702754371344999962, 1517.014196759610059, 205.6580786742169948 ) ) ;
#42158=CARTESIAN_POINT ( 'NONE',  ( -13.86349730046637774, 1513.912023431221542, 192.4354951056943435 ) ) ;
#42175=CARTESIAN_POINT ( 'NONE',  ( -6.648384463103849562, 1508.610125760109895, 216.2179245631680260 ) ) ;
#42185=CARTESIAN_POINT ( 'NONE',  ( -6.944231786295000042, 1516.882690742909972, 202.5683215544970039 ) ) ;
#42189=DIRECTION ( 'NONE',  ( -0.7071067811865492381, 0.000000000000000000, 0.7071067811865457964 ) ) ;
#42190=CARTESIAN_POINT ( 'NONE',  ( -6.500000019064997581, 1515.051704408389924, 209.1218459511669892 ) ) ;
#42200=CARTESIAN_POINT ( 'NONE',  ( -3.487592468028334114, 1508.783371651612924, 213.6678281800169259 ) ) ;
#42208=DIRECTION ( 'NONE',  ( 6.706399138190049698E-17, -1.000000000000000000, 0.000000000000000000 ) ) ;
#42212=CARTESIAN_POINT ( 'NONE',  ( 5.763076004854999823, 1514.407352313670117, 201.4560207676169910 ) ) ;
#42220=CARTESIAN_POINT ( 'NONE',  ( -0.7396922758749979732, 1517.135701590510052, 216.4591432822169850 ) ) ;
#42230=CARTESIAN_POINT ( 'NONE',  ( -7.337153806245000354, 1517.119374999550018, 205.8621166342670108 ) ) ;
#42235=CARTESIAN_POINT ( 'NONE',  ( 6.809551132454999767, 1512.240414293160029, 216.3848881498070114 ) ) ;
#42243=CARTESIAN_POINT ( 'NONE',  ( 4.040527303974999818, 1516.815231249920089, 213.7327841816070020 ) ) ;
#42247=CARTESIAN_POINT ( 'NONE',  ( 6.140129320397309520, 1508.880864719049896, 216.6292689899020161 ) ) ;
#42248=CARTESIAN_POINT ( 'NONE',  ( -6.546302780145000000, 1516.577434278289957, 211.6089493897669911 ) ) ;
#42264=ORIENTED_EDGE ( 'NONE', *, *, #94494, .T. ) ;
#42265=CARTESIAN_POINT ( 'NONE',  ( -2.486474780875000512, 1516.560253536979872, 202.1879665292270261 ) ) ;
#42284=CARTESIAN_POINT ( 'NONE',  ( -4.832613825698169663, 1508.551704408610021, 212.6094309338790254 ) ) ;
#42290=LINE ( 'NONE', #93767, #41812 ) ;
#42308=FACE_OUTER_BOUND ( 'NONE', #30494, .T. ) ;
#42321=CARTESIAN_POINT ( 'NONE',  ( 7.530701491966509842, 1510.600498152046157, 203.2644113281531304 ) ) ;
#42328=DIRECTION ( 'NONE',  ( 1.000000000000000000, 0.000000000000000000, 0.000000000000000000 ) ) ;
#42341=CARTESIAN_POINT ( 'NONE',  ( 3.265407117845000151, 1516.754149861460064, 213.7315192116670062 ) ) ;
#42342=CARTESIAN_POINT ( 'NONE',  ( 5.106974046795000000, 1511.397837225850026, 217.6801467072069727 ) ) ;
#42346=CARTESIAN_POINT ( 'NONE',  ( -6.945490086935000029, 1516.932669162149978, 203.3434733684869968 ) ) ;
#42354=CARTESIAN_POINT ( 'NONE',  ( 6.126746143464999683, 1514.923664147150021, 200.9956116846470309 ) ) ;
#42359=CARTESIAN_POINT ( 'NONE',  ( 3.462948796544999652, 1516.956048353049937, 211.4063724288770061 ) ) ;
#42364=CARTESIAN_POINT ( 'NONE',  ( -5.011551406145000165, 1517.080322339569875, 208.3849417611969841 ) ) ;
#42366=DIRECTION ( 'NONE',  ( 0.001614263105669359660, 0.06164622090537569266, -0.9980967576356069015 ) ) ;
#42370=FACE_OUTER_BOUND ( 'NONE', #48289, .T. ) ;
#42379=CARTESIAN_POINT ( 'NONE',  ( -3.255340964424999761, 1516.962555622980062, 213.7459452615670159 ) ) ;
#42382=CARTESIAN_POINT ( 'NONE',  ( -4.035536263215000474, 1517.086065052259983, 216.8453260496270047 ) ) ;
#42404=ORIENTED_EDGE ( 'NONE', *, *, #77466, .T. ) ;
#42405=VERTEX_POINT ( 'NONE', #31694 ) ;
#42462=CARTESIAN_POINT ( 'NONE',  ( 2.292217010694999946, 1516.941178807709775, 209.1086494233340147 ) ) ;
#42470=LINE ( 'NONE', #41930, #4946 ) ;
#42478=ORIENTED_EDGE ( 'NONE', *, *, #7513, .T. ) ;
#42496=CARTESIAN_POINT ( 'NONE',  ( -3.267603553834999897, 1516.858171774179937, 205.8687047948669999 ) ) ;
#42497=VERTEX_POINT ( 'NONE', #83757 ) ;
#42499=CARTESIAN_POINT ( 'NONE',  ( 15.25249359122459936, 1513.170547668170002, 195.0348937637239999 ) ) ;
#42532=EDGE_CURVE ( 'NONE', #51877, #98379, #92132, .T. ) ;
#42551=CARTESIAN_POINT ( 'NONE',  ( 0.01322035751810150123, 1516.939819969850078, 213.1588969678170145 ) ) ;
#42578=VERTEX_POINT ( 'NONE', #40075 ) ;
#42594=VECTOR ( 'NONE', #74926, 1000.000000000000114 ) ;
#42596=CARTESIAN_POINT ( 'NONE',  ( -7.725372170364999569, 1517.158319634930194, 206.2490093095770192 ) ) ;
#42608=DIRECTION ( 'NONE',  ( 0.000000000000000000, -0.02617694830808806397, -0.9996573249755517088 ) ) ;
#42612=CARTESIAN_POINT ( 'NONE',  ( 2.494020282435000180, 1516.876240617270014, 211.4047611534970201 ) ) ;
#42641=CARTESIAN_POINT ( 'NONE',  ( 7.714371502985000184, 1516.738222552470233, 203.3422428319769892 ) ) ;
#42642=CARTESIAN_POINT ( 'NONE',  ( -1.122033430074999893, 1516.972341476009888, 209.8777854684929878 ) ) ;
#42643=VERTEX_POINT ( 'NONE', #17036 ) ;
#42659=CARTESIAN_POINT ( 'NONE',  ( -6.252266492314999979, 1511.741868877540128, 200.3335294429169835 ) ) ;
#42670=VERTEX_POINT ( 'NONE', #2521 ) ;
#42686=CARTESIAN_POINT ( 'NONE',  ( -1.716392779905000054, 1516.788317650260069, 206.2580580763669786 ) ) ;
#42707=ADVANCED_FACE ( 'NONE', ( #66824 ), #109905, .T. ) ;
#42730=CARTESIAN_POINT ( 'NONE',  ( 14.11150867580459511, 1517.034034075909631, 192.1634499395738942 ) ) ;
#42734=CARTESIAN_POINT ( 'NONE',  ( -7.500000019064999357, 1516.934643012909874, 209.1218459511669892 ) ) ;
#42737=CARTESIAN_POINT ( 'NONE',  ( 7.326795523374999952, 1516.760434454289907, 203.3416138547669902 ) ) ;
#42745=ORIENTED_EDGE ( 'NONE', *, *, #35885, .F. ) ;
#42748=VERTEX_POINT ( 'NONE', #33732 ) ;
#42764=CARTESIAN_POINT ( 'NONE',  ( 8.308248917014999790, 1512.693483295309989, 202.0206284635169993 ) ) ;
#42777=CYLINDRICAL_SURFACE ( 'NONE', #40327, 0.4999999999999449329 ) ;
#42780=CARTESIAN_POINT ( 'NONE',  ( 1.118353215965000036, 1516.977201124959947, 206.6281488911770055 ) ) ;
#42787=CARTESIAN_POINT ( 'NONE',  ( 7.304088249714999925, 1513.265135866640094, 216.6543191384870113 ) ) ;
#42796=CARTESIAN_POINT ( 'NONE',  ( -7.713117841115000317, 1516.690345681169902, 214.1262880092169780 ) ) ;
#42797=B_SPLINE_CURVE_WITH_KNOTS ( 'NONE', 5,
 ( #73364, #107502, #21815, #5043, #48170, #39188 ),
 .UNSPECIFIED., .F., .F.,
 ( 6, 6 ),
 ( 0.000000000000000000, 1.000000000000000000 ),
 .UNSPECIFIED. ) ;
#42800=CARTESIAN_POINT ( 'NONE',  ( 5.513207777283239963, 1508.731180391410135, 216.5668095921479903 ) ) ;
#42801=CARTESIAN_POINT ( 'NONE',  ( -1.700706814495000163, 1516.923170579120097, 211.4225755968969906 ) ) ;
#42820=CARTESIAN_POINT ( 'NONE',  ( 4.613762356885000138, 1516.939574742129935, 203.3372076122869885 ) ) ;
#42856=( BOUNDED_CURVE ( )  B_SPLINE_CURVE ( 3, ( #93529, #109799, #50461, #59417 ),
 .UNSPECIFIED., .F., .F. ) 
 B_SPLINE_CURVE_WITH_KNOTS ( ( 4, 4 ),
 ( 5.097274837781307077, 5.883015582180852299 ),
 .UNSPECIFIED. ) 
 CURVE ( )  GEOMETRIC_REPRESENTATION_ITEM ( )  RATIONAL_B_SPLINE_CURVE ( ( 1.000000000000000000, 0.9492093126141469828, 0.9492093126141469828, 1.000000000000000000 ) ) 
 REPRESENTATION_ITEM ( '' )  );
#42882=CARTESIAN_POINT ( 'NONE',  ( 7.469839230337810498, 1510.808998942815151, 202.9715998142987985 ) ) ;
#42890=DIRECTION ( 'NONE',  ( 0.000000000000000000, 0.000000000000000000, 1.000000000000000000 ) ) ;
#42902=LINE ( 'NONE', #58603, #96640 ) ;
#42904=CARTESIAN_POINT ( 'NONE',  ( -6.549762485114999144, 1516.729202374750002, 213.7405950387170037 ) ) ;
#42911=CARTESIAN_POINT ( 'NONE',  ( 3.451033388965000004, 1517.025653221279981, 203.3353183697670090 ) ) ;
#42928=CARTESIAN_POINT ( 'NONE',  ( 4.624736859184999993, 1516.994127245590107, 211.9896495963369887 ) ) ;
#42932=CARTESIAN_POINT ( 'NONE',  ( 5.781585778145000631, 1516.939646076049939, 209.1093989964429909 ) ) ;
#42947=CARTESIAN_POINT ( 'NONE',  ( 3.265407117845000151, 1516.754149861460064, 213.7315192116670062 ) ) ;
#42950=CARTESIAN_POINT ( 'NONE',  ( -6.554778571775000451, 1516.929962200689943, 216.8412383526069789 ) ) ;
#42966=EDGE_CURVE ( 'NONE', #43145, #2720, #88436, .T. ) ;
#42993=EDGE_LOOP ( 'NONE', ( #97822, #36987, #5588, #104733 ) ) ;
#43018=LINE ( 'NONE', #51407, #91574 ) ;
#43026=CARTESIAN_POINT ( 'NONE',  ( -8.723513748773688903, 1511.461300288249959, 214.7083397760629850 ) ) ;
#43032=CARTESIAN_POINT ( 'NONE',  ( -0.7468175536419978666, 1517.006509894990131, 209.1289748073840258 ) ) ;
#43042=CARTESIAN_POINT ( 'NONE',  ( -14.86025866229079995, 1514.013728165539987, 223.9912627551279911 ) ) ;
#43043=FACE_OUTER_BOUND ( 'NONE', #10126, .T. ) ;
#43064=CARTESIAN_POINT ( 'NONE',  ( 4.609064303374999838, 1516.723920667490120, 206.2441009858569885 ) ) ;
#43092=CLOSED_SHELL ( 'NONE', ( #80232, #61878, #71595, #83659, #43713, #56991, #64610, #43213, #54197, #22031, #78967, #19387, #43979, #23700, #13357, #79872, #32868, #82246, #90576, #60165, #89807, #105744, #18887, #109678, #4170, #77849, #22890, #56473, #33845, #58221, #84950, #11068, #58658, #32297, #66541, #5410, #109221, #33942, #99412, #19930, #94747, #78455, #58938, #9648, #42707, #2956, #110728, #64671, #47773, #45248, #52186, #76954, #86702, #7639, #89163, #90737, #14477, #1558, #68732, #28252, #29008, #50024, #6869, #78342, #29506, #54437, #14599, #27361, #31161, #85011, #36658, #41803, #11826, #88618, #61021, #68704, #62835, #86822, #8488, #37892, #16898, #103100, #50786, #17634, #34311, #102782, #93701, #109002, #57755, #85705, #48652, #14522, #104112, #68882, #44708, #88325, #14459, #49534, #102680, #85165, #109361, #69508, #58654, #45414, #83141, #37103 ) ) ;
#43114=CARTESIAN_POINT ( 'NONE',  ( -5.773668852974999766, 1516.734985836460055, 213.1604834329569940 ) ) ;
#43145=VERTEX_POINT ( 'NONE', #105802 ) ;
#43150=DIRECTION ( 'NONE',  ( 0.000000000000000000, -1.000000000000000000, 6.123233995736769734E-17 ) ) ;
#43158=CARTESIAN_POINT ( 'NONE',  ( -7.724732447025000504, 1517.133889586189980, 205.8614888033369823 ) ) ;
#43167=CARTESIAN_POINT ( 'NONE',  ( -16.78391011319079951, 1513.564960623335764, 222.3707652303824318 ) ) ;
#43173=CARTESIAN_POINT ( 'NONE',  ( 1.717432448265000078, 1516.836638729160086, 211.4041475482669910 ) ) ;
#43196=CARTESIAN_POINT ( 'NONE',  ( 5.984345098296709686, 1508.551704613440052, 202.1093217104930204 ) ) ;
#43203=CARTESIAN_POINT ( 'NONE',  ( -0.01244697378919850002, 1516.939646076049939, 203.3402601539570185 ) ) ;
#43204=CARTESIAN_POINT ( 'NONE',  ( -7.337297350114999617, 1517.135701590510052, 208.3821536943570152 ) ) ;
#43213=ADVANCED_FACE ( 'NONE', ( #5529 ), #91729, .F. ) ;
#43227=ORIENTED_EDGE ( 'NONE', *, *, #98682, .T. ) ;
#43242=CARTESIAN_POINT ( 'NONE',  ( -15.99263756166499917, 1514.225267046429963, 224.1757580215669918 ) ) ;
#43247=CARTESIAN_POINT ( 'NONE',  ( -5.788097265284999793, 1517.099836525840146, 206.6397780718770036 ) ) ;
#43262=CARTESIAN_POINT ( 'NONE',  ( -2.258825589925000266, 1511.942942747529969, 201.5330432499970073 ) ) ;
#43269=CARTESIAN_POINT ( 'NONE',  ( -7.500000019064999357, 1516.934643012909874, 209.1218459511669892 ) ) ;
#43270=CARTESIAN_POINT ( 'NONE',  ( -14.81821971718517439, 1514.585417787315237, 192.8869359013385747 ) ) ;
#43298=CARTESIAN_POINT ( 'NONE',  ( -5.782749439735000330, 1516.858301627840092, 203.3453548368569841 ) ) ;
#43324=CARTESIAN_POINT ( 'NONE',  ( 2.493699768634999536, 1516.858326417339867, 211.5985794462469869 ) ) ;
#43327=CARTESIAN_POINT ( 'NONE',  ( 6.321172833974999961, 1513.830194289060273, 201.5514268169769991 ) ) ;
#43337=CARTESIAN_POINT ( 'NONE',  ( -4.616272334694999202, 1517.030858226499959, 216.4568033268070053 ) ) ;
#43338=CARTESIAN_POINT ( 'NONE',  ( -8.220050563718016789, 1511.455710047913726, 213.1985981866891677 ) ) ;
#43342=CARTESIAN_POINT ( 'NONE',  ( 4.987078416394999714, 1509.051704408389924, 209.1727295022979831 ) ) ;
#43344=CARTESIAN_POINT ( 'NONE',  ( -5.012317106364999830, 1517.020727862619879, 206.2534121335969814 ) ) ;
#43350=CARTESIAN_POINT ( 'NONE',  ( 7.869278964325000736, 1514.500328598809801, 215.5039757893969750 ) ) ;
#43361=CARTESIAN_POINT ( 'NONE',  ( 3.262264650305000124, 1516.633288330999903, 215.6694029015669969 ) ) ;
#43365=CARTESIAN_POINT ( 'NONE',  ( 0.01323701367210150005, 1516.939658295650133, 211.6080660720070341 ) ) ;
#43373=FACE_OUTER_BOUND ( 'NONE', #79490, .T. ) ;
#43380=ORIENTED_EDGE ( 'NONE', *, *, #180, .T. ) ;
#43381=CARTESIAN_POINT ( 'NONE',  ( -7.720650173434999708, 1516.977993847330026, 203.3422188780170075 ) ) ;
#43395=DIRECTION ( 'NONE',  ( -0.01484500364079610613, 0.5669078173018522460, 0.8236474686107853049 ) ) ;
#43418=ORIENTED_EDGE ( 'NONE', *, *, #5526, .T. ) ;
#43436=CARTESIAN_POINT ( 'NONE',  ( 7.550704948200230859, 1510.491946830140705, 203.5278907278841700 ) ) ;
#43456=EDGE_CURVE ( 'NONE', #36699, #40040, #30318, .T. ) ;
#43459=CARTESIAN_POINT ( 'NONE',  ( 3.459156578084999989, 1516.769879638719885, 213.7318425517769924 ) ) ;
#43466=CARTESIAN_POINT ( 'NONE',  ( 3.257220602695000355, 1517.040132827679827, 203.3350082531769942 ) ) ;
#43469=CARTESIAN_POINT ( 'NONE',  ( -7.683535681777359905, 1517.051704408389924, 208.6863461652989997 ) ) ;
#43483=CARTESIAN_POINT ( 'NONE',  ( 7.337153768115000751, 1517.119374999550018, 212.3815752680669959 ) ) ;
#43487=CARTESIAN_POINT ( 'NONE',  ( -4.044319925355000400, 1517.073005577650065, 208.0013022344469960 ) ) ;
#43495=DIRECTION ( 'NONE',  ( 0.9996573249755517088, -0.02617694830808747070, 0.000000000000000000 ) ) ;
#43502=CARTESIAN_POINT ( 'NONE',  ( -6.549762485114999144, 1516.729202374750002, 213.7405950387170037 ) ) ;
#43505=CARTESIAN_POINT ( 'NONE',  ( -7.329303116114999739, 1516.857992118400034, 216.4524001036569985 ) ) ;
#43506=EDGE_LOOP ( 'NONE', ( #105005, #31323, #62679 ) ) ;
#43534=LINE ( 'NONE', #444, #45137 ) ;
#43539=CARTESIAN_POINT ( 'NONE',  ( -1.458596267000419999, 1516.574598972179956, 201.4117590633649968 ) ) ;
#43548=LINE ( 'NONE', #50838, #52875 ) ;
#43583=CARTESIAN_POINT ( 'NONE',  ( 4.623892060624999800, 1517.066898074209803, 209.8584071487349831 ) ) ;
#43588=ORIENTED_EDGE ( 'NONE', *, *, #50906, .F. ) ;
#43599=CARTESIAN_POINT ( 'NONE',  ( 3.449647440015000122, 1516.829948096479939, 208.3645479958780129 ) ) ;
#43609=EDGE_CURVE ( 'NONE', #68294, #85474, #49808, .T. ) ;
#43616=CARTESIAN_POINT ( 'NONE',  ( 7.710285837685000310, 1516.582197289609894, 205.8614676770269796 ) ) ;
#43618=VERTEX_POINT ( 'NONE', #108684 ) ;
#43620=CARTESIAN_POINT ( 'NONE',  ( -5.761714458496140168, 1516.919864955513731, 204.2610115332772409 ) ) ;
#43662=CARTESIAN_POINT ( 'NONE',  ( -4.028630622785000170, 1516.812923327049930, 212.5819478221170016 ) ) ;
#43700=CARTESIAN_POINT ( 'NONE',  ( -7.018605345631014458, 1516.569754971243356, 211.7654319798640188 ) ) ;
#43703=CARTESIAN_POINT ( 'NONE',  ( -13.62888597016050163, 1517.051704413129983, 226.2994540733420195 ) ) ;
#43704=CARTESIAN_POINT ( 'NONE',  ( -2.299656354225000143, 1516.843453247299749, 206.6453952679669896 ) ) ;
#43713=ADVANCED_FACE ( 'NONE', ( #73994 ), #5687, .F. ) ;
#43718=CARTESIAN_POINT ( 'NONE',  ( 2.493073829755000137, 1516.826109302209943, 211.9861720575370043 ) ) ;
#43747=CARTESIAN_POINT ( 'NONE',  ( 1.708102589285000139, 1517.199196846569976, 202.5572672468869939 ) ) ;
#43748=CARTESIAN_POINT ( 'NONE',  ( -4.042388539304999640, 1517.045004075700035, 208.3857484934819979 ) ) ;
#43751=CARTESIAN_POINT ( 'NONE',  ( 2.983377196939291043, 1512.076549611913379, 217.0139528183213997 ) ) ;
#43753=CARTESIAN_POINT ( 'NONE',  ( 4.487249753905000027, 1509.038615934169911, 212.6094383991670043 ) ) ;
#43769=ORIENTED_EDGE ( 'NONE', *, *, #106248, .F. ) ;
#43784=CARTESIAN_POINT ( 'NONE',  ( -16.46592305696500347, 1512.456207068040158, 220.8712538603669771 ) ) ;
#43788=CARTESIAN_POINT ( 'NONE',  ( 5.771149074885000729, 1516.616791731099966, 206.6334853027970269 ) ) ;
#43790=CARTESIAN_POINT ( 'NONE',  ( 7.269615798715341803, 1508.603735221739498, 214.6352815282469351 ) ) ;
#43806=CARTESIAN_POINT ( 'NONE',  ( -2.711770233124999763, 1512.058324472099912, 201.4383516934770171 ) ) ;
#43822=DIRECTION ( 'NONE',  ( 0.4999999999998399614, -0.7071067811867740582, -0.4999999999998399614 ) ) ;
#43843=CARTESIAN_POINT ( 'NONE',  ( 1.121383591734999907, 1517.104192383289956, 204.4960559556369901 ) ) ;
#43861=( BOUNDED_CURVE ( )  B_SPLINE_CURVE ( 3, ( #13644, #31572, #97136, #80341 ),
 .UNSPECIFIED., .F., .T. ) 
 B_SPLINE_CURVE_WITH_KNOTS ( ( 4, 4 ),
 ( 0.9002477009696591148, 1.144704976403996710 ),
 .UNSPECIFIED. ) 
 CURVE ( )  GEOMETRIC_REPRESENTATION_ITEM ( )  RATIONAL_B_SPLINE_CURVE ( ( 1.000000000000000000, 0.9950262502543076870, 0.9950262502543076870, 1.000000000000000000 ) ) 
 REPRESENTATION_ITEM ( '' )  );
#43866=CARTESIAN_POINT ( 'NONE',  ( 1.136004274065000041, 1516.815173273089840, 211.9874827793370287 ) ) ;
#43870=CARTESIAN_POINT ( 'NONE',  ( 7.843966614384998870, 1513.355826799099759, 201.5485691027769803 ) ) ;
#43876=CARTESIAN_POINT ( 'NONE',  ( -8.788316527315000570, 1511.741868877540128, 215.3741124244170067 ) ) ;
#43879=CARTESIAN_POINT ( 'NONE',  ( -5.779627092215000594, 1516.977993847330026, 216.8424961055369806 ) ) ;
#43886=CARTESIAN_POINT ( 'NONE',  ( 6.934528529765000116, 1516.588006113850042, 206.2478870805069846 ) ) ;
#43891=CARTESIAN_POINT ( 'NONE',  ( -5.513211403820640122, 1508.731183031489991, 201.6768811751110206 ) ) ;
#43904=CARTESIAN_POINT ( 'NONE',  ( -6.551643424905000401, 1516.807958722750072, 214.9033365145770063 ) ) ;
#43908=CARTESIAN_POINT ( 'NONE',  ( 0.7579843820170020230, 1516.883361325900069, 211.4083188566570186 ) ) ;
#43924=CARTESIAN_POINT ( 'NONE',  ( 2.480187016714999970, 1517.025470194390209, 204.4964864072570094 ) ) ;
#43952=DIRECTION ( 'NONE',  ( -0.02616798426500960631, -0.9993150019883682011, -0.02616798426500960631 ) ) ;
#43974=DIRECTION ( 'NONE',  ( 0.9996573249755574819, -0.02617694830786557875, 0.000000000000000000 ) ) ;
#43979=ADVANCED_FACE ( 'NONE', ( #61488 ), #84988, .F. ) ;
#43994=CARTESIAN_POINT ( 'NONE',  ( 7.717505752974999744, 1516.857914730730045, 216.8393517232070167 ) ) ;
#44008=CARTESIAN_POINT ( 'NONE',  ( -3.448206916814999801, 1516.904492006980036, 213.1642637479369853 ) ) ;
#44009=CARTESIAN_POINT ( 'NONE',  ( 4.522891059284999571, 1511.193640125469983, 216.9700256452169924 ) ) ;
#44017=CARTESIAN_POINT ( 'NONE',  ( -7.721907926364999675, 1517.026025493960105, 204.1173703575669833 ) ) ;
#44019=CARTESIAN_POINT ( 'NONE',  ( -2.930838077694999821, 1510.983859056260144, 201.5581577403170002 ) ) ;
#44030=CARTESIAN_POINT ( 'NONE',  ( -2.864326125434999870, 1516.826109302209943, 211.6149197999869784 ) ) ;
#44035=CARTESIAN_POINT ( 'NONE',  ( 6.550870144104999682, 1516.727502608469877, 208.3674577492799926 ) ) ;
#44043=CYLINDRICAL_SURFACE ( 'NONE', #54966, 0.5000000000000022204 ) ;
#44051=CARTESIAN_POINT ( 'NONE',  ( 4.618749068485000109, 1516.729202374750002, 215.6716084172169872 ) ) ;
#44063=CARTESIAN_POINT ( 'NONE',  ( 7.950581774744748920, 1511.645396655840159, 203.1073707467290319 ) ) ;
#44092=CARTESIAN_POINT ( 'NONE',  ( -2.691174921192619696, 1516.547507499529956, 201.4124685881550079 ) ) ;
#44140=CARTESIAN_POINT ( 'NONE',  ( -3.449647478144999724, 1516.829948096479939, 209.8791439064560223 ) ) ;
#44150=CARTESIAN_POINT ( 'NONE',  ( 6.942354273414999888, 1516.905946377369901, 201.4030824261969883 ) ) ;
#44156=CARTESIAN_POINT ( 'NONE',  ( 5.000329995535000016, 1516.770163853809890, 208.3657552043160024 ) ) ;
#44160=VERTEX_POINT ( 'NONE', #46351 ) ;
#44161=VERTEX_POINT ( 'NONE', #105694 ) ;
#44173=CARTESIAN_POINT ( 'NONE',  ( -4.042729840925000317, 1516.919782530640077, 205.8674445284970034 ) ) ;
#44183=DIRECTION ( 'NONE',  ( -0.6742693640208961003, 0.000000000000000000, -0.7384854939285241393 ) ) ;
#44192=CARTESIAN_POINT ( 'NONE',  ( 0.7560907277860019482, 1516.770163853809890, 214.1221759657669850 ) ) ;
#44199=DIRECTION ( 'NONE',  ( -0.01484500364079635246, -0.5669078173018518019, 0.8236474686107856380 ) ) ;
#44206=EDGE_CURVE ( 'NONE', #65542, #4206, #79378, .T. ) ;
#44222=CARTESIAN_POINT ( 'NONE',  ( 5.010422963235000360, 1516.929569650079884, 213.1529883219070030 ) ) ;
#44232=ORIENTED_EDGE ( 'NONE', *, *, #66245, .T. ) ;
#44262=CARTESIAN_POINT ( 'NONE',  ( -7.078000874848796364, 1516.557769095839603, 211.6025370379481672 ) ) ;
#44267=CARTESIAN_POINT ( 'NONE',  ( -4.043990345725000601, 1516.983612918759945, 206.6425990843970055 ) ) ;
#44276=CARTESIAN_POINT ( 'NONE',  ( 13.49160166387382453, 1516.729020965289010, 192.0695843282071849 ) ) ;
#44280=CARTESIAN_POINT ( 'NONE',  ( -2.477373643995000485, 1516.891731298979948, 212.0030687278169808 ) ) ;
#44303=CARTESIAN_POINT ( 'NONE',  ( 5.513222313296060051, 1508.611138448520023, 201.8002184229020202 ) ) ;
#44307=CARTESIAN_POINT ( 'NONE',  ( 3.452289182574999948, 1517.069378699710114, 202.5601595088670024 ) ) ;
#44308=CARTESIAN_POINT ( 'NONE',  ( 7.339107202615000602, 1517.203017563489766, 210.2473558205170150 ) ) ;
#44313=CARTESIAN_POINT ( 'NONE',  ( 5.513435558552500559, 1508.909942010212490, 201.6124651694741488 ) ) ;
#44322=CARTESIAN_POINT ( 'NONE',  ( -2.956771579574999809, 1512.877808311729950, 201.2153269223470033 ) ) ;
#44345=CARTESIAN_POINT ( 'NONE',  ( 12.38398709303499956, 1512.136030808819896, 224.0418830982669931 ) ) ;
#44349=CARTESIAN_POINT ( 'NONE',  ( -16.44145560006500162, 1512.902436350919970, 220.7137343290669946 ) ) ;
#44354=CARTESIAN_POINT ( 'NONE',  ( 1.701027822874999984, 1516.937508036699910, 206.6270879340970055 ) ) ;
#44361=DIRECTION ( 'NONE',  ( 0.7071067811865475727, 2.497298964526426743E-16, 0.7071067811865475727 ) ) ;
#44372=CARTESIAN_POINT ( 'NONE',  ( -3.167889856915000024, 1511.297452611760036, 201.5028532582269918 ) ) ;
#44398=CARTESIAN_POINT ( 'NONE',  ( -7.508705023303230419, 1508.884117426920056, 214.6350462346350128 ) ) ;
#44407=CARTESIAN_POINT ( 'NONE',  ( -2.877744984375000037, 1516.723920667490120, 204.5127816287269980 ) ) ;
#44427=CARTESIAN_POINT ( 'NONE',  ( 3.461360093275000160, 1516.874084700499907, 212.3753080308970311 ) ) ;
#44430=CARTESIAN_POINT ( 'NONE',  ( 6.715925843064999512, 1514.199187793459942, 201.3425812415170242 ) ) ;
#44437=CARTESIAN_POINT ( 'NONE',  ( -6.781132916885000306, 1512.686126173240154, 216.3888413780769895 ) ) ;
#44448=CARTESIAN_POINT ( 'NONE',  ( -3.268235758764999943, 1516.890356958860139, 206.2562572478169898 ) ) ;
#44453=CARTESIAN_POINT ( 'NONE',  ( -7.321630743333059854, 1508.611141564370200, 203.6086204835860087 ) ) ;
#44464=CARTESIAN_POINT ( 'NONE',  ( -6.939219520934999608, 1516.783701990830195, 214.9027072062869763 ) ) ;
#44467=CARTESIAN_POINT ( 'NONE',  ( 5.822794770344668969, 1511.432897564909808, 217.0586008862449887 ) ) ;
#44469=CARTESIAN_POINT ( 'NONE',  ( 6.562635822504999439, 1517.111322026010157, 211.9927976380170094 ) ) ;
#44477=CARTESIAN_POINT ( 'NONE',  ( -7.594039287445000674, 1512.142919181319940, 211.3515775794370199 ) ) ;
#44486=CARTESIAN_POINT ( 'NONE',  ( -2.488360667435000284, 1516.616791731099966, 203.3506968572170308 ) ) ;
#44528=CARTESIAN_POINT ( 'NONE',  ( 7.329303077985000137, 1516.857992118400034, 201.7912917986770083 ) ) ;
#44533=CARTESIAN_POINT ( 'NONE',  ( 7.588802682105000308, 1511.942942747529969, 206.8630203803070060 ) ) ;
#44561=CARTESIAN_POINT ( 'NONE',  ( -4.999456428534999830, 1516.830644417779922, 213.7431138541670066 ) ) ;
#44562=CARTESIAN_POINT ( 'NONE',  ( 2.229731609205000353, 1512.142919181319940, 216.7158852195469763 ) ) ;
#44563=ORIENTED_EDGE ( 'NONE', *, *, #34619, .F. ) ;
#44569=CARTESIAN_POINT ( 'NONE',  ( 4.612507273904999039, 1516.886345593249871, 204.1123678647870179 ) ) ;
#44585=CARTESIAN_POINT ( 'NONE',  ( -3.251888867474999945, 1516.793978928989873, 211.6142896211370044 ) ) ;
#44591=CARTESIAN_POINT ( 'NONE',  ( 2.292217010694999946, 1516.941178807709775, 209.1086494233340147 ) ) ;
#44610=CARTESIAN_POINT ( 'NONE',  ( -5.002593397454999646, 1516.960844870249957, 215.6810146069769871 ) ) ;
#44614=CARTESIAN_POINT ( 'NONE',  ( 6.554778533645000849, 1516.929962200689943, 201.4024535497269994 ) ) ;
#44622=CARTESIAN_POINT ( 'NONE',  ( 7.494431743707549387, 1510.714321716100130, 203.0291457976910010 ) ) ;
#44625=CARTESIAN_POINT ( 'NONE',  ( 7.821732060355000016, 1513.613303996360173, 216.8564630578470087 ) ) ;
#44638=DIRECTION ( 'NONE',  ( 0.7071067811865492381, 0.000000000000000000, 0.7071067811865457964 ) ) ;
#44651=CARTESIAN_POINT ( 'NONE',  ( -2.454407622921550125, 1516.534924556719943, 201.4127979744969821 ) ) ;
#44699=CARTESIAN_POINT ( 'NONE',  ( -1.704170752255000032, 1516.927039499179955, 209.8797722570040207 ) ) ;
#44704=EDGE_LOOP ( 'NONE', ( #76979, #3043, #13917, #38266 ) ) ;
#44708=ADVANCED_FACE ( 'NONE', ( #104437 ), #19468, .T. ) ;
#44716=CARTESIAN_POINT ( 'NONE',  ( -7.339749373344999661, 1517.224900789629828, 207.4124613591469881 ) ) ;
#44735=CARTESIAN_POINT ( 'NONE',  ( -3.461047329755000401, 1516.858765657450249, 205.6745815831370123 ) ) ;
#44740=CARTESIAN_POINT ( 'NONE',  ( 4.987078416414999715, 1508.551704408389924, 212.6094384009469707 ) ) ;
#44753=CARTESIAN_POINT ( 'NONE',  ( -5.773668852974999766, 1516.734985836460055, 213.1604834329569940 ) ) ;
#44760=CARTESIAN_POINT ( 'NONE',  ( 3.727807031261289872, 1517.051706634850007, 202.5053387368750180 ) ) ;
#44820=CARTESIAN_POINT ( 'NONE',  ( -8.656560647815000564, 1514.517422889970021, 203.9087166159570188 ) ) ;
#44823=CARTESIAN_POINT ( 'NONE',  ( -7.081311148617888129, 1516.557149304009954, 211.5931455169218793 ) ) ;
#44828=CARTESIAN_POINT ( 'NONE',  ( 1.118353215965000036, 1516.977201124959947, 206.6281488911770055 ) ) ;
#44839=CARTESIAN_POINT ( 'NONE',  ( 0.01328393942530149870, 1516.939580991450157, 212.3834982571270018 ) ) ;
#44840=( BOUNDED_CURVE ( )  B_SPLINE_CURVE ( 3, ( #12574, #106622, #29909, #1995 ),
 .UNSPECIFIED., .F., .F. ) 
 B_SPLINE_CURVE_WITH_KNOTS ( ( 4, 4 ),
 ( 1.282864256197260078, 2.438226007366384618 ),
 .UNSPECIFIED. ) 
 CURVE ( )  GEOMETRIC_REPRESENTATION_ITEM ( )  RATIONAL_B_SPLINE_CURVE ( ( 1.000000000000000000, 0.8918208900530331107, 0.8918208900530331107, 1.000000000000000000 ) ) 
 REPRESENTATION_ITEM ( '' )  );
#44871=CARTESIAN_POINT ( 'NONE',  ( -1.710004586925000236, 1516.557392317769882, 202.5758445815369839 ) ) ;
#44872=CARTESIAN_POINT ( 'NONE',  ( 7.339749335215000059, 1517.224900789629828, 210.8312305431869902 ) ) ;
#44895=CARTESIAN_POINT ( 'NONE',  ( -7.194888370995000670, 1513.142795523600171, 201.8217789698469744 ) ) ;
#44905=VERTEX_POINT ( 'NONE', #84735 ) ;
#44911=CARTESIAN_POINT ( 'NONE',  ( 10.96015508933500016, 1512.830284628050094, 225.0317485278669949 ) ) ;
#44919=CARTESIAN_POINT ( 'NONE',  ( -7.725372170364999569, 1517.158319634930194, 206.2490093095770192 ) ) ;
#44936=CARTESIAN_POINT ( 'NONE',  ( 5.818054393111782296, 1510.580107409934271, 216.6577242164569839 ) ) ;
#44969=CARTESIAN_POINT ( 'NONE',  ( -6.559798094425000059, 1516.987478262539980, 204.5068286042669854 ) ) ;
#44990=CARTESIAN_POINT ( 'NONE',  ( -4.609064341505000328, 1516.723920667490120, 211.9995909164769898 ) ) ;
#44996=VERTEX_POINT ( 'NONE', #16409 ) ;
#44999=ORIENTED_EDGE ( 'NONE', *, *, #87105, .F. ) ;
#45002=CARTESIAN_POINT ( 'NONE',  ( -7.660003975705000023, 1511.444830760690138, 215.2207434837270057 ) ) ;
#45003=CARTESIAN_POINT ( 'NONE',  ( 16.77006244281658809, 1513.317537412908678, 196.3881396080545585 ) ) ;
#45014=CARTESIAN_POINT ( 'NONE',  ( -0.01319654689839849966, 1516.941178807709775, 206.8296289214069930 ) ) ;
#45015=ORIENTED_EDGE ( 'NONE', *, *, #42532, .T. ) ;
#45024=CARTESIAN_POINT ( 'NONE',  ( 15.19278567220069931, 1512.351864386150055, 196.1968638649200329 ) ) ;
#45026=CARTESIAN_POINT ( 'NONE',  ( -6.089577322537190085, 1511.778877376279979, 200.6487354888959942 ) ) ;
#45033=CARTESIAN_POINT ( 'NONE',  ( -5.001338666445000136, 1516.911981270829983, 214.9058546054269812 ) ) ;
#45035=CARTESIAN_POINT ( 'NONE',  ( 6.013128406968769823, 1510.874996213040049, 216.6400301521790084 ) ) ;
#45037=CARTESIAN_POINT ( 'NONE',  ( -2.477373643995000485, 1516.891731298979948, 212.0030687278169808 ) ) ;
#45055=CARTESIAN_POINT ( 'NONE',  ( -6.945490086935000029, 1516.932669162149978, 203.3434733684869968 ) ) ;
#45099=CARTESIAN_POINT ( 'NONE',  ( -7.329925260535000042, 1516.833976295079992, 201.4049670291269933 ) ) ;
#45112=CARTESIAN_POINT ( 'NONE',  ( -7.550503362055001055, 1510.480349266450048, 214.6730346442070072 ) ) ;
#45129=CARTESIAN_POINT ( 'NONE',  ( -6.939219520934999608, 1516.783701990830195, 214.9027072062869763 ) ) ;
#45136=CARTESIAN_POINT ( 'NONE',  ( 1.121383591734999907, 1517.104192383289956, 204.4960559556369901 ) ) ;
#45137=VECTOR ( 'NONE', #110170, 1000.000000000000000 ) ;
#45150=CARTESIAN_POINT ( 'NONE',  ( -4.996642198295000448, 1516.697242742309982, 211.9989590406970024 ) ) ;
#45157=CARTESIAN_POINT ( 'NONE',  ( -5.006259886824999228, 1516.939723362869927, 209.1347437590049765 ) ) ;
#45168=CARTESIAN_POINT ( 'NONE',  ( 4.987078413254999454, 1508.551704408389924, 213.0804953801570036 ) ) ;
#45170=CARTESIAN_POINT ( 'NONE',  ( -3.258474617075000079, 1517.083030555940013, 215.6838419306269827 ) ) ;
#45180=CARTESIAN_POINT ( 'NONE',  ( 7.601092399332859628, 1510.855104182140167, 203.4698203236769984 ) ) ;
#45192=ORIENTED_EDGE ( 'NONE', *, *, #8680, .T. ) ;
#45208=CARTESIAN_POINT ( 'NONE',  ( 5.551188674472009588, 1510.480349264700180, 216.6723492941099778 ) ) ;
#45211=ORIENTED_EDGE ( 'NONE', *, *, #18478, .T. ) ;
#45218=EDGE_CURVE ( 'NONE', #55731, #72815, #107830, .T. ) ;
#45228=CARTESIAN_POINT ( 'NONE',  ( 15.20279577643499991, 1515.867682058960099, 225.0317485278669949 ) ) ;
#45248=ADVANCED_FACE ( 'NONE', ( #38955 ), #30007, .F. ) ;
#45258=CARTESIAN_POINT ( 'NONE',  ( 7.337297311985000015, 1517.135701590510052, 209.8615382079770200 ) ) ;
#45272=CARTESIAN_POINT ( 'NONE',  ( 4.610079833424999940, 1516.713079096360161, 207.9883289669969884 ) ) ;
#45287=CARTESIAN_POINT ( 'NONE',  ( 5.770883563884999568, 1516.603620185149794, 206.8276363026970159 ) ) ;
#45297=CARTESIAN_POINT ( 'NONE',  ( 7.326141149145000142, 1517.051704409989952, 213.3996074426069924 ) ) ;
#45308=CARTESIAN_POINT ( 'NONE',  ( 5.781490544344999982, 1516.807958722750072, 215.6734893570070142 ) ) ;
#45355=VECTOR ( 'NONE', #80439, 1000.000000000000000 ) ;
#45368=EDGE_LOOP ( 'NONE', ( #60113, #61780, #80081, #20973, #68162, #65626, #67230, #92043 ) ) ;
#45376=CARTESIAN_POINT ( 'NONE',  ( -5.380079384537971521, 1516.847814776033829, 214.3564748279252115 ) ) ;
#45382=CARTESIAN_POINT ( 'NONE',  ( 3.445685077385000294, 1516.778761582560037, 206.6297153089269898 ) ) ;
#45394=CARTESIAN_POINT ( 'NONE',  ( 4.043366220174999803, 1516.951766529250108, 211.9887038632370206 ) ) ;
#45398=CARTESIAN_POINT ( 'NONE',  ( 2.613924552144012647, 1516.542698303460384, 216.8310974888379405 ) ) ;
#45403=CARTESIAN_POINT ( 'NONE',  ( 14.24701162106355135, 1514.160701258722611, 225.6749658073803460 ) ) ;
#45414=ADVANCED_FACE ( 'NONE', ( #1293 ), #15836, .T. ) ;
#45415=CARTESIAN_POINT ( 'NONE',  ( 5.513200267037420055, 1508.884117426719968, 201.6131409466659932 ) ) ;
#45422=CARTESIAN_POINT ( 'NONE',  ( 5.774609621945000271, 1516.777260590120022, 204.5018377250270021 ) ) ;
#45442=EDGE_CURVE ( 'NONE', #107049, #21389, #5254, .T. ) ;
#45444=CARTESIAN_POINT ( 'NONE',  ( -7.585800469905000121, 1513.656171171920050, 202.9549341796069939 ) ) ;
#45447=AXIS2_PLACEMENT_3D ( 'NONE', #71864, #80769, #104313 ) ;
#45470=CARTESIAN_POINT ( 'NONE',  ( -5.014195139944999546, 1517.120861839400050, 207.4163795216369977 ) ) ;
#45490=CARTESIAN_POINT ( 'NONE',  ( -2.950959360024999700, 1512.115618635729788, 201.2383024395870166 ) ) ;
#45526=CARTESIAN_POINT ( 'NONE',  ( 1.704794803334999997, 1517.096587378560116, 204.4952540647470016 ) ) ;
#45535=ORIENTED_EDGE ( 'NONE', *, *, #62570, .T. ) ;
#45547=CARTESIAN_POINT ( 'NONE',  ( 7.724732408895000013, 1517.133889586189980, 212.3822030989969960 ) ) ;
#45551=ORIENTED_EDGE ( 'NONE', *, *, #82960, .T. ) ;
#45556=ORIENTED_EDGE ( 'NONE', *, *, #71079, .T. ) ;
#45557=CARTESIAN_POINT ( 'NONE',  ( -7.382751585984999920, 1511.929989569689951, 215.7327168677470013 ) ) ;
#45567=CARTESIAN_POINT ( 'NONE',  ( 1.117840086735000016, 1516.949031626070109, 207.4047068479870006 ) ) ;
#45578=CARTESIAN_POINT ( 'NONE',  ( -6.253177289296100838, 1511.742575854359984, 200.3335783645690071 ) ) ;
#45585=CARTESIAN_POINT ( 'NONE',  ( 4.618119666265000589, 1516.706638732659940, 216.0591847158069925 ) ) ;
#45587=CARTESIAN_POINT ( 'NONE',  ( 5.925858227311150195, 1511.532396045849964, 217.0681951087739776 ) ) ;
#45589=CARTESIAN_POINT ( 'NONE',  ( -2.284199401535000007, 1516.940296199220029, 212.3910308785969789 ) ) ;
#45593=ORIENTED_EDGE ( 'NONE', *, *, #7513, .F. ) ;
#45607=CARTESIAN_POINT ( 'NONE',  ( -3.457266643525000127, 1516.691414181030041, 203.3491180233569935 ) ) ;
#45611=B_SPLINE_CURVE_WITH_KNOTS ( 'NONE', 3,
 ( #81170, #63853, #29668, #37527, #54355, #12312, #46502, #2845, #71160, #98524, #20699, #96334, #80635, #12865, #54895, #21790, #105846, #29125, #19612, #97965, #97430, #55992, #47046, #90115, #30210, #21235, #53814, #4485, #45403, #88486, #38616, #3397, #64401, #13398, #38076, #55447, #71729, #105283, #87950, #11771, #3949, #63311, #45940, #79542, #47585, #89020, #2307, #36418, #70610, #72253 ),
 .UNSPECIFIED., .F., .F.,
 ( 4, 2, 2, 1, 1, 2, 2, 2, 2, 1, 1, 1, 2, 2, 2, 2, 1, 1, 1, 2, 2, 2, 2, 1, 1, 1, 1, 2, 2, 2, 4 ),
 ( 0.000000000000000000, 0.1250000000004282963, 0.1875000000006428469, 0.2187500000007644441, 0.2343750000008096579, 0.2421875000008512635, 0.2500000000008928414, 0.3750000000017443824, 0.4375000000021700974, 0.4687500000024091840, 0.4843750000025029423, 0.4921875000025491831, 0.4960937500025454638, 0.5000000000025417446, 0.6250000000030592195, 0.6875000000033516523, 0.7187500000034974246, 0.7343750000035393910, 0.7421875000035882408, 0.7460937500036100012, 0.7500000000036317616, 0.8125000000047263304, 0.8437500000052703397, 0.8593750000055055960, 0.8671875000056231686, 0.8710937500056854521, 0.8730468750057130967, 0.8740234375057269745, 0.8750000000057408522, 0.9375000000028704816, 1.000000000000000000 ),
 .UNSPECIFIED. ) ;
#45621=EDGE_CURVE ( 'NONE', #85474, #61609, #53361, .T. ) ;
#45649=CARTESIAN_POINT ( 'NONE',  ( -14.58906259456500010, 1513.961173499609913, 192.6975966445669712 ) ) ;
#45653=CARTESIAN_POINT ( 'NONE',  ( 0.7403205670290020635, 1517.139320148880188, 201.3969713189170250 ) ) ;
#45667=CARTESIAN_POINT ( 'NONE',  ( -7.556074100184999587, 1510.693074690949970, 213.9348573562170088 ) ) ;
#45686=CARTESIAN_POINT ( 'NONE',  ( 4.618749068485000109, 1516.729202374750002, 215.6716084172169872 ) ) ;
#45687=CARTESIAN_POINT ( 'NONE',  ( 2.942029631075000040, 1512.314860029340025, 217.0136234567869735 ) ) ;
#45693=CARTESIAN_POINT ( 'NONE',  ( 6.548821941055000373, 1516.688761843659904, 205.0844676760469838 ) ) ;
#45697=CARTESIAN_POINT ( 'NONE',  ( -1.708092304294999808, 1516.523379810429788, 201.4131002843170108 ) ) ;
#45699=CARTESIAN_POINT ( 'NONE',  ( -12.18971938666500066, 1512.123542805230272, 194.3960765485670095 ) ) ;
#45706=CARTESIAN_POINT ( 'NONE',  ( 0.01327404799950150129, 1516.939877939420057, 212.5773418040870126 ) ) ;
#45712=CARTESIAN_POINT ( 'NONE',  ( -7.719640941135000212, 1516.939452820819952, 209.1319487995289705 ) ) ;
#45727=CARTESIAN_POINT ( 'NONE',  ( 5.781490544344999982, 1516.807958722750072, 215.6734893570070142 ) ) ;
#45735=CARTESIAN_POINT ( 'NONE',  ( -14.84895963876500780, 1511.957228877180114, 221.1990661657671637 ) ) ;
#45737=CARTESIAN_POINT ( 'NONE',  ( 7.447811282559439583, 1511.198033794599951, 202.8566241436609801 ) ) ;
#45809=CARTESIAN_POINT ( 'NONE',  ( -7.323390445344999833, 1516.613712827999962, 210.2512321725070024 ) ) ;
#45811=DIRECTION ( 'NONE',  ( -0.7071067811865475727, -1.473812113707079158E-16, -0.7071067811865475727 ) ) ;
#45816=( BOUNDED_CURVE ( )  B_SPLINE_CURVE ( 3, ( #61844, #19797, #3588, #3040 ),
 .UNSPECIFIED., .F., .F. ) 
 B_SPLINE_CURVE_WITH_KNOTS ( ( 4, 4 ),
 ( 5.499719231357318883, 7.069826863760232172 ),
 .UNSPECIFIED. ) 
 CURVE ( )  GEOMETRIC_REPRESENTATION_ITEM ( )  RATIONAL_B_SPLINE_CURVE ( ( 1.000000000000000000, 0.8049001529976759217, 0.8049001529976759217, 1.000000000000000000 ) ) 
 REPRESENTATION_ITEM ( '' )  );
#45817=CARTESIAN_POINT ( 'NONE',  ( 5.003848121975000396, 1517.005755693489846, 201.7875176594370146 ) ) ;
#45822=CARTESIAN_POINT ( 'NONE',  ( -0.007128875282218469743, 1517.006509894990131, 208.3750284165899984 ) ) ;
#45833=CARTESIAN_POINT ( 'NONE',  ( 7.717505752974999744, 1516.857914730730045, 216.8393517232070167 ) ) ;
#45838=CARTESIAN_POINT ( 'NONE',  ( -0.01323705180209850014, 1516.939658295650133, 206.6356258303270010 ) ) ;
#45855=CARTESIAN_POINT ( 'NONE',  ( -2.870951705914999597, 1517.111322026010157, 215.6844817927369888 ) ) ;
#45862=FACE_OUTER_BOUND ( 'NONE', #84244, .T. ) ;
#45873=DIRECTION ( 'NONE',  ( 1.000000000000000000, 0.000000000000000000, 0.000000000000000000 ) ) ;
#45921=CARTESIAN_POINT ( 'NONE',  ( 5.771149074885000729, 1516.616791731099966, 206.6334853027970269 ) ) ;
#45940=CARTESIAN_POINT ( 'NONE',  ( 14.78981622368054971, 1514.562529184305731, 225.3765129853291000 ) ) ;
#45959=CARTESIAN_POINT ( 'NONE',  ( -6.559168674874999105, 1516.960844870249957, 204.1192525727769862 ) ) ;
#45963=CARTESIAN_POINT ( 'NONE',  ( 4.487249753905000027, 1509.038615934169911, 212.6094383991670043 ) ) ;
#45985=CARTESIAN_POINT ( 'NONE',  ( -6.396410548735000035, 1511.623805160490065, 201.6463516768869795 ) ) ;
#46001=CARTESIAN_POINT ( 'NONE',  ( 14.28353071843499933, 1513.113451381389950, 224.7690913644670161 ) ) ;
#46011=CARTESIAN_POINT ( 'NONE',  ( -7.338753868364999988, 1517.184383877180153, 206.8309596656170015 ) ) ;
#46034=FACE_OUTER_BOUND ( 'NONE', #66616, .T. ) ;
#46042=CARTESIAN_POINT ( 'NONE',  ( 7.559010162000579847, 1510.805212306241174, 203.6254155100018011 ) ) ;
#46049=CYLINDRICAL_SURFACE ( 'NONE', #9052, 0.9999999999999988898 ) ;
#46070=CARTESIAN_POINT ( 'NONE',  ( -2.296124889065000119, 1516.677239312369920, 204.5136991508470032 ) ) ;
#46092=CARTESIAN_POINT ( 'NONE',  ( 7.337153768115000751, 1517.119374999550018, 212.3815752680669959 ) ) ;
#46095=ORIENTED_EDGE ( 'NONE', *, *, #4288, .T. ) ;
#46100=VERTEX_POINT ( 'NONE', #46218 ) ;
#46103=CARTESIAN_POINT ( 'NONE',  ( -7.750386781025000893, 1513.342361861140034, 216.5914658619369959 ) ) ;
#46115=CARTESIAN_POINT ( 'NONE',  ( -3.269184946495000244, 1516.940296199220029, 206.8376465686969823 ) ) ;
#46122=CARTESIAN_POINT ( 'NONE',  ( -7.507422039880669473, 1508.880866118479844, 202.9817282009999815 ) ) ;
#46126=CARTESIAN_POINT ( 'NONE',  ( 14.89373265416590009, 1512.150422497879845, 196.7424079551790044 ) ) ;
#46128=CARTESIAN_POINT ( 'NONE',  ( -5.949235733474299792, 1511.655824793919919, 200.8322428604340075 ) ) ;
#46137=CARTESIAN_POINT ( 'NONE',  ( 5.780232077335000440, 1516.760434454289907, 216.4486414936069991 ) ) ;
#46141=CARTESIAN_POINT ( 'NONE',  ( 5.784678349096259886, 1511.501844456730169, 217.8912146184260052 ) ) ;
#46142=CARTESIAN_POINT ( 'NONE',  ( 2.686321661465695065, 1516.547182400040128, 216.8312149107646576 ) ) ;
#46143=CARTESIAN_POINT ( 'NONE',  ( 3.268235720634999897, 1516.890356958860139, 211.9874346545169885 ) ) ;
#46159=CARTESIAN_POINT ( 'NONE',  ( -4.041472511874999896, 1516.858649670339901, 205.0922732913970208 ) ) ;
#46171=CARTESIAN_POINT ( 'NONE',  ( 8.648691725468450997, 1514.216922324319739, 214.7715657207340030 ) ) ;
#46195=CARTESIAN_POINT ( 'NONE',  ( -13.50445036796499920, 1512.655881406850085, 193.7448231092670028 ) ) ;
#46199=CARTESIAN_POINT ( 'NONE',  ( 3.260357128764999946, 1517.133889586189980, 201.3971135232069969 ) ) ;
#46203=CARTESIAN_POINT ( 'NONE',  ( 7.772759690054999560, 1512.089957059379913, 206.2799139137070199 ) ) ;
#46209=DIRECTION ( 'NONE',  ( 0.6742693640212139572, 4.521919481779819710E-17, 0.7384854939282339270 ) ) ;
#46213=CARTESIAN_POINT ( 'NONE',  ( -7.559010200714999961, 1510.805212328559946, 214.6182764915270127 ) ) ;
#46218=CARTESIAN_POINT ( 'NONE',  ( 3.487592428935230249, 1508.551704408389924, 214.1089243929580164 ) ) ;
#46220=FILL_AREA_STYLE ('',( #12592 ) ) ;
#46236=CARTESIAN_POINT ( 'NONE',  ( 3.262264650305000124, 1516.633288330999903, 215.6694029015669969 ) ) ;
#46237=CARTESIAN_POINT ( 'NONE',  ( 3.481979419164999978, 1511.353635254350138, 216.8568855192669957 ) ) ;
#46243=AXIS2_PLACEMENT_3D ( 'NONE', #32613, #30951, #57294 ) ;
#46246=CARTESIAN_POINT ( 'NONE',  ( 2.866857893004999713, 1516.951766529250108, 205.0784797119270024 ) ) ;
#46255=DIRECTION ( 'NONE',  ( -0.7063774289747313251, 0.04540766091858282338, 0.7063774289747313251 ) ) ;
#46261=CARTESIAN_POINT ( 'NONE',  ( -3.447264387095000160, 1516.858765657450249, 212.5828932618570093 ) ) ;
#46268=CARTESIAN_POINT ( 'NONE',  ( -2.286472924554999953, 1516.883361325900069, 209.8798303522490016 ) ) ;
#46273=CARTESIAN_POINT ( 'NONE',  ( -5.513435801945663961, 1508.611350399025241, 201.8000010755221751 ) ) ;
#46280=FACE_OUTER_BOUND ( 'NONE', #39772, .T. ) ;
#46283=CARTESIAN_POINT ( 'NONE',  ( 5.780861236055000241, 1516.783701990830195, 216.0610654530370027 ) ) ;
#46288=CARTESIAN_POINT ( 'NONE',  ( 1.124894050234999998, 1517.194816588360027, 202.1703287997270309 ) ) ;
#46295=CARTESIAN_POINT ( 'NONE',  ( 8.795036018429138736, 1511.645100227929788, 202.9941036799409915 ) ) ;
#46323=CARTESIAN_POINT ( 'NONE',  ( 0.3712394671979279970, 1517.036116044630262, 201.3996746346359714 ) ) ;
#46326=CARTESIAN_POINT ( 'NONE',  ( 13.89676589599709899, 1513.004579589660125, 224.4119314900950144 ) ) ;
#46338=AXIS2_PLACEMENT_3D ( 'NONE', #40696, #49668, #39026 ) ;
#46347=VERTEX_POINT ( 'NONE', #67150 ) ;
#46351=CARTESIAN_POINT ( 'NONE',  ( -12.18971938666500066, 1512.123542805230272, 194.3960765485670095 ) ) ;
#46363=CARTESIAN_POINT ( 'NONE',  ( 5.014195101815000832, 1517.120861839400050, 210.8273123806970091 ) ) ;
#46364=CARTESIAN_POINT ( 'NONE',  ( -7.454017790216410866, 1508.783371651619063, 203.6084103740970193 ) ) ;
#46372=CARTESIAN_POINT ( 'NONE',  ( -2.485846037024999955, 1516.545806094630279, 201.8003900583769905 ) ) ;
#46374=MECHANICAL_DESIGN_GEOMETRIC_PRESENTATION_REPRESENTATION('',(#60686),#17688);
#46397=CARTESIAN_POINT ( 'NONE',  ( 7.321455873725000174, 1516.545806094630279, 206.6359999332069890 ) ) ;
#46413=CARTESIAN_POINT ( 'NONE',  ( 2.294209629405000062, 1516.603620185149794, 214.8927295341169952 ) ) ;
#46429=ORIENTED_EDGE ( 'NONE', *, *, #61773, .T. ) ;
#46435=AXIS2_PLACEMENT_3D ( 'NONE', #35507, #69700, #103819 ) ;
#46457=DIRECTION ( 'NONE',  ( 0.02616798426500960631, 0.9993150019883682011, 0.02616798426500960631 ) ) ;
#46481=CARTESIAN_POINT ( 'NONE',  ( 1.700259675955000160, 1516.898441858519845, 207.4036424686470070 ) ) ;
#46500=ORIENTED_EDGE ( 'NONE', *, *, #60946, .T. ) ;
#46502=CARTESIAN_POINT ( 'NONE',  ( 11.88248411615536071, 1513.001574290550934, 225.6614044502198340 ) ) ;
#46518=CARTESIAN_POINT ( 'NONE',  ( -1.711311266675000109, 1516.591755933730155, 203.3510257909670145 ) ) ;
#46540=CARTESIAN_POINT ( 'NONE',  ( -6.044020076205000258, 1511.752511073100095, 200.8248430530570090 ) ) ;
#46554=CARTESIAN_POINT ( 'NONE',  ( 12.80694033583499980, 1512.080583811389943, 224.7218690204669826 ) ) ;
#46564=CARTESIAN_POINT ( 'NONE',  ( -1.718203501584999904, 1516.898441858519845, 207.4215862561470090 ) ) ;
#46623=CARTESIAN_POINT ( 'NONE',  ( -1.714334285315000095, 1516.699825673279975, 205.0952314524469955 ) ) ;
#46653=CARTESIAN_POINT ( 'NONE',  ( -5.763076042985000313, 1514.407352313670117, 216.7876711347169874 ) ) ;
#46654=CARTESIAN_POINT ( 'NONE',  ( 16.66011979181740443, 1513.969110093212976, 195.1663535919080914 ) ) ;
#46665=CARTESIAN_POINT ( 'NONE',  ( -4.045182518055000287, 1517.057265928030120, 207.4180663268770104 ) ) ;
#46677=CARTESIAN_POINT ( 'NONE',  ( -5.619918030323759695, 1511.009256124219974, 201.4419183480959816 ) ) ;
#46683=CARTESIAN_POINT ( 'NONE',  ( 2.486474742745000022, 1516.560253536979872, 216.0557253731069807 ) ) ;
#46688=CARTESIAN_POINT ( 'NONE',  ( -4.609064341505000328, 1516.723920667490120, 211.9995909164769898 ) ) ;
#46705=CARTESIAN_POINT ( 'NONE',  ( 1.703779605225000049, 1517.057265928030120, 205.0766634521770015 ) ) ;
#46732=CARTESIAN_POINT ( 'NONE',  ( 8.302022980286720255, 1511.419866572826550, 204.7917934253724184 ) ) ;
#46746=FACE_OUTER_BOUND ( 'NONE', #29895, .T. ) ;
#46750=CARTESIAN_POINT ( 'NONE',  ( 5.003848121975000396, 1517.005755693489846, 201.7875176594370146 ) ) ;
#46754=CARTESIAN_POINT ( 'NONE',  ( 7.615555629554999761, 1511.534866634170157, 206.2833989651869899 ) ) ;
#46765=CARTESIAN_POINT ( 'NONE',  ( -8.213194891504999262, 1511.437978678640093, 213.1815177657570075 ) ) ;
#46775=CARTESIAN_POINT ( 'NONE',  ( -15.24750712096500038, 1514.857962383129916, 223.5728236591669997 ) ) ;
#46780=EDGE_CURVE ( 'NONE', #10547, #31839, #107198, .T. ) ;
#46786=CARTESIAN_POINT ( 'NONE',  ( -7.326795561505000443, 1516.760434454289907, 214.9020780475669881 ) ) ;
#46794=CARTESIAN_POINT ( 'NONE',  ( -1.133517003235000153, 1516.713079096360161, 204.5117660986770147 ) ) ;
#46800=CARTESIAN_POINT ( 'NONE',  ( -2.344512155952720001, 1516.526058380829909, 201.4130301786289863 ) ) ;
#46806=CARTESIAN_POINT ( 'NONE',  ( -4.028630622785000170, 1516.812923327049930, 212.5819478221170016 ) ) ;
#46811=CARTESIAN_POINT ( 'NONE',  ( -7.709431855391500221, 1516.549587951120202, 211.8473045898290081 ) ) ;
#46812=CARTESIAN_POINT ( 'NONE',  ( 1.133653140995000141, 1516.978425811520083, 209.8592968530090275 ) ) ;
#46820=CARTESIAN_POINT ( 'NONE',  ( -15.01814846036320006, 1514.214451730469818, 194.3960741685959874 ) ) ;
#46826=CARTESIAN_POINT ( 'NONE',  ( -0.7396922758749979732, 1517.135701590510052, 216.4591432822169850 ) ) ;
#46831=CARTESIAN_POINT ( 'NONE',  ( 0.7396922377450010355, 1517.135701590510052, 201.7845486201169933 ) ) ;
#46855=CARTESIAN_POINT ( 'NONE',  ( -1.906495983305939756E-08, 1508.551704408389924, 214.1089243866270238 ) ) ;
#46864=CARTESIAN_POINT ( 'NONE',  ( -0.3328841718826340279, 1516.837731796779963, 201.4048689279690052 ) ) ;
#46869=CARTESIAN_POINT ( 'NONE',  ( 13.18795884192349988, 1512.495155157800127, 224.3903603686180190 ) ) ;
#46870=ORIENTED_EDGE ( 'NONE', *, *, #62690, .T. ) ;
#46911=ORIENTED_EDGE ( 'NONE', *, *, #72735, .F. ) ;
#46912=VERTEX_POINT ( 'NONE', #94268 ) ;
#46913=CARTESIAN_POINT ( 'NONE',  ( 3.463767257884999839, 1517.014196759610059, 210.8246003415769962 ) ) ;
#46916=PLANE ( 'NONE',  #60542 ) ;
#46922=CARTESIAN_POINT ( 'NONE',  ( -5.005071046424999892, 1516.710692850270107, 201.7963041449669959 ) ) ;
#46937=CARTESIAN_POINT ( 'NONE',  ( 2.881325373965000214, 1517.003078582959688, 210.2407492406470055 ) ) ;
#46942=CARTESIAN_POINT ( 'NONE',  ( 7.558229865324999963, 1510.775363762149937, 205.2680898081869998 ) ) ;
#46943=CARTESIAN_POINT ( 'NONE',  ( -6.950833568235000648, 1517.156142772249950, 206.6378959915070084 ) ) ;
#46946=CARTESIAN_POINT ( 'NONE',  ( 0.08509230700728949437, 1516.966051576903965, 201.6138908561003973 ) ) ;
#46959=CARTESIAN_POINT ( 'NONE',  ( 7.720650135305000994, 1516.977993847330026, 214.9014730243169993 ) ) ;
#46961=CARTESIAN_POINT ( 'NONE',  ( 7.709377398217750255, 1516.547505386119838, 206.4302690467380046 ) ) ;
#47022=FACE_OUTER_BOUND ( 'NONE', #74160, .T. ) ;
#47025=CARTESIAN_POINT ( 'NONE',  ( -4.625790014595000166, 1517.104192383289956, 208.0004623403669939 ) ) ;
#47046=CARTESIAN_POINT ( 'NONE',  ( 13.41829267866989106, 1513.652806704122668, 225.8959966016125236 ) ) ;
#47059=CARTESIAN_POINT ( 'NONE',  ( -3.487586626270560153, 1508.731366866819826, 204.5668911269270041 ) ) ;
#47061=CARTESIAN_POINT ( 'NONE',  ( -3.458526536014999930, 1516.742629295279812, 204.1242721449069961 ) ) ;
#47082=CARTESIAN_POINT ( 'NONE',  ( -6.775684858734999594, 1512.341575225259930, 201.7407336143970156 ) ) ;
#47095=CARTESIAN_POINT ( 'NONE',  ( 12.53415176833500055, 1512.123798513659949, 225.3767377372669785 ) ) ;
#47102=CARTESIAN_POINT ( 'NONE',  ( -3.269984819434999856, 1516.999105586269934, 207.4194399470370058 ) ) ;
#47120=EDGE_LOOP ( 'NONE', ( #2018, #66005, #73862, #87689 ) ) ;
#47144=EDGE_CURVE ( 'NONE', #71879, #14033, #28474, .T. ) ;
#47146=DIRECTION ( 'NONE',  ( 0.7384854939282339270, 1.641580738839949676E-15, -0.6742693640212139572 ) ) ;
#47156=CARTESIAN_POINT ( 'NONE',  ( -5.785582951674999919, 1516.981965530290154, 205.0894480302270040 ) ) ;
#47170=CARTESIAN_POINT ( 'NONE',  ( 2.493697040924999886, 1516.977201124959947, 210.2401991861970032 ) ) ;
#47184=CARTESIAN_POINT ( 'NONE',  ( -6.910053069894999567, 1514.330398624150121, 217.1607477560669679 ) ) ;
#47185=CARTESIAN_POINT ( 'NONE',  ( 16.78435730151638694, 1513.560745841035896, 195.8810728685500635 ) ) ;
#47197=CARTESIAN_POINT ( 'NONE',  ( 4.608146781254999880, 1516.677239312369920, 206.8257210811669893 ) ) ;
#47208=CARTESIAN_POINT ( 'NONE',  ( -5.689538399873499408, 1510.689985724140115, 201.5635966250480067 ) ) ;
#47210=CARTESIAN_POINT ( 'NONE',  ( -5.726916886920052185, 1510.539524115660697, 201.5773753062340461 ) ) ;
#47214=CARTESIAN_POINT ( 'NONE',  ( -2.870951705914999597, 1517.111322026010157, 215.6844817927369888 ) ) ;
#47217=CARTESIAN_POINT ( 'NONE',  ( 2.491619553449157642, 1516.536652113955824, 216.8309391655190836 ) ) ;
#47218=CARTESIAN_POINT ( 'NONE',  ( 2.298048923505000118, 1516.764084769670262, 212.5672535042169784 ) ) ;
#47228=EDGE_CURVE ( 'NONE', #19916, #94671, #81794, .T. ) ;
#47236=CARTESIAN_POINT ( 'NONE',  ( 4.609996581545000360, 1516.769879638719885, 205.6626893540170329 ) ) ;
#47264=CARTESIAN_POINT ( 'NONE',  ( 7.976333483275767300, 1511.738168994444095, 205.8271000182464832 ) ) ;
#47274=CARTESIAN_POINT ( 'NONE',  ( -10.96015512746500065, 1512.830284628050094, 193.2119433744669834 ) ) ;
#47277=CARTESIAN_POINT ( 'NONE',  ( -7.718134667564999774, 1516.881930554049859, 201.7919159189069944 ) ) ;
#47285=VERTEX_POINT ( 'NONE', #45963 ) ;
#47292=CARTESIAN_POINT ( 'NONE',  ( -7.589847775084999526, 1511.982868782460173, 211.5342623288869959 ) ) ;
#47307=EDGE_CURVE ( 'NONE', #56739, #14033, #1494, .T. ) ;
#47312=CARTESIAN_POINT ( 'NONE',  ( 2.875850094215000041, 1516.647618671360078, 214.8936433964170192 ) ) ;
#47318=DIRECTION ( 'NONE',  ( -0.7044160264027579110, -0.08715574274767008689, -0.7044160264027579110 ) ) ;
#47319=CARTESIAN_POINT ( 'NONE',  ( -3.459156616214999591, 1516.769879638719885, 204.5118493505569859 ) ) ;
#47333=CARTESIAN_POINT ( 'NONE',  ( 7.723480079395000253, 1517.086065052259983, 213.1573821953169841 ) ) ;
#47338=CARTESIAN_POINT ( 'NONE',  ( -7.719696504299309758, 1516.941612417570013, 209.0971862408350148 ) ) ;
#47340=CARTESIAN_POINT ( 'NONE',  ( -4.608021707265000266, 1516.660388280709867, 210.8351633799069873 ) ) ;
#47343=CARTESIAN_POINT ( 'NONE',  ( 2.759768239755020058, 1516.551696783219995, 216.8313331240459831 ) ) ;
#47357=CARTESIAN_POINT ( 'NONE',  ( -1.124894088365000044, 1517.194816588360027, 216.0733631026070043 ) ) ;
#47362=CARTESIAN_POINT ( 'NONE',  ( -5.004442077115000664, 1516.690345681169902, 201.4087281291169802 ) ) ;
#47365=CARTESIAN_POINT ( 'NONE',  ( -15.18044686046500935, 1511.791180387469922, 220.8782529452671497 ) ) ;
#47445=CARTESIAN_POINT ( 'NONE',  ( -1.700259714084999763, 1516.898441858519845, 210.8400494336869997 ) ) ;
#47448=CARTESIAN_POINT ( 'NONE',  ( -2.283570671295000132, 1516.909589401870107, 212.0033943946770023 ) ) ;
#47456=CARTESIAN_POINT ( 'NONE',  ( -4.616861546545000472, 1516.666407245520077, 201.4093549791169835 ) ) ;
#47458=FACE_OUTER_BOUND ( 'NONE', #97187, .T. ) ;
#47472=CARTESIAN_POINT ( 'NONE',  ( 1.718203463455000080, 1516.898441858519845, 210.8221056461869978 ) ) ;
#47478=CARTESIAN_POINT ( 'NONE',  ( 7.848179674985000354, 1511.193640125469983, 204.5989548728170178 ) ) ;
#47479=CARTESIAN_POINT ( 'NONE',  ( -4.043990345725000601, 1516.983612918759945, 206.6425990843970055 ) ) ;
#47482=CARTESIAN_POINT ( 'NONE',  ( -1.949295105551302365, 1516.541277319989604, 201.8775772585021286 ) ) ;
#47495=CARTESIAN_POINT ( 'NONE',  ( -5.001338666445000136, 1516.911981270829983, 214.9058546054269812 ) ) ;
#47497=CARTESIAN_POINT ( 'NONE',  ( 7.708939270935911026, 1516.530773980259937, 207.1624426174489884 ) ) ;
#47515=EDGE_CURVE ( 'NONE', #29266, #40040, #72430, .T. ) ;
#47516=CARTESIAN_POINT ( 'NONE',  ( -7.012921474261649024, 1508.551704408390151, 202.7299072940186875 ) ) ;
#47525=CARTESIAN_POINT ( 'NONE',  ( -3.780286426965000057, 1510.542924508009946, 201.5697040178069983 ) ) ;
#47554=CARTESIAN_POINT ( 'NONE',  ( -6.769661310147350619, 1509.032013615249980, 216.3879269483049939 ) ) ;
#47565=CARTESIAN_POINT ( 'NONE',  ( -4.626591905484999323, 1517.096587378560116, 207.4170511287669854 ) ) ;
#47585=CARTESIAN_POINT ( 'NONE',  ( 14.79465543570480079, 1514.566425925628209, 225.3731531939783679 ) ) ;
#47600=CARTESIAN_POINT ( 'NONE',  ( -3.487587141067280072, 1509.038630944639863, 204.6345965622120104 ) ) ;
#47602=CARTESIAN_POINT ( 'NONE',  ( -4.039897316195000698, 1516.787536375099990, 204.1233307748069876 ) ) ;
#47608=VERTEX_POINT ( 'NONE', #106025 ) ;
#47613=CARTESIAN_POINT ( 'NONE',  ( -14.42425707855669970, 1513.497693042470019, 193.9846077359950129 ) ) ;
#47633=ORIENTED_EDGE ( 'NONE', *, *, #918, .T. ) ;
#47639=CARTESIAN_POINT ( 'NONE',  ( 12.04783377103500008, 1512.799725290120023, 225.7711220359670108 ) ) ;
#47660=DIRECTION ( 'NONE',  ( 0.02616798426500965835, 0.9993150019883683122, 0.02616798426500955774 ) ) ;
#47696=CARTESIAN_POINT ( 'NONE',  ( -3.029841966249135599, 1511.989348024461833, 201.2192106154559781 ) ) ;
#47703=CARTESIAN_POINT ( 'NONE',  ( -3.461047329755000401, 1516.858765657450249, 205.6745815831370123 ) ) ;
#47717=CARTESIAN_POINT ( 'NONE',  ( 3.269984781304999810, 1516.999105586269934, 210.8242519552970009 ) ) ;
#47725=EDGE_LOOP ( 'NONE', ( #11628, #50219, #25052 ) ) ;
#47730=CARTESIAN_POINT ( 'NONE',  ( -7.248946814685000462, 1514.005261957190214, 217.0303516513569946 ) ) ;
#47743=CARTESIAN_POINT ( 'NONE',  ( 2.868112131164999745, 1516.855632454399938, 208.3641823986619954 ) ) ;
#47744=ORIENTED_EDGE ( 'NONE', *, *, #87105, .T. ) ;
#47751=DIRECTION ( 'NONE',  ( 0.000000000000000000, 1.000000000000000000, -6.123233995736769734E-17 ) ) ;
#47753=CARTESIAN_POINT ( 'NONE',  ( -5.762402200599920477, 1511.083508941950186, 201.4380933754170258 ) ) ;
#47755=CARTESIAN_POINT ( 'NONE',  ( -5.750872970432570952, 1510.549724825256135, 201.5793989082007727 ) ) ;
#47756=CYLINDRICAL_SURFACE ( 'NONE', #109008, 0.4999999999999449329 ) ;
#47760=CARTESIAN_POINT ( 'NONE',  ( -1.709384611084999950, 1517.224900789629828, 216.4615953054470197 ) ) ;
#47764=CARTESIAN_POINT ( 'NONE',  ( 2.346054097678328176, 1516.530616268062886, 216.8307811113319303 ) ) ;
#47765=CARTESIAN_POINT ( 'NONE',  ( -2.285487619494999567, 1517.001127920769704, 213.1661676502270097 ) ) ;
#47773=ADVANCED_FACE ( 'NONE', ( #107665 ), #23086, .F. ) ;
#47785=CARTESIAN_POINT ( 'NONE',  ( 5.773668814845000163, 1516.734985836460055, 205.0832084693769843 ) ) ;
#47813=CARTESIAN_POINT ( 'NONE',  ( 8.384950263960369909, 1511.400233449589450, 204.5379475627291868 ) ) ;
#47822=CARTESIAN_POINT ( 'NONE',  ( -12.15948100306500024, 1512.592133792520144, 192.4950717916669873 ) ) ;
#47826=CARTESIAN_POINT ( 'NONE',  ( -7.718763544034999313, 1516.905946377369901, 202.1794916586869988 ) ) ;
#47830=CARTESIAN_POINT ( 'NONE',  ( 15.29601658473500159, 1513.169116394660023, 194.9970914992669861 ) ) ;
#47836=ORIENTED_EDGE ( 'NONE', *, *, #101568, .T. ) ;
#47851=CARTESIAN_POINT ( 'NONE',  ( 8.788316489185000080, 1511.741868877540128, 202.8695794779170001 ) ) ;
#47862=CARTESIAN_POINT ( 'NONE',  ( -5.778372601744999670, 1516.932669162149978, 216.0673360190369863 ) ) ;
#47869=CARTESIAN_POINT ( 'NONE',  ( -7.723480117524999855, 1517.086065052259983, 205.0863097070169943 ) ) ;
#47871=CARTESIAN_POINT ( 'NONE',  ( 5.006259848694999626, 1516.939723362869927, 209.1089481433290018 ) ) ;
#47874=CARTESIAN_POINT ( 'NONE',  ( 6.772137591825000413, 1511.702066573639968, 216.3336057811770274 ) ) ;
#47883=CARTESIAN_POINT ( 'NONE',  ( 1.715361092244999996, 1516.743010792419909, 212.5670474586069929 ) ) ;
#47890=CARTESIAN_POINT ( 'NONE',  ( -7.708862459925570398, 1516.527839230000154, 211.3267386195620077 ) ) ;
#47891=CARTESIAN_POINT ( 'NONE',  ( -7.321169269124999879, 1516.531533746980131, 210.8305669548069829 ) ) ;
#47905=CARTESIAN_POINT ( 'NONE',  ( -4.034908597844999889, 1517.068717944079935, 216.4577469658269990 ) ) ;
#47911=CARTESIAN_POINT ( 'NONE',  ( -6.942973667334999988, 1516.833844030519913, 201.7931697622170191 ) ) ;
#47929=DIRECTION ( 'NONE',  ( 0.000000000000000000, 6.123233995736769734E-17, 1.000000000000000000 ) ) ;
#47948=CARTESIAN_POINT ( 'NONE',  ( 14.62991242738410058, 1513.722010161000071, 224.1519871687980014 ) ) ;
#47991=CARTESIAN_POINT ( 'NONE',  ( -4.995623491025000362, 1516.636036526019780, 210.8344906863870278 ) ) ;
#47994=CARTESIAN_POINT ( 'NONE',  ( 7.335900995594999863, 1517.068717944079935, 213.1567545299469657 ) ) ;
#48002=CARTESIAN_POINT ( 'NONE',  ( 6.553524377605000062, 1516.882690742909972, 202.1776141839370098 ) ) ;
#48018=CARTESIAN_POINT ( 'NONE',  ( 4.625789976465000564, 1517.104192383289956, 210.2432295619669844 ) ) ;
#48019=EDGE_CURVE ( 'NONE', #84553, #46912, #13080, .T. ) ;
#48024=CARTESIAN_POINT ( 'NONE',  ( 7.559010162584999470, 1510.805212328559946, 203.6254154108069940 ) ) ;
#48025=CARTESIAN_POINT ( 'NONE',  ( 1.118104729594999958, 1516.965971551240045, 206.8221779662269739 ) ) ;
#48026=ORIENTED_EDGE ( 'NONE', *, *, #84024, .F. ) ;
#48042=CARTESIAN_POINT ( 'NONE',  ( 2.873329360754999673, 1516.572193931679976, 216.4439510378570048 ) ) ;
#48044=CARTESIAN_POINT ( 'NONE',  ( 7.714747304227939750, 1516.752573823159992, 208.4886776470619907 ) ) ;
#48075=CARTESIAN_POINT ( 'NONE',  ( -5.441672406744999968, 1511.126521646420088, 201.4186169135170132 ) ) ;
#48108=( BOUNDED_CURVE ( )  B_SPLINE_CURVE ( 3, ( #82173, #106282, #5473, #107930 ),
 .UNSPECIFIED., .F., .F. ) 
 B_SPLINE_CURVE_WITH_KNOTS ( ( 4, 4 ),
 ( 1.282549416543149912, 2.438195290895380118 ),
 .UNSPECIFIED. ) 
 CURVE ( )  GEOMETRIC_REPRESENTATION_ITEM ( )  RATIONAL_B_SPLINE_CURVE ( ( 1.000000000000000000, 0.8917691661751018239, 0.8917691661751018239, 1.000000000000000000 ) ) 
 REPRESENTATION_ITEM ( '' )  );
#48121=CARTESIAN_POINT ( 'NONE',  ( 7.708745647785000266, 1516.523379810429788, 207.4137536659370085 ) ) ;
#48148=EDGE_CURVE ( 'NONE', #31839, #55731, #88352, .T. ) ;
#48163=CARTESIAN_POINT ( 'NONE',  ( 4.029572640705000985, 1516.858649670339901, 205.0803734583570019 ) ) ;
#48167=ORIENTED_EDGE ( 'NONE', *, *, #83652, .T. ) ;
#48170=CARTESIAN_POINT ( 'NONE',  ( 4.491293097786513755, 1508.884207228267314, 205.6342589212028713 ) ) ;
#48171=CARTESIAN_POINT ( 'NONE',  ( -13.08508101585309902, 1512.436270050410030, 193.8787656426380011 ) ) ;
#48249=AXIS2_PLACEMENT_3D ( 'NONE', #28385, #19414, #95036 ) ;
#48255=CARTESIAN_POINT ( 'NONE',  ( -4.936086582586449722, 1511.397679222030092, 200.6202249550506167 ) ) ;
#48263=CARTESIAN_POINT ( 'NONE',  ( 4.997573787194999895, 1516.742629295279812, 205.6633194342169872 ) ) ;
#48277=CARTESIAN_POINT ( 'NONE',  ( 0.7559394982620020187, 1516.972341476009888, 210.2438793621770117 ) ) ;
#48283=PRODUCT ( 'Cutting Blade', 'Cutting Blade', '', ( #58327 ) ) ;
#48289=EDGE_LOOP ( 'NONE', ( #32134, #86789, #15457, #85973, #95925 ) ) ;
#48291=CARTESIAN_POINT ( 'NONE',  ( -7.014484281215001005, 1513.886778334009932, 216.7648687176869942 ) ) ;
#48292=CARTESIAN_POINT ( 'NONE',  ( 16.55311983492223504, 1514.160701262335579, 194.8748343058166199 ) ) ;
#48306=CARTESIAN_POINT ( 'NONE',  ( 3.454172615424999648, 1517.122088787240045, 201.3974225380069925 ) ) ;
#48307=CARTESIAN_POINT ( 'NONE',  ( 3.253301381255000013, 1516.790374942449944, 207.9863856151469861 ) ) ;
#48318=CARTESIAN_POINT ( 'NONE',  ( -5.556441586205710159, 1511.478393686179970, 200.7426215012330033 ) ) ;
#48320=CARTESIAN_POINT ( 'NONE',  ( -6.150246140235383407, 1510.808998927847597, 201.6520066974360077 ) ) ;
#48326=B_SPLINE_SURFACE_WITH_KNOTS ( 'NONE', 5, 5, ( 
 ( #90009, #48587, #56986, #99498, #48024, #82721 ),
 ( #5460, #82161, #31757, #72683, #22781, #4904 ),
 ( #12762, #107914, #57544, #89468, #6011, #108473 ),
 ( #55336, #91667, #47478, #91117, #56429, #39620 ),
 ( #30097, #106807, #64292, #39043, #46942, #22230 ),
 ( #65393, #14393, #30663, #40164, #74346, #81061 ),
 ( #81600, #64848, #4375, #21684, #38505, #98412 ),
 ( #55890, #13286, #20402, #46754, #3102, #29362 ),
 ( #105543, #11481, #4181, #104982, #38314, #70314 ),
 ( #104428, #46203, #72493, #37231, #28272, #44533 ),
 ( #87641, #106084, #19859, #80337, #89277, #62465 ),
 ( #61907, #96587, #96025, #80885, #78678, #37783 ) ),
 .UNSPECIFIED., .F., .F., .F.,
 ( 6, 3, 3, 6 ),
 ( 6, 6 ),
 ( 3.686514310890000257, 6.076675143290000136, 7.815970586859999791, 8.927001670199999239 ),
 ( 0.000000000000000000, 1.000000000000000000 ),
 .UNSPECIFIED. ) ;
#48327=CARTESIAN_POINT ( 'NONE',  ( -6.941727290454999810, 1516.882217593000178, 216.4530290611770056 ) ) ;
#48331=CARTESIAN_POINT ( 'NONE',  ( -2.478306858074999841, 1516.938330505699923, 212.5844667883370107 ) ) ;
#48334=CARTESIAN_POINT ( 'NONE',  ( 3.487584104944840391, 1508.551704408389924, 214.1089243997540166 ) ) ;
#48343=DIRECTION ( 'NONE',  ( 0.000000000000000000, -0.02617694830788849791, -0.9996573249755569268 ) ) ;
#48349=CARTESIAN_POINT ( 'NONE',  ( 3.448206878685000198, 1516.904492006980036, 205.0794281543969646 ) ) ;
#48363=VECTOR ( 'NONE', #61506, 1000.000000000000000 ) ;
#48369=LINE ( 'NONE', #14183, #33394 ) ;
#48374=CARTESIAN_POINT ( 'NONE',  ( -3.669386717783980068, 1517.051704642929963, 215.6629163041010031 ) ) ;
#48378=CARTESIAN_POINT ( 'NONE',  ( 8.520846174749847179, 1511.399999645683920, 204.1281607283802089 ) ) ;
#48385=CARTESIAN_POINT ( 'NONE',  ( -7.458082279446967888, 1510.848430437142952, 215.3131282273689919 ) ) ;
#48393=CARTESIAN_POINT ( 'NONE',  ( -5.780861274184998955, 1516.783701990830195, 202.1826264492970324 ) ) ;
#48396=CARTESIAN_POINT ( 'NONE',  ( 15.46640438443499832, 1511.810036768419877, 197.0767216879669945 ) ) ;
#48402=VERTEX_POINT ( 'NONE', #27512 ) ;
#48421=CARTESIAN_POINT ( 'NONE',  ( 8.371228001764999149, 1512.069761553110084, 202.7380249772070044 ) ) ;
#48432=CARTESIAN_POINT ( 'NONE',  ( 0.7543881828220019292, 1516.727502608469877, 215.6727161143369926 ) ) ;
#48440=CARTESIAN_POINT ( 'NONE',  ( -2.298369507954999946, 1516.779243033999819, 205.8702346062869992 ) ) ;
#48442=CARTESIAN_POINT ( 'NONE',  ( -1.127928371535000140, 1516.989863902050047, 209.1319708558790182 ) ) ;
#48450=CARTESIAN_POINT ( 'NONE',  ( 5.513435558250590951, 1508.884207225577711, 216.6305528438562362 ) ) ;
#48456=CARTESIAN_POINT ( 'NONE',  ( -3.255340964424999761, 1516.962555622980062, 213.7459452615670159 ) ) ;
#48460=CARTESIAN_POINT ( 'NONE',  ( -7.708997972447890312, 1516.533014244449987, 211.5310356469510111 ) ) ;
#48461=CARTESIAN_POINT ( 'NONE',  ( 2.493697040924999886, 1516.977201124959947, 210.2401991861970032 ) ) ;
#48475=CARTESIAN_POINT ( 'NONE',  ( 2.873329360754999673, 1516.572193931679976, 216.4439510378570048 ) ) ;
#48480=CARTESIAN_POINT ( 'NONE',  ( -4.616861546545000472, 1516.666407245520077, 201.4093549791169835 ) ) ;
#48489=VECTOR ( 'NONE', #25579, 1000.000000000000000 ) ;
#48511=CARTESIAN_POINT ( 'NONE',  ( 2.564633783425000146, 1511.308638870219966, 216.6940388207569868 ) ) ;
#48515=CARTESIAN_POINT ( 'NONE',  ( 14.42425704043469814, 1513.497693042480023, 224.2590841663360095 ) ) ;
#48554=EDGE_LOOP ( 'NONE', ( #103419, #75006, #757, #80415 ) ) ;
#48555=CARTESIAN_POINT ( 'NONE',  ( -3.445685115514999897, 1516.778761582560037, 211.6139765934069885 ) ) ;
#48559=CARTESIAN_POINT ( 'NONE',  ( -0.7356989727169980231, 1517.020847257979995, 212.5827121409169820 ) ) ;
#48563=ORIENTED_EDGE ( 'NONE', *, *, #103887, .T. ) ;
#48565=CARTESIAN_POINT ( 'NONE',  ( -5.780861274184998955, 1516.783701990830195, 202.1826264492970324 ) ) ;
#48581=CARTESIAN_POINT ( 'NONE',  ( 3.268859396054999866, 1516.922519270759949, 211.5998327024669834 ) ) ;
#48587=CARTESIAN_POINT ( 'NONE',  ( 8.324963421445000122, 1511.468585915670019, 203.7405339563369751 ) ) ;
#48588=CARTESIAN_POINT ( 'NONE',  ( -4.044321718124999521, 1517.001127920769704, 206.8363583507369867 ) ) ;
#48590=DIRECTION ( 'NONE',  ( -2.479303797180243098E-05, 0.02617627755937491918, 0.9996573422320469415 ) ) ;
#48604=CARTESIAN_POINT ( 'NONE',  ( -7.512750246095000861, 1509.038615934239942, 214.6352815282469919 ) ) ;
#48605=CARTESIAN_POINT ( 'NONE',  ( -2.871580426725000024, 1517.129577905929864, 216.0720609035170128 ) ) ;
#48607=CARTESIAN_POINT ( 'NONE',  ( 7.710157425188729263, 1516.577293414350152, 207.6821489692630109 ) ) ;
#48633=DIRECTION ( 'NONE',  ( 0.02616798426500965835, 0.9993150019883683122, -0.02616798426500970692 ) ) ;
#48652=ADVANCED_FACE ( 'NONE', ( #12906 ), #48743, .T. ) ;
#48673=CARTESIAN_POINT ( 'NONE',  ( 3.052975896485000007, 1516.551704408390151, 217.1245693350269903 ) ) ;
#48683=CARTESIAN_POINT ( 'NONE',  ( -3.269025173884999802, 1517.026534522949987, 208.0024068424170025 ) ) ;
#48718=CARTESIAN_POINT ( 'NONE',  ( -1.134358008724999811, 1516.744381837270112, 205.0932347109869909 ) ) ;
#48721=CARTESIAN_POINT ( 'NONE',  ( 14.97619053132000033, 1512.179780174510142, 196.6274074352839989 ) ) ;
#48723=EDGE_LOOP ( 'NONE', ( #73026, #74928, #81565, #38097 ) ) ;
#48727=CARTESIAN_POINT ( 'NONE',  ( -12.85932415441300058, 1512.319979277499897, 193.9537317410139963 ) ) ;
#48743=CYLINDRICAL_SURFACE ( 'NONE', #8703, 2.000000000000007550 ) ;
#48760=CARTESIAN_POINT ( 'NONE',  ( 12.18971934853500194, 1512.123542805230272, 223.8476153537669973 ) ) ;
#48819=CARTESIAN_POINT ( 'NONE',  ( 5.772727908745000747, 1516.691414181030041, 205.6645793267070133 ) ) ;
#48834=CARTESIAN_POINT ( 'NONE',  ( 2.299667965875000331, 1516.965971551240045, 210.2399506998270056 ) ) ;
#48863=CARTESIAN_POINT ( 'NONE',  ( -3.260378293205000055, 1516.582197289609894, 201.4115600944169842 ) ) ;
#48864=CARTESIAN_POINT ( 'NONE',  ( -0.007128875282218469743, 1517.006509894990131, 208.3750284165899984 ) ) ;
#48883=CARTESIAN_POINT ( 'NONE',  ( -1.125509888415000104, 1517.203017563489766, 216.4609531728469847 ) ) ;
#48884=ORIENTED_EDGE ( 'NONE', *, *, #7006, .T. ) ;
#48888=CARTESIAN_POINT ( 'NONE',  ( -6.935457963315000640, 1516.627618683580067, 212.5772239474869991 ) ) ;
#48891=CARTESIAN_POINT ( 'NONE',  ( 4.369720457535109404, 1508.879003890470131, 213.2412450826520001 ) ) ;
#48907=CARTESIAN_POINT ( 'NONE',  ( -1.135185082175000026, 1516.778853242349896, 205.6747174714770097 ) ) ;
#48935=CARTESIAN_POINT ( 'NONE',  ( 8.652776089875690246, 1511.435001055579960, 203.7363227723449768 ) ) ;
#48949=CARTESIAN_POINT ( 'NONE',  ( -2.486474780875000512, 1516.560253536979872, 202.1879665292270261 ) ) ;
#48952=CARTESIAN_POINT ( 'NONE',  ( 15.84317032663500058, 1513.136578080079744, 194.8016171615669805 ) ) ;
#48965=CARTESIAN_POINT ( 'NONE',  ( -7.629870583244999338, 1512.332007210709889, 211.6709574174969930 ) ) ;
#48976=CARTESIAN_POINT ( 'NONE',  ( 7.660003937574999533, 1511.444830760690138, 203.0229484186070010 ) ) ;
#48984=CARTESIAN_POINT ( 'NONE',  ( -2.483322492024999661, 1517.139039350860003, 215.6851008610869940 ) ) ;
#48991=CARTESIAN_POINT ( 'NONE',  ( 2.284526458645000258, 1516.956048353049937, 205.6588971355569981 ) ) ;
#48993=CARTESIAN_POINT ( 'NONE',  ( 6.949703334655000120, 1517.130100026000036, 209.8609679372960102 ) ) ;
#48996=CARTESIAN_POINT ( 'NONE',  ( 6.169347524795000481, 1511.326779185850000, 216.6603264655069836 ) ) ;
#48997=B_SPLINE_CURVE_WITH_KNOTS ( 'NONE', 3,
 ( #32543, #30326, #64515, #5127, #75112, #24109, #6226, #40381, #47696, #58301, #99721, #100822, #21898, #22449, #92423, #74558, #13508, #4591, #38724, #81824, #72899, #107589, #31983, #107039, #82398, #108691, #90783, #66173, #39839, #23014, #100293, #23574, #39283, #74002, #57767, #108134, #31427, #73458, #91886, #30875, #65054, #56650, #48255, #15159, #6770, #40934, #109259, #17914, #607 ),
 .UNSPECIFIED., .F., .F.,
 ( 4, 2, 1, 2, 2, 2, 1, 1, 2, 2, 2, 2, 1, 1, 1, 2, 2, 2, 2, 1, 1, 1, 2, 2, 2, 1, 1, 2, 2, 4 ),
 ( 0.000000000000000000, 0.06249999999932660810, 0.09374999999899018277, 0.1093749999988207072, 0.1249999999986512178, 0.1874999999982259469, 0.2187499999980131726, 0.2343749999978273768, 0.2421874999977315923, 0.2499999999976357801, 0.3749999999976260656, 0.4374999999976176834, 0.4687499999975849874, 0.4843749999975918707, 0.4921874999975986431, 0.4960937499975791587, 0.4999999999975597298, 0.6249999999982577270, 0.6874999999986254329, 0.7187499999988058441, 0.7343749999988899990, 0.7421874999989331867, 0.7460937499989542809, 0.7499999999989752641, 0.8124999999992322808, 0.8437499999993610666, 0.8593749999994289013, 0.8671874999994627631, 0.8749999999994966249, 1.000000000000000000 ),
 .UNSPECIFIED. ) ;
#49005=CARTESIAN_POINT ( 'NONE',  ( -2.867803664234999772, 1516.994127245590107, 213.7465828294170080 ) ) ;
#49009=CARTESIAN_POINT ( 'NONE',  ( -7.709324863577120546, 1516.545501335879862, 211.7787317697519995 ) ) ;
#49010=CARTESIAN_POINT ( 'NONE',  ( 6.564578685215000320, 1517.199196846569976, 210.8299485595169926 ) ) ;
#49017=EDGE_CURVE ( 'NONE', #80871, #37685, #78177, .T. ) ;
#49026=CARTESIAN_POINT ( 'NONE',  ( -2.290256301855000398, 1517.170721208160103, 216.0730210990169837 ) ) ;
#49027=DIRECTION ( 'NONE',  ( 3.531714064933559186E-16, 1.000000000000000000, 0.000000000000000000 ) ) ;
#49031=CARTESIAN_POINT ( 'NONE',  ( 3.452289182574999948, 1517.069378699710114, 202.5601595088670024 ) ) ;
#49032=CARTESIAN_POINT ( 'NONE',  ( -16.30040994386499875, 1513.841826332629807, 223.7820414851669852 ) ) ;
#49096=DIRECTION ( 'NONE',  ( -0.001614263105659359630, 0.06164622090537578980, 0.9980967576356069015 ) ) ;
#49105=CARTESIAN_POINT ( 'NONE',  ( 0.7578857918350010436, 1516.872851364150165, 211.6022732247369902 ) ) ;
#49108=CARTESIAN_POINT ( 'NONE',  ( -2.865588722415000067, 1516.890356958860139, 212.3900816908670208 ) ) ;
#49116=CARTESIAN_POINT ( 'NONE',  ( 4.034280915654999689, 1517.049325831759916, 202.1735242262370207 ) ) ;
#49129=CARTESIAN_POINT ( 'NONE',  ( -3.958634283238929630, 1508.551704408389924, 204.1347675023280033 ) ) ;
#49132=CARTESIAN_POINT ( 'NONE',  ( -4.995726007844999650, 1516.651306816259876, 211.4173314712770093 ) ) ;
#49137=CARTESIAN_POINT ( 'NONE',  ( -5.013274999515000552, 1517.068517094990057, 206.8347616620369820 ) ) ;
#49155=CARTESIAN_POINT ( 'NONE',  ( 6.943602653455000606, 1516.858069504249897, 216.0629462479770098 ) ) ;
#49157=CARTESIAN_POINT ( 'NONE',  ( 7.714865528678569895, 1516.757088632780096, 208.5051077213929887 ) ) ;
#49167=DIRECTION ( 'NONE',  ( -0.02616798426398481495, -0.9993150019883594304, -0.02616798426637241201 ) ) ;
#49168=EDGE_CURVE ( 'NONE', #103079, #68646, #82184, .T. ) ;
#49175=CARTESIAN_POINT ( 'NONE',  ( -4.626591905484999323, 1517.096587378560116, 207.4170511287669854 ) ) ;
#49187=CARTESIAN_POINT ( 'NONE',  ( -5.160317838924999734, 1510.729589429620091, 201.5648160248170200 ) ) ;
#49201=DIRECTION ( 'NONE',  ( -0.6742693640212151784, 0.000000000000000000, -0.7384854939282328168 ) ) ;
#49230=CARTESIAN_POINT ( 'NONE',  ( -5.786847777804999815, 1517.104497701820037, 208.3841784293060186 ) ) ;
#49263=CARTESIAN_POINT ( 'NONE',  ( -4.159841847218469724, 1508.728286212990042, 204.6953463774560191 ) ) ;
#49265=CARTESIAN_POINT ( 'NONE',  ( 6.935457925184999262, 1516.627618683580067, 205.6664679548470076 ) ) ;
#49268=CARTESIAN_POINT ( 'NONE',  ( 15.21580400995989812, 1513.293387711960122, 194.9022240235440222 ) ) ;
#49273=CARTESIAN_POINT ( 'NONE',  ( -14.08695220650660218, 1513.170547668159998, 193.8693523408769863 ) ) ;
#49354=CARTESIAN_POINT ( 'NONE',  ( -5.786837717054999608, 1517.040132827679827, 205.8646253294070050 ) ) ;
#49363=CARTESIAN_POINT ( 'NONE',  ( -16.23489791427282114, 1514.585431660245149, 223.9400827068218689 ) ) ;
#49369=CARTESIAN_POINT ( 'NONE',  ( 1.135898785685000023, 1516.958737650239982, 210.2414381519470226 ) ) ;
#49382=EDGE_LOOP ( 'NONE', ( #89541, #57370, #92576, #30807, #42404 ) ) ;
#49391=CARTESIAN_POINT ( 'NONE',  ( -3.487587049029018171, 1508.884207228266860, 204.6305528343158642 ) ) ;
#49400=CARTESIAN_POINT ( 'NONE',  ( 5.003848121975000396, 1517.005755693489846, 201.7875176594370146 ) ) ;
#49401=CARTESIAN_POINT ( 'NONE',  ( -7.339107240745000205, 1517.203017563489766, 207.9963360818169917 ) ) ;
#49416=CARTESIAN_POINT ( 'NONE',  ( -5.980914397353036094, 1510.675349062206351, 201.6120256252374645 ) ) ;
#49417=DIRECTION ( 'NONE',  ( -0.4770263929449307105, 0.7067418228238977473, -0.5224574779879248565 ) ) ;
#49427=DIRECTION ( 'NONE',  ( -0.9996573249755569268, -0.02617694830788839730, 1.602875797835060096E-18 ) ) ;
#49429=CARTESIAN_POINT ( 'NONE',  ( 4.623787969365000805, 1516.947419719950176, 212.5709951659769956 ) ) ;
#49432=CARTESIAN_POINT ( 'NONE',  ( 4.426491198842340324, 1508.728286123109910, 213.2817096034670215 ) ) ;
#49446=CARTESIAN_POINT ( 'NONE',  ( -6.561995998525000040, 1517.083030555940013, 205.8633713531569924 ) ) ;
#49456=DIRECTION ( 'NONE',  ( 0.000000000000000000, -1.000000000000000000, 6.123233995736769734E-17 ) ) ;
#49465=CARTESIAN_POINT ( 'NONE',  ( 4.329791490734999471, 1515.051704408389924, 205.7917117663369879 ) ) ;
#49469=CARTESIAN_POINT ( 'NONE',  ( -12.05354680877381490, 1513.055463255244376, 192.5148414102740446 ) ) ;
#49473=CARTESIAN_POINT ( 'NONE',  ( -4.590060415194109567, 1517.051704403100075, 216.8444262830430205 ) ) ;
#49494=CARTESIAN_POINT ( 'NONE',  ( 3.259101798884999734, 1517.102359858469754, 202.1722709844570147 ) ) ;
#49497=CARTESIAN_POINT ( 'NONE',  ( 16.53923913363500020, 1512.406775501100128, 196.8368690890669939 ) ) ;
#49508=VERTEX_POINT ( 'NONE', #63640 ) ;
#49512=CARTESIAN_POINT ( 'NONE',  ( -7.585404424514999633, 1511.813148765560072, 211.5972449069469974 ) ) ;
#49523=FACE_OUTER_BOUND ( 'NONE', #18857, .T. ) ;
#49527=EDGE_LOOP ( 'NONE', ( #22767, #62981, #95794, #18984 ) ) ;
#49532=CARTESIAN_POINT ( 'NONE',  ( 2.486474742745000022, 1516.560253536979872, 216.0557253731069807 ) ) ;
#49534=ADVANCED_FACE ( 'NONE', ( #82619 ), #84963, .T. ) ;
#49540=CARTESIAN_POINT ( 'NONE',  ( -1.715361130375000043, 1516.743010792419909, 205.6766444437269854 ) ) ;
#49542=CARTESIAN_POINT ( 'NONE',  ( 6.562094069294999166, 1517.122674412569950, 209.8604508749069737 ) ) ;
#49554=CARTESIAN_POINT ( 'NONE',  ( 4.621267883935000320, 1516.830644417779922, 214.1213023606370029 ) ) ;
#49558=CARTESIAN_POINT ( 'NONE',  ( -7.719818767491180900, 1516.946282269519997, 209.0807804088159969 ) ) ;
#49559=CARTESIAN_POINT ( 'NONE',  ( 2.494757998004999866, 1516.937508036699910, 210.8228737931069929 ) ) ;
#49564=ORIENTED_EDGE ( 'NONE', *, *, #23393, .F. ) ;
#49568=AXIS2_PLACEMENT_3D ( 'NONE', #40734, #80122, #75465 ) ;
#49578=CARTESIAN_POINT ( 'NONE',  ( -5.780861274184998955, 1516.783701990830195, 202.1826264492970324 ) ) ;
#49609=CARTESIAN_POINT ( 'NONE',  ( 3.780286388835000011, 1510.542924508009946, 216.6739878845270084 ) ) ;
#49654=CARTESIAN_POINT ( 'NONE',  ( -2.864326125434999870, 1516.826109302209943, 211.6149197999869784 ) ) ;
#49658=CARTESIAN_POINT ( 'NONE',  ( 3.266349474065000091, 1516.797038924770050, 213.1501537103870021 ) ) ;
#49664=VERTEX_POINT ( 'NONE', #96953 ) ;
#49667=CARTESIAN_POINT ( 'NONE',  ( -4.618119704395000191, 1516.706638732659940, 202.1845071865270143 ) ) ;
#49668=DIRECTION ( 'NONE',  ( -0.01484500364079610613, 0.5669078173018522460, 0.8236474686107853049 ) ) ;
#49681=AXIS2_PLACEMENT_3D ( 'NONE', #18792, #72014, #79286 ) ;
#49683=CARTESIAN_POINT ( 'NONE',  ( -7.708770045145000083, 1516.524310051880093, 211.4128934593470035 ) ) ;
#49687=CARTESIAN_POINT ( 'NONE',  ( 6.933587655514999781, 1516.542957540330008, 207.4124872689769745 ) ) ;
#49698=LINE ( 'NONE', #14953, #88862 ) ;
#49703=CARTESIAN_POINT ( 'NONE',  ( -4.612507312034999529, 1516.886345593249871, 214.1313240375470173 ) ) ;
#49705=PLANE ( 'NONE',  #49568 ) ;
#49706=CARTESIAN_POINT ( 'NONE',  ( 6.942973629204999497, 1516.833844030519913, 216.4505221401170161 ) ) ;
#49778=CARTESIAN_POINT ( 'NONE',  ( 1.709766494024999917, 1516.959716008189844, 209.1091877442879934 ) ) ;
#49808=CIRCLE ( 'NONE', #101566, 0.9999999999999972244 ) ;
#49817=CARTESIAN_POINT ( 'NONE',  ( -2.490245952555000031, 1516.691389976299888, 204.5134284255869943 ) ) ;
#49821=CARTESIAN_POINT ( 'NONE',  ( 15.19269320784599842, 1513.356256558030054, 194.8382808670130260 ) ) ;
#49881=CARTESIAN_POINT ( 'NONE',  ( 17.15254153798861481, 1516.660421270691131, 195.1616943382034322 ) ) ;
#49906=CARTESIAN_POINT ( 'NONE',  ( -7.337153806245000354, 1517.119374999550018, 205.8621166342670108 ) ) ;
#49916=CARTESIAN_POINT ( 'NONE',  ( -16.30010424779411338, 1514.508970279820687, 223.8444557749070327 ) ) ;
#49920=CARTESIAN_POINT ( 'NONE',  ( 4.625359524845000792, 1517.025470194390209, 211.6020329869469947 ) ) ;
#49925=CARTESIAN_POINT ( 'NONE',  ( -15.15808450826500042, 1514.857962383129916, 193.1672320681669817 ) ) ;
#49940=CARTESIAN_POINT ( 'NONE',  ( 3.254300166275531314, 1516.622698719816071, 215.8883720907380450 ) ) ;
#49945=CARTESIAN_POINT ( 'NONE',  ( 7.328676169885000036, 1516.833844030519913, 202.1788723028969912 ) ) ;
#49946=CARTESIAN_POINT ( 'NONE',  ( 5.000329995535000016, 1516.770163853809890, 208.3657552043160024 ) ) ;
#49965=CARTESIAN_POINT ( 'NONE',  ( 5.779603100124999671, 1516.738222552470233, 216.8362174732170047 ) ) ;
#49970=CARTESIAN_POINT ( 'NONE',  ( 1.417628642355521551, 1516.580839848236337, 216.8320962620632599 ) ) ;
#49971=CARTESIAN_POINT ( 'NONE',  ( -7.712490991114999694, 1516.666407245520077, 213.7387074786470009 ) ) ;
#49974=CARTESIAN_POINT ( 'NONE',  ( 4.668116770205860355, 1508.551704407329908, 213.4552354802430045 ) ) ;
#49989=CARTESIAN_POINT ( 'NONE',  ( -4.042729840925000317, 1516.919782530640077, 205.8674445284970034 ) ) ;
#50024=ADVANCED_FACE ( 'NONE', ( #61569 ), #3331, .T. ) ;
#50032=CARTESIAN_POINT ( 'NONE',  ( -7.542447059886042027, 1510.549724835355164, 214.8727189264162121 ) ) ;
#50036=CARTESIAN_POINT ( 'NONE',  ( -15.37680651676500077, 1514.414736986979960, 193.7541704988670119 ) ) ;
#50044=CARTESIAN_POINT ( 'NONE',  ( 1.124289655455000148, 1517.184063036290127, 202.5579304082170040 ) ) ;
#50047=CARTESIAN_POINT ( 'NONE',  ( 16.74824990173500083, 1512.868709057579963, 195.8013333919669776 ) ) ;
#50054=ORIENTED_EDGE ( 'NONE', *, *, #56436, .F. ) ;
#50081=CARTESIAN_POINT ( 'NONE',  ( 4.036748838804999906, 1516.667393516340098, 216.0582443258770127 ) ) ;
#50082=CARTESIAN_POINT ( 'NONE',  ( -8.431984396555888495, 1511.395334939771374, 213.8483103588398819 ) ) ;
#50088=ORIENTED_EDGE ( 'NONE', *, *, #26725, .F. ) ;
#50089=CARTESIAN_POINT ( 'NONE',  ( -7.336844680545000053, 1517.106845464700200, 205.6683011064770312 ) ) ;
#50095=CARTESIAN_POINT ( 'NONE',  ( 6.760013121875000586, 1512.520476835140016, 216.7629435481970006 ) ) ;
#50102=EDGE_CURVE ( 'NONE', #74270, #33006, #69840, .T. ) ;
#50103=EDGE_CURVE ( 'NONE', #36027, #33006, #53784, .T. ) ;
#50105=CARTESIAN_POINT ( 'NONE',  ( -0.7360974767499980365, 1517.045004075700035, 213.1642344714070134 ) ) ;
#50109=CARTESIAN_POINT ( 'NONE',  ( 7.320051241770920036, 1508.610505977480216, 215.2032452850019695 ) ) ;
#50110=CARTESIAN_POINT ( 'NONE',  ( -1.701027861004999808, 1516.937508036699910, 211.6166039682370013 ) ) ;
#50126=CARTESIAN_POINT ( 'NONE',  ( 4.616861508414999093, 1516.666407245520077, 216.8343369232169948 ) ) ;
#50131=CARTESIAN_POINT ( 'NONE',  ( 3.258474578945000033, 1517.083030555940013, 202.5598499717069956 ) ) ;
#50134=CARTESIAN_POINT ( 'NONE',  ( 7.460636200844970034, 1509.035273823678153, 215.1586051060212412 ) ) ;
#50159=B_SPLINE_SURFACE_WITH_KNOTS ( 'NONE', 5, 5, ( 
 ( #22495, #87115, #10967, #88230, #70353, #2590, #36716, #65105, #48306, #99217, #82447, #69796, #90275, #11521, #10406, #3141, #78720, #104465, #70908, #45697, #105024, #75159, #15209, #48863, #7925, #109306, #33670, #7381, #100868, #24159, #109849, #93572, #25259 ),
 ( #5744, #40429, #108741, #74606, #57271, #49400, #91398, #93031, #32592, #16847, #92474, #42095, #66769, #76243, #16302, #50506, #57811, #24702, #58349, #83526, #31474, #41546, #65655, #75702, #67862, #15744, #100340, #39887, #84628, #82989, #67313, #91935, #33126 ),
 ( #51050, #49945, #23061, #23629, #14676, #110390, #74054, #101410, #101973, #6281, #58899, #59462, #32032, #108183, #66221, #99772, #6820, #40979, #84083, #94690, #18511, #52708, #26375, #17963, #19630, #70631, #655, #104749, #95795, #62226, #10136, #103074, #52158 ),
 ( #96352, #19062, #53267, #87406, #104198, #103647, #68419, #86843, #44307, #28036, #60570, #35339, #86291, #43747, #9575, #17403, #10699, #77898, #2324, #44871, #79022, #78451, #36434, #85182, #51599, #1205, #69527, #27483, #34786, #35902, #8468, #26945, #1764 ),
 ( #42641, #76794, #111, #70085, #34233, #102521, #77353, #61672, #61134, #95248, #25813, #60011, #94132, #85732, #68973, #9031, #43203, #30228, #105864, #46518, #80096, #98539, #72811, #38635, #106402, #21807, #63870, #97985, #21252, #5036, #105302, #106943, #29143 ),
 ( #55463, #54376, #13414, #64418, #89591, #63331, #4501, #38092, #36986, #72268, #107491, #39181, #87970, #56007, #30785, #11260, #28592, #64965, #12882, #71747, #90131, #29686, #81185, #3416, #47061, #47602, #81728, #53831, #88508, #45959, #11792, #62793, #97451 ),
 ( #73355, #2865, #96908, #37545, #45422, #20719, #99079, #79564, #71180, #20178, #80652, #54914, #89040, #12328, #3967, #108039, #58213, #92896, #91792, #22359, #31334, #49817, #15611, #40846, #82842, #40290, #32983, #67725, #15068, #39748, #6133, #73911, #24568 ),
 ( #50373, #65520, #75576, #84499, #99627, #109708, #22914, #48163, #67172, #41955, #5598, #31890, #66631, #100732, #74474, #66076, #56559, #7789, #48718, #76109, #101271, #110249, #92339, #108602, #100201, #58758, #57122, #23485, #16170, #57678, #33523, #90687, #83947 ),
 ( #7247, #13975, #49265, #83392, #6689, #75019, #91248, #109169, #32455, #41408, #24016, #82300, #14528, #8883, #35202, #102396, #61536, #10002, #69389, #525, #52575, #86159, #85042, #9451, #44735, #87267, #25125, #86709, #78885, #59329, #76654, #2191, #103500 ),
 ( #43616, #77765, #95115, #36305, #10561, #101832, #110804, #68834, #102936, #26802, #16709, #1076, #34096, #50911, #35761, #8332, #68288, #93999, #93440, #25679, #18379, #18934, #60989, #42496, #94545, #44173, #78310, #59872, #17263, #51455, #1625, #95666, #60427 ),
 ( #69945, #85587, #104059, #77224, #27352, #53130, #43064, #34650, #26238, #17818, #52019, #64294, #38506, #21130, #97855, #105738, #11662, #80528, #3844, #71053, #28467, #55891, #88916, #19497, #37971, #81062, #12202, #90010, #63208, #97315, #53699, #55337, #54784 ),
 ( #54246, #46397, #36860, #96781, #88372, #4377, #81602, #72685, #106808, #30099, #89469, #72153, #87840, #106271, #29557, #13287, #45838, #20585, #79971, #29022, #3289, #2739, #98413, #63742, #21685, #47479, #4907, #12764, #70500, #104617, #46943, #11128, #27913 ),
 ( #62095, #96220, #37420, #71618, #45287, #79428, #20052, #105175, #62659, #16042, #74888, #56987, #6012, #7117, #48025, #91118, #41272, #40165, #109581, #101151, #109039, #100608, #74347, #107916, #98958, #48588, #40716, #49137, #14942, #15490, #14394, #31758, #65394 ),
 ( #83817, #6566, #49687, #58633, #5461, #65944, #82722, #58086, #99499, #23892, #75445, #108475, #83270, #39622, #32852, #92219, #32322, #100069, #67044, #23354, #22232, #57545, #92765, #24445, #73225, #50243, #84372, #107368, #13840, #39045, #66504, #91668, #30664 ),
 ( #22782, #64849, #56430, #90561, #82162, #73790, #31210, #76519, #59195, #17125, #93314, #94983, #77090, #95531, #94405, #9868, #68696, #78173, #18251, #52447, #59736, #26658, #398, #51315, #33397, #43487, #67592, #9324, #35616, #34517, #102264, #7659, #86575 ),
 ( #26096, #68156, #25544, #44035, #52999, #102801, #24990, #93855, #16576, #1484, #41816, #943, #69812, #50771, #60859, #103929, #84906, #27228, #8197, #101699, #103356, #60286, #61408, #17681, #51887, #86023, #18803, #42364, #75972, #85451, #110669, #110124, #77631 ),
 ( #33962, #35068, #8749, #69248, #42932, #70367, #71483, #29972, #72551, #10422, #37840, #64164, #44591, #61966, #98282, #20456, #105043, #89339, #105604, #3710, #36732, #88793, #28888, #63083, #87132, #10982, #79296, #45157, #27776, #96647, #96080, #63620, #45712 ),
 ( #2607, #78736, #87702, #80396, #4241, #97182, #2051, #79849, #72027, #54665, #19355, #70927, #53556, #12075, #46812, #3160, #36184, #28332, #106142, #29421, #46268, #62524, #19915, #97736, #21559, #37292, #104483, #54116, #88244, #12635, #11537, #21007, #38375 ),
 ( #55210, #80942, #106681, #13704, #41135, #74217, #4772, #65807, #66371, #108346, #75315, #48461, #82599, #38918, #40586, #40035, #109458, #81468, #39491, #31628, #22097, #82027, #73662, #100490, #66917, #23771, #57958, #92091, #74758, #99926, #73099, #23220, #91546 ),
 ( #65261, #57420, #14823, #49010, #32187, #107794, #5889, #5331, #15369, #108895, #101026, #49559, #83687, #6983, #32737, #83146, #107238, #6441, #55769, #89884, #31078, #13154, #99372, #14270, #22645, #98837, #47340, #30529, #64721, #56296, #90426, #47891, #56850 ),
 ( #90982, #34396, #86452, #75851, #9204, #110548, #101573, #92637, #25968, #78051, #58507, #26540, #18131, #51764, #15910, #43908, #16454, #60167, #59606, #42801, #76395, #41692, #84236, #110001, #84781, #94856, #68025, #94285, #8626, #76961, #17563, #1358, #35500 ),
 ( #59063, #50650, #93186, #33278, #33835, #67468, #814, #93722, #69692, #270, #60735, #85329, #52329, #34940, #69127, #102134, #43365, #16999, #25413, #50110, #85898, #7536, #77512, #9742, #51199, #8077, #24324, #103230, #24861, #42248, #68571, #102670, #37711 ),
 ( #62394, #10292, #87577, #44469, #106028, #103812, #97076, #20889, #78614, #46143, #55087, #1929, #80273, #36067, #18678, #71912, #12509, #87003, #2489, #37165, #71360, #45037, #36606, #38250, #89215, #19223, #46688, #3587, #80819, #28760, #10865, #70806, #29304 ),
 ( #63501, #104920, #97620, #4125, #62964, #54546, #28205, #61842, #52874, #96518, #105473, #3039, #79730, #27111, #79182, #19796, #53429, #61296, #11957, #88679, #45589, #95414, #20341, #70252, #104359, #27656, #95962, #53999, #88131, #11420, #29852, #74082, #15237 ),
 ( #39912, #81899, #23091, #56721, #55638, #90857, #49429, #57834, #106564, #57297, #83551, #64038, #47218, #6844, #5769, #90298, #74630, #14144, #99797, #21970, #108211, #48331, #82471, #72434, #107112, #64591, #30400, #13031, #5206, #81345, #48888, #30954, #98155 ),
 ( #21428, #72973, #65679, #100366, #31499, #89760, #65129, #91424, #14699, #4659, #98710, #38798, #83016, #32058, #99242, #56162, #13579, #6308, #40453, #108765, #47765, #39359, #66247, #73533, #22518, #107668, #23652, #91960, #44753, #41005, #35782, #70519, #58376 ),
 ( #52596, #41572, #109872, #27931, #61010, #100892, #86731, #53150, #95137, #62114, #33696, #67891, #24187, #27373, #26825, #96239, #66792, #24728, #18398, #7407, #67339, #58925, #87288, #61555, #10022, #84107, #33151, #15769, #78335, #2210, #110416, #75183, #49971 ),
 ( #104079, #16329, #1646, #10583, #101438, #109333, #75727, #69966, #93056, #36322, #78902, #95688, #18954, #76268, #50529, #44192, #104634, #84654, #7951, #19515, #53720, #92502, #87857, #32616, #42120, #103521, #3860, #37988, #105194, #106826, #106287, #107383, #36876 ),
 ( #46959, #29040, #88932, #90025, #20069, #63225, #13302, #12219, #81619, #73243, #81079, #72701, #46413, #79988, #71071, #20602, #12781, #21146, #97871, #98430, #97331, #72170, #37438, #55907, #30116, #64311, #63758, #47495, #55353, #89486, #4396, #30679, #62677 ),
 ( #88390, #79445, #38523, #64866, #45308, #4922, #39064, #21702, #2756, #98974, #3308, #22248, #80545, #29572, #54800, #28485, #96799, #54262, #71635, #56446, #11145, #11678, #45855, #105755, #83836, #67610, #110141, #33414, #65411, #57563, #91685, #23909, #5479 ),
 ( #99517, #67062, #49155, #101720, #66522, #92785, #40735, #50263, #101168, #24462, #31778, #109600, #83287, #22802, #65965, #16060, #14960, #84392, #41835, #15507, #41292, #6585, #48605, #39639, #100090, #92236, #100626, #58105, #58651, #23372, #74909, #6030, #7679 ),
 ( #32342, #75991, #49706, #7137, #75466, #25012, #31229, #32872, #109059, #57008, #48042, #90578, #13858, #82181, #73808, #107937, #91136, #14413, #82739, #40183, #74365, #108493, #77649, #417, #76538, #8217, #110690, #8769, #18822, #102822, #60877, #43505, #963 ),
 ( #95003, #35087, #69268, #59213, #93878, #51335, #17144, #33981, #68717, #68176, #35636, #17701, #36201, #103374, #61426, #9343, #53017, #69830, #103947, #34535, #78193, #51905, #26116, #84924, #18271, #42382, #52464, #87152, #86045, #42950, #93332, #27245, #102283 ) ),
 .UNSPECIFIED., .F., .F., .F.,
 ( 6, 3, 3, 3, 3, 3, 3, 3, 3, 3, 6 ),
 ( 6, 3, 3, 3, 3, 3, 3, 3, 3, 3, 6 ),
 ( 0.000000000000000000, 1.936717162300000128, 3.873434324599999812, 4.841792905749999321, 5.810151486899999718, 7.746868649199999624, 9.683585811500000418, 10.65194439270000082, 11.62030297379999944, 13.55702013610000023, 15.49373729840000102 ),
 ( 0.000000000000000000, 1.936717162300000128, 3.873434324599999812, 4.841792905749999321, 5.810151486899999718, 7.746868649199999624, 9.683585811500000418, 10.65194439270000082, 11.62030297379999944, 13.55702013610000023, 15.49373729840000102 ),
 .UNSPECIFIED. ) ;
#50160=CARTESIAN_POINT ( 'NONE',  ( -13.92686555291570194, 1517.051704405520013, 226.1812314194930025 ) ) ;
#50167=CARTESIAN_POINT ( 'NONE',  ( 2.930838039564999775, 1510.983859056260144, 216.6855341620170350 ) ) ;
#50192=ORIENTED_EDGE ( 'NONE', *, *, #51415, .T. ) ;
#50194=CARTESIAN_POINT ( 'NONE',  ( 7.548952298499977509, 1510.510563526942860, 203.4716113541371385 ) ) ;
#50214=CARTESIAN_POINT ( 'NONE',  ( 4.041472473744999405, 1516.858649670339901, 213.1514186109370144 ) ) ;
#50216=CARTESIAN_POINT ( 'NONE',  ( 7.487063056100070391, 1517.051702153270071, 209.5621714086410066 ) ) ;
#50219=ORIENTED_EDGE ( 'NONE', *, *, #13848, .F. ) ;
#50221=CARTESIAN_POINT ( 'NONE',  ( -2.292940207144999576, 1516.565291103010168, 202.5758065368070220 ) ) ;
#50222=DIRECTION ( 'NONE',  ( 0.7063774289747313251, 0.04540766091858282338, 0.7063774289747313251 ) ) ;
#50228=ORIENTED_EDGE ( 'NONE', *, *, #38568, .T. ) ;
#50234=CARTESIAN_POINT ( 'NONE',  ( -4.429742689765809871, 1508.551704408389924, 204.3196046976010223 ) ) ;
#50237=CARTESIAN_POINT ( 'NONE',  ( 2.494020282435000180, 1516.876240617270014, 211.4047611534970201 ) ) ;
#50243=CARTESIAN_POINT ( 'NONE',  ( -4.045182518055000287, 1517.057265928030120, 207.4180663268770104 ) ) ;
#50256=EDGE_CURVE ( 'NONE', #69935, #84966, #1284, .T. ) ;
#50260=CARTESIAN_POINT ( 'NONE',  ( 0.7564342142240020328, 1516.783665406140017, 213.7345173100169973 ) ) ;
#50263=CARTESIAN_POINT ( 'NONE',  ( 4.036748838804999906, 1516.667393516340098, 216.0582443258770127 ) ) ;
#50265=CARTESIAN_POINT ( 'NONE',  ( 7.719451313342379883, 1516.932212683739863, 209.1137067812010173 ) ) ;
#50301=ORIENTED_EDGE ( 'NONE', *, *, #80887, .T. ) ;
#50306=EDGE_LOOP ( 'NONE', ( #90619, #30335, #81189, #42136 ) ) ;
#50309=DIRECTION ( 'NONE',  ( -0.02616798426619638615, 0.9993150019883495494, -0.02616798426453459045 ) ) ;
#50343=CARTESIAN_POINT ( 'NONE',  ( -3.267039729984999585, 1517.012231669750008, 208.3862772893259887 ) ) ;
#50373=CARTESIAN_POINT ( 'NONE',  ( 7.711550677984999602, 1516.630499592039996, 205.0863552195469879 ) ) ;
#50376=CARTESIAN_POINT ( 'NONE',  ( 15.24308028946400029, 1512.436270050410030, 196.0367649543779862 ) ) ;
#50381=CARTESIAN_POINT ( 'NONE',  ( -14.97085961631660034, 1514.147575501539905, 194.3487857625829918 ) ) ;
#50461=CARTESIAN_POINT ( 'NONE',  ( -2.862715468142697617, 1516.551704408386058, 201.3093830337851387 ) ) ;
#50465=CARTESIAN_POINT ( 'NONE',  ( 2.284199363404999961, 1516.940296199220029, 205.8526610237369994 ) ) ;
#50474=CARTESIAN_POINT ( 'NONE',  ( -16.25130726159467542, 1514.566425925963586, 223.9165014063416379 ) ) ;
#50478=CARTESIAN_POINT ( 'NONE',  ( -3.445201526505000000, 1516.743010792419909, 210.8372070624770060 ) ) ;
#50480=VECTOR ( 'NONE', #75493, 1000.000000000000000 ) ;
#50506=CARTESIAN_POINT ( 'NONE',  ( 0.7396922377450010355, 1517.135701590510052, 201.7845486201169933 ) ) ;
#50507=CARTESIAN_POINT ( 'NONE',  ( 5.011551368014999674, 1517.080322339569875, 209.8587501411369942 ) ) ;
#50510=CARTESIAN_POINT ( 'NONE',  ( 3.836782192165181904, 1511.512562116162371, 217.2653043727980560 ) ) ;
#50528=CARTESIAN_POINT ( 'NONE',  ( 0.4290910254045180450, 1516.809856563741278, 216.8380932758135771 ) ) ;
#50529=CARTESIAN_POINT ( 'NONE',  ( 1.132949076425000090, 1516.693851263360102, 214.1195642086070166 ) ) ;
#50546=CARTESIAN_POINT ( 'NONE',  ( -0.01328397755539850039, 1516.939580991450157, 205.8601936452070049 ) ) ;
#50567=CARTESIAN_POINT ( 'NONE',  ( -15.09731539277014001, 1514.821745470009319, 193.1064629479987502 ) ) ;
#50586=CARTESIAN_POINT ( 'NONE',  ( 7.722580314274734903, 1517.051704408389924, 211.3043090471990126 ) ) ;
#50588=CARTESIAN_POINT ( 'NONE',  ( -1.710004586925000236, 1516.557392317769882, 202.5758445815369839 ) ) ;
#50614=CARTESIAN_POINT ( 'NONE',  ( 6.390054448255000352, 1513.333000339840055, 201.6257627613769614 ) ) ;
#50622=CARTESIAN_POINT ( 'NONE',  ( -3.259729335964999919, 1517.119374999550018, 216.4589997383470177 ) ) ;
#50623=CARTESIAN_POINT ( 'NONE',  ( -8.133931657293652862, 1511.520884441827775, 212.9284830860449631 ) ) ;
#50627=EDGE_CURVE ( 'NONE', #46100, #19958, #108087, .T. ) ;
#50629=ORIENTED_EDGE ( 'NONE', *, *, #89820, .F. ) ;
#50630=CARTESIAN_POINT ( 'NONE',  ( 1.118903270415000151, 1517.003078582959688, 206.2405205581369785 ) ) ;
#50637=CARTESIAN_POINT ( 'NONE',  ( 7.649034400464999273, 1514.243099272629934, 214.7715657207469917 ) ) ;
#50642=B_SPLINE_CURVE_WITH_KNOTS ( 'NONE', 3,
 ( #40663, #66445, #87079, #27724, #27177, #63031 ),
 .UNSPECIFIED., .F., .F.,
 ( 4, 2, 4 ),
 ( 0.000000000000000000, 0.5000000000000000000, 1.000000000000000000 ),
 .UNSPECIFIED. ) ;
#50646=CARTESIAN_POINT ( 'NONE',  ( 1.134357970594999987, 1516.744381837270112, 213.1504571913470159 ) ) ;
#50649=CARTESIAN_POINT ( 'NONE',  ( 6.455425405871869415, 1508.551704612109916, 215.9494989760289911 ) ) ;
#50650=CARTESIAN_POINT ( 'NONE',  ( 7.338411959395000572, 1517.170512887980067, 211.6064236274570192 ) ) ;
#50667=CARTESIAN_POINT ( 'NONE',  ( -2.487103457664999961, 1516.577434278289957, 202.5755431900869894 ) ) ;
#50686=CARTESIAN_POINT ( 'NONE',  ( -4.679794233794990710, 1508.610718263850003, 212.9834969940540077 ) ) ;
#50705=CARTESIAN_POINT ( 'NONE',  ( 7.364872175426726564, 1516.579711047741739, 207.6756468922182819 ) ) ;
#50741=CARTESIAN_POINT ( 'NONE',  ( 2.877113070465000089, 1516.697242742309982, 214.1184881303969973 ) ) ;
#50749=CARTESIAN_POINT ( 'NONE',  ( -1.709358701255000001, 1516.542957540330008, 202.1882582765869927 ) ) ;
#50766=CARTESIAN_POINT ( 'NONE',  ( 4.043990307595000111, 1516.983612918759945, 211.6010928179370012 ) ) ;
#50771=CARTESIAN_POINT ( 'NONE',  ( 1.704170714124999986, 1516.927039499179955, 208.3639196453299860 ) ) ;
#50786=ADVANCED_FACE ( 'NONE', ( #29315 ), #65691, .T. ) ;
#50789=CARTESIAN_POINT ( 'NONE',  ( -3.449777353855000062, 1516.974592746400049, 214.1332139170270068 ) ) ;
#50838=CARTESIAN_POINT ( 'NONE',  ( -15.90990259576500065, 1513.492015765619954, 220.0820010595669771 ) ) ;
#50876=CARTESIAN_POINT ( 'NONE',  ( -0.7533003905399979772, 1516.992029636990083, 208.3816250717139837 ) ) ;
#50884=CARTESIAN_POINT ( 'NONE',  ( -15.30266652055029830, 1512.633419863009976, 222.5280214136559778 ) ) ;
#50901=CARTESIAN_POINT ( 'NONE',  ( -7.649034438594999763, 1514.243099272629934, 203.4721261815869866 ) ) ;
#50906=EDGE_CURVE ( 'NONE', #29671, #89283, #102010, .T. ) ;
#50909=CARTESIAN_POINT ( 'NONE',  ( -3.958629232097630180, 1508.551704408389924, 204.1347648892599977 ) ) ;
#50911=CARTESIAN_POINT ( 'NONE',  ( 1.702405985064999960, 1516.999105586269934, 205.8518611507970206 ) ) ;
#50914=CARTESIAN_POINT ( 'NONE',  ( 15.29008551986609987, 1513.004579589629884, 195.2250800361269967 ) ) ;
#50920=CARTESIAN_POINT ( 'NONE',  ( -13.62888597016050163, 1517.051704413129983, 226.2994540733420195 ) ) ;
#50945=DIRECTION ( 'NONE',  ( -0.7071067811865475727, 0.000000000000000000, 0.7071067811865475727 ) ) ;
#50955=PLANE ( 'NONE',  #28136 ) ;
#50964=CARTESIAN_POINT ( 'NONE',  ( 0.7568986996720019622, 1516.805675336850072, 213.1530147380969993 ) ) ;
#51001=CARTESIAN_POINT ( 'NONE',  ( -7.012921688925192854, 1508.551704408389696, 215.5137845987784146 ) ) ;
#51006=CARTESIAN_POINT ( 'NONE',  ( 0.7353365397730019515, 1516.995911393979895, 206.2425275143270085 ) ) ;
#51014=CARTESIAN_POINT ( 'NONE',  ( -16.25466705341527529, 1514.562529184129517, 223.9116621936409217 ) ) ;
#51019=CARTESIAN_POINT ( 'NONE',  ( 7.338753830235000386, 1517.184383877180153, 211.4127322367170052 ) ) ;
#51027=ORIENTED_EDGE ( 'NONE', *, *, #6667, .F. ) ;
#51037=LINE ( 'NONE', #60001, #22315 ) ;
#51050=CARTESIAN_POINT ( 'NONE',  ( 7.716252052974999387, 1516.810037859429940, 202.1795012402670011 ) ) ;
#51051=CARTESIAN_POINT ( 'NONE',  ( 2.292217010694999946, 1516.941178807709775, 209.1086494233340147 ) ) ;
#51067=CARTESIAN_POINT ( 'NONE',  ( -7.012921583605000286, 1509.051704408389924, 209.1218459511669892 ) ) ;
#51081=CARTESIAN_POINT ( 'NONE',  ( 4.802232110086869454, 1508.551704408389924, 213.5516190689590132 ) ) ;
#51095=ORIENTED_EDGE ( 'NONE', *, *, #50256, .T. ) ;
#51096=CARTESIAN_POINT ( 'NONE',  ( 2.865588684285000021, 1516.890356958860139, 205.8536102114670143 ) ) ;
#51117=CARTESIAN_POINT ( 'NONE',  ( -7.359379718520192348, 1516.577810474467015, 210.5819051629668195 ) ) ;
#51118=CARTESIAN_POINT ( 'NONE',  ( -13.95544062720738054, 1513.969077476929442, 192.4617105174407072 ) ) ;
#51132=FACE_OUTER_BOUND ( 'NONE', #106089, .T. ) ;
#51142=CARTESIAN_POINT ( 'NONE',  ( 6.937965660314999283, 1516.732530461250008, 204.1161457306970135 ) ) ;
#51144=CARTESIAN_POINT ( 'NONE',  ( 14.72577131403500061, 1514.214451716350140, 194.1036979393670094 ) ) ;
#51148=VERTEX_POINT ( 'NONE', #19102 ) ;
#51172=DIRECTION ( 'NONE',  ( -0.02616798426500960631, 0.9993150019883682011, 0.02616798426500960631 ) ) ;
#51173=CARTESIAN_POINT ( 'NONE',  ( 3.260378255074999565, 1516.582197289609894, 216.8321318079170226 ) ) ;
#51174=CARTESIAN_POINT ( 'NONE',  ( -8.501621014552872779, 1511.397679221962107, 214.0579325126637968 ) ) ;
#51177=CARTESIAN_POINT ( 'NONE',  ( -1.906499580428539872E-08, 1517.051704408389924, 216.8444262845069943 ) ) ;
#51180=CARTESIAN_POINT ( 'NONE',  ( -6.950214971414999887, 1517.129577905929864, 206.2502655435069983 ) ) ;
#51181=EDGE_LOOP ( 'NONE', ( #103379, #19086, #28725, #86049, #17052, #77500 ) ) ;
#51186=CARTESIAN_POINT ( 'NONE',  ( 7.496083170734999968, 1513.333000339860064, 215.5119004184770120 ) ) ;
#51194=CARTESIAN_POINT ( 'NONE',  ( -3.255967424474999650, 1516.989560013210166, 214.1335248082570217 ) ) ;
#51198=CARTESIAN_POINT ( 'NONE',  ( 5.513258753594000083, 1508.551704615640119, 216.1343122516159951 ) ) ;
#51199=CARTESIAN_POINT ( 'NONE',  ( -3.445685115514999897, 1516.778761582560037, 211.6139765934069885 ) ) ;
#51201=EDGE_CURVE ( 'NONE', #36699, #108462, #52200, .T. ) ;
#51217=CARTESIAN_POINT ( 'NONE',  ( -7.331812124104999384, 1516.906641539930206, 202.5676945058570197 ) ) ;
#51235=CARTESIAN_POINT ( 'NONE',  ( -3.487587080698910214, 1508.884219106000046, 213.6131341098150074 ) ) ;
#51273=CARTESIAN_POINT ( 'NONE',  ( 7.465999341866490724, 1510.821818219470515, 202.9578065124467230 ) ) ;
#51288=EDGE_LOOP ( 'NONE', ( #57385, #107559, #76583, #20645, #38757, #52097, #81186, #66067 ) ) ;
#51291=CARTESIAN_POINT ( 'NONE',  ( -6.936398393775000670, 1516.667393516340098, 213.1585948090369698 ) ) ;
#51296=CARTESIAN_POINT ( 'NONE',  ( -3.458526536014999930, 1516.742629295279812, 204.1242721449069961 ) ) ;
#51302=DIRECTION ( 'NONE',  ( -0.9980844203940560933, -0.06184550950400349856, -0.001619481661280090237 ) ) ;
#51310=CARTESIAN_POINT ( 'NONE',  ( -4.609064341505000328, 1516.723920667490120, 211.9995909164769898 ) ) ;
#51315=CARTESIAN_POINT ( 'NONE',  ( -3.269025173884999802, 1517.026534522949987, 208.0024068424170025 ) ) ;
#51332=CARTESIAN_POINT ( 'NONE',  ( 6.945490048805000427, 1516.932669162149978, 214.9002185338470099 ) ) ;
#51335=CARTESIAN_POINT ( 'NONE',  ( 5.004442038985000174, 1516.690345681169902, 216.8349637732169697 ) ) ;
#51407=CARTESIAN_POINT ( 'NONE',  ( -1.906563618092599921E-08, 1509.038615934239942, 213.6090957241370063 ) ) ;
#51415=EDGE_CURVE ( 'NONE', #48402, #55385, #9901, .T. ) ;
#51423=CARTESIAN_POINT ( 'NONE',  ( 6.944466742375000834, 1516.939530130779985, 209.1105810159089913 ) ) ;
#51432=CARTESIAN_POINT ( 'NONE',  ( -14.72577118585429901, 1514.214451951579804, 224.1399941292770279 ) ) ;
#51438=VERTEX_POINT ( 'NONE', #60320 ) ;
#51455=CARTESIAN_POINT ( 'NONE',  ( -6.561995998525000040, 1517.083030555940013, 205.8633713531569924 ) ) ;
#51458=CARTESIAN_POINT ( 'NONE',  ( 15.26851439840219982, 1512.495155157840145, 195.9338870901020186 ) ) ;
#51474=CARTESIAN_POINT ( 'NONE',  ( -1.906499846882070084E-08, 1516.051704408390151, 209.1218459511669892 ) ) ;
#51508=CARTESIAN_POINT ( 'NONE',  ( 3.266349474065000091, 1516.797038924770050, 213.1501537103870021 ) ) ;
#51545=CARTESIAN_POINT ( 'NONE',  ( -1.906499758064230099E-08, 1516.051704408390151, 209.1218459511669892 ) ) ;
#51554=CARTESIAN_POINT ( 'NONE',  ( -3.461360131404999763, 1516.874084700499907, 205.8683838714370040 ) ) ;
#51555=VECTOR ( 'NONE', #63266, 1000.000000000000114 ) ;
#51571=CARTESIAN_POINT ( 'NONE',  ( 7.338411959395000572, 1517.170512887980067, 211.6064236274570192 ) ) ;
#51599=CARTESIAN_POINT ( 'NONE',  ( -3.456007423304999993, 1516.647534046129977, 202.5739645571870255 ) ) ;
#51600=CARTESIAN_POINT ( 'NONE',  ( 0.7468175155120010400, 1517.006509894990131, 209.1147170949500094 ) ) ;
#51604=CARTESIAN_POINT ( 'NONE',  ( 4.330052502347664145, 1511.419866573372474, 217.4238689493611787 ) ) ;
#51611=CARTESIAN_POINT ( 'NONE',  ( -0.4382461997867930226, 1517.051704408389924, 216.6878286752280189 ) ) ;
#51637=CARTESIAN_POINT ( 'NONE',  ( -15.16677556006500005, 1513.509764667529907, 223.5894014746669995 ) ) ;
#51643=CARTESIAN_POINT ( 'NONE',  ( -2.299014068865000038, 1516.811292230880099, 206.2578025137869986 ) ) ;
#51659=ORIENTED_EDGE ( 'NONE', *, *, #15076, .F. ) ;
#51661=CARTESIAN_POINT ( 'NONE',  ( -3.432975322854999956, 1511.645462744430006, 201.1048498743170114 ) ) ;
#51664=EDGE_CURVE ( 'NONE', #33692, #81968, #41174, .T. ) ;
#51669=CARTESIAN_POINT ( 'NONE',  ( -14.24695065547103034, 1514.160659596399228, 192.5687003935095731 ) ) ;
#51694=CARTESIAN_POINT ( 'NONE',  ( 1.706797785944999868, 1517.164987839469859, 203.3324512698969784 ) ) ;
#51719=COLOUR_RGB ( '', 0.72549020, 0.75294118, 0.79215686) ;
#51724=CARTESIAN_POINT ( 'NONE',  ( 2.881222757585000238, 1516.891731298979948, 211.5992195760969707 ) ) ;
#51727=CARTESIAN_POINT ( 'NONE',  ( 8.080850430355001279, 1512.335510084610178, 202.5241399173669947 ) ) ;
#51735=CARTESIAN_POINT ( 'NONE',  ( -7.329303116114999739, 1516.857992118400034, 216.4524001036569985 ) ) ;
#51736=CARTESIAN_POINT ( 'NONE',  ( -8.147601308547534060, 1511.509050022407564, 212.9717243131179316 ) ) ;
#51743=ORIENTED_EDGE ( 'NONE', *, *, #19250, .T. ) ;
#51744=CARTESIAN_POINT ( 'NONE',  ( 4.609064303374999838, 1516.723920667490120, 206.2441009858569885 ) ) ;
#51750=CARTESIAN_POINT ( 'NONE',  ( 7.692900448525000101, 1514.487275757750012, 214.9404204251670194 ) ) ;
#51758=CIRCLE ( 'NONE', #76751, 7.500000000000000000 ) ;
#51760=CARTESIAN_POINT ( 'NONE',  ( 4.037378256055000669, 1516.688761843659904, 215.6706679112870120 ) ) ;
#51764=CARTESIAN_POINT ( 'NONE',  ( 1.717432448265000078, 1516.836638729160086, 211.4041475482669910 ) ) ;
#51778=LINE ( 'NONE', #59083, #71091 ) ;
#51780=ORIENTED_EDGE ( 'NONE', *, *, #60395, .T. ) ;
#51781=CARTESIAN_POINT ( 'NONE',  ( -1.711311266675000109, 1516.591755933730155, 203.3510257909670145 ) ) ;
#51800=CARTESIAN_POINT ( 'NONE',  ( -4.833437661688551046, 1508.551704408389924, 213.0319860769199920 ) ) ;
#51804=DIRECTION ( 'NONE',  ( 0.000000000000000000, -1.000000000000000000, 6.123233995736769734E-17 ) ) ;
#51815=B_SPLINE_CURVE_WITH_KNOTS ( 'NONE', 5,
 ( #78155, #55059, #5174, #95513, #36166, #44019, #103911, #30922, #89186, #12478, #61392, #18783 ),
 .UNSPECIFIED., .F., .F.,
 ( 6, 3, 3, 6 ),
 ( -8.927001670169998349, -7.815970586829999789, -6.076675143260000134, -3.686514310899999813 ),
 .UNSPECIFIED. ) ;
#51820=VERTEX_POINT ( 'NONE', #10322 ) ;
#51847=FACE_OUTER_BOUND ( 'NONE', #87118, .T. ) ;
#51859=CARTESIAN_POINT ( 'NONE',  ( 13.92686551478569967, 1517.051704405520013, 192.0624604828410043 ) ) ;
#51861=CARTESIAN_POINT ( 'NONE',  ( -2.285487619494999567, 1517.001127920769704, 213.1661676502270097 ) ) ;
#51866=CARTESIAN_POINT ( 'NONE',  ( -7.334328310795000583, 1517.005755693489846, 204.1179978101270081 ) ) ;
#51870=CARTESIAN_POINT ( 'NONE',  ( -3.034964906435000387, 1517.051704408389924, 217.3038049130670117 ) ) ;
#51877=VERTEX_POINT ( 'NONE', #11986 ) ;
#51883=CARTESIAN_POINT ( 'NONE',  ( -4.027697264044999947, 1516.766397346390022, 212.0005392193770035 ) ) ;
#51887=CARTESIAN_POINT ( 'NONE',  ( -3.460866208815000178, 1517.020847257979995, 208.3861469975149987 ) ) ;
#51899=CARTESIAN_POINT ( 'NONE',  ( 0.4382461657092809881, 1517.051704408389924, 201.5558633854139998 ) ) ;
#51902=CARTESIAN_POINT ( 'NONE',  ( -5.000083865865000199, 1516.858456333729919, 214.1306941701269864 ) ) ;
#51905=CARTESIAN_POINT ( 'NONE',  ( -2.485205687335000135, 1517.181921232829836, 216.8478361320569832 ) ) ;
#51910=ADVANCED_BREP_SHAPE_REPRESENTATION ( '', ( #11085, #21632 ), #78983 ) ;
#51925=ORIENTED_EDGE ( 'NONE', *, *, #51664, .T. ) ;
#51938=CARTESIAN_POINT ( 'NONE',  ( -1.633027085391620004, 1516.553531807389845, 201.4123107264900057 ) ) ;
#51953=TOROIDAL_SURFACE ( 'NONE', #55316, 6.500000000000000000, 1.000000000000000000 ) ;
#51978=VECTOR ( 'NONE', #106616, 1000.000000000000114 ) ;
#51985=CARTESIAN_POINT ( 'NONE',  ( -7.719640941135000212, 1516.939452820819952, 209.1319487995289705 ) ) ;
#52002=CARTESIAN_POINT ( 'NONE',  ( -0.7559395363919990674, 1516.972341476009888, 207.9998125401569951 ) ) ;
#52019=CARTESIAN_POINT ( 'NONE',  ( 2.864972116015000125, 1516.859514182039902, 206.2412530031170093 ) ) ;
#52071=CARTESIAN_POINT ( 'NONE',  ( 6.560742225334999844, 1517.028034847769959, 213.1554992345569701 ) ) ;
#52091=DIRECTION ( 'NONE',  ( 0.000000000000000000, -6.123233995736769734E-17, -1.000000000000000000 ) ) ;
#52097=ORIENTED_EDGE ( 'NONE', *, *, #17134, .T. ) ;
#52108=CARTESIAN_POINT ( 'NONE',  ( -4.329791528864999961, 1515.051704408389924, 205.7917117663469924 ) ) ;
#52111=CARTESIAN_POINT ( 'NONE',  ( -4.588057595808531453, 1516.952111086027799, 215.0815035125188501 ) ) ;
#52116=CARTESIAN_POINT ( 'NONE',  ( 3.445407533985000104, 1516.764084769670262, 206.8237970085970119 ) ) ;
#52130=CARTESIAN_POINT ( 'NONE',  ( -1.118104767724999782, 1516.965971551240045, 211.4215139361070044 ) ) ;
#52158=CARTESIAN_POINT ( 'NONE',  ( -7.718763544034999313, 1516.905946377369901, 202.1794916586869988 ) ) ;
#52159=CARTESIAN_POINT ( 'NONE',  ( -5.786847777804999815, 1517.104497701820037, 208.3841784293060186 ) ) ;
#52164=CARTESIAN_POINT ( 'NONE',  ( 3.059233499280463064, 1511.948749218694957, 217.0319409951804062 ) ) ;
#52166=CARTESIAN_POINT ( 'NONE',  ( 3.487592431261229642, 1509.038615938009798, 213.6090957240379851 ) ) ;
#52186=ADVANCED_FACE ( 'NONE', ( #105923 ), #4019, .F. ) ;
#52200=LINE ( 'NONE', #85773, #9154 ) ;
#52201=CARTESIAN_POINT ( 'NONE',  ( -16.42424932566499862, 1513.961173499609913, 223.7109085266669979 ) ) ;
#52206=CARTESIAN_POINT ( 'NONE',  ( 2.476733476015000157, 1516.858326417339867, 206.6281461634669938 ) ) ;
#52223=CARTESIAN_POINT ( 'NONE',  ( -2.325731141814999958, 1511.751588929339960, 201.5380540260670159 ) ) ;
#52238=FACE_OUTER_BOUND ( 'NONE', #84411, .T. ) ;
#52260=CARTESIAN_POINT ( 'NONE',  ( 2.870951667784999994, 1517.111322026010157, 202.5592101095969895 ) ) ;
#52284=CARTESIAN_POINT ( 'NONE',  ( 3.268859396054999866, 1516.922519270759949, 211.5998327024669834 ) ) ;
#52287=CARTESIAN_POINT ( 'NONE',  ( 7.072298189685000125, 1512.974587999910000, 201.9513001534670309 ) ) ;
#52295=CARTESIAN_POINT ( 'NONE',  ( 16.37694613928643150, 1512.916366990907363, 197.5610450319645679 ) ) ;
#52297=CARTESIAN_POINT ( 'NONE',  ( -4.616899872884999922, 1517.050041317280147, 216.8443827349270236 ) ) ;
#52306=CARTESIAN_POINT ( 'NONE',  ( 2.282915183265000092, 1516.876240617270014, 206.6278256496669883 ) ) ;
#52312=CARTESIAN_POINT ( 'NONE',  ( -7.012473013355389639, 1508.551704609589933, 203.6085845825829779 ) ) ;
#52317=CARTESIAN_POINT ( 'NONE',  ( -5.925858265440809625, 1511.532396045849964, 201.1754967935600007 ) ) ;
#52324=CARTESIAN_POINT ( 'NONE',  ( 6.945490048805000427, 1516.932669162149978, 214.9002185338470099 ) ) ;
#52329=CARTESIAN_POINT ( 'NONE',  ( 2.299656316094999653, 1516.843453247299749, 211.5982966343670171 ) ) ;
#52346=CARTESIAN_POINT ( 'NONE',  ( 3.255967386345000047, 1516.989560013210166, 204.1101670940770134 ) ) ;
#52387=CARTESIAN_POINT ( 'NONE',  ( 7.156843037479131198, 1516.545712885865214, 206.8754839868354907 ) ) ;
#52398=CARTESIAN_POINT ( 'NONE',  ( -5.513435596820279727, 1509.038615934079871, 216.6345961782780023 ) ) ;
#52402=CARTESIAN_POINT ( 'NONE',  ( 7.550614469730767553, 1510.484595326600129, 203.5546347261997937 ) ) ;
#52420=CARTESIAN_POINT ( 'NONE',  ( -0.7365612166329978949, 1517.066898074209803, 213.7457380308570123 ) ) ;
#52421=CARTESIAN_POINT ( 'NONE',  ( 4.461625796074999428, 1510.696675236759802, 216.6780121820170280 ) ) ;
#52426=CARTESIAN_POINT ( 'NONE',  ( -4.039897316195000698, 1516.787536375099990, 204.1233307748069876 ) ) ;
#52441=CARTESIAN_POINT ( 'NONE',  ( 3.461995158685000185, 1516.906233342200039, 211.9877574868770012 ) ) ;
#52443=EDGE_CURVE ( 'NONE', #42578, #47608, #101204, .T. ) ;
#52447=CARTESIAN_POINT ( 'NONE',  ( -1.717139122245000094, 1516.949031626070109, 208.0040058453670042 ) ) ;
#52461=CARTESIAN_POINT ( 'NONE',  ( 7.331812085974999782, 1516.906641539930206, 215.6759973964769870 ) ) ;
#52464=CARTESIAN_POINT ( 'NONE',  ( -4.616899872884999922, 1517.050041317280147, 216.8443827349270236 ) ) ;
#52465=ORIENTED_EDGE ( 'NONE', *, *, #20517, .F. ) ;
#52484=CARTESIAN_POINT ( 'NONE',  ( 5.775165528996293318, 1509.036904579127395, 201.6091405375480008 ) ) ;
#52490=CARTESIAN_POINT ( 'NONE',  ( 0.4403324358131759930, 1517.051704035390003, 201.6347831756999938 ) ) ;
#52492=CARTESIAN_POINT ( 'NONE',  ( -7.983219840484640173, 1511.369014876942174, 214.5214371862444693 ) ) ;
#52541=CARTESIAN_POINT ( 'NONE',  ( 1.135898785685000023, 1516.958737650239982, 210.2414381519470226 ) ) ;
#52550=DIRECTION ( 'NONE',  ( -0.02616798426500960631, -0.9993150019883682011, 0.02616798426500970345 ) ) ;
#52551=CARTESIAN_POINT ( 'NONE',  ( -14.81793325873010048, 1514.080593477700177, 224.0430682687909894 ) ) ;
#52558=CARTESIAN_POINT ( 'NONE',  ( -7.727327152855000492, 1517.232977404109988, 207.4118332116069894 ) ) ;
#52575=CARTESIAN_POINT ( 'NONE',  ( -2.298048961635000165, 1516.764084769670262, 205.6764383981169715 ) ) ;
#52581=ORIENTED_EDGE ( 'NONE', *, *, #83652, .F. ) ;
#52587=CARTESIAN_POINT ( 'NONE',  ( 6.616506887542479731, 1517.051706634660150, 212.8496527657779893 ) ) ;
#52596=CARTESIAN_POINT ( 'NONE',  ( 7.722536764694999611, 1517.050041317280147, 213.7387458049869906 ) ) ;
#52623=CARTESIAN_POINT ( 'NONE',  ( -7.323034312095000331, 1516.609912606490070, 212.5765947784269940 ) ) ;
#52649=CYLINDRICAL_SURFACE ( 'NONE', #39505, 0.4999999999999449329 ) ;
#52666=CARTESIAN_POINT ( 'NONE',  ( -1.717432486395000124, 1516.836638729160086, 206.8395443540670158 ) ) ;
#52675=CARTESIAN_POINT ( 'NONE',  ( 9.126915900878477927, 1516.551188146009054, 213.9333071022012120 ) ) ;
#52679=CARTESIAN_POINT ( 'NONE',  ( -1.118903308544999975, 1517.003078582959688, 212.0031713441969998 ) ) ;
#52704=CARTESIAN_POINT ( 'NONE',  ( 7.012466281385699496, 1508.551704615640119, 203.6085871785070083 ) ) ;
#52708=CARTESIAN_POINT ( 'NONE',  ( -2.486474780875000512, 1516.560253536979872, 202.1879665292270261 ) ) ;
#52709=CARTESIAN_POINT ( 'NONE',  ( -6.949703372784999722, 1517.130100026000036, 208.3827239650380250 ) ) ;
#52746=CARTESIAN_POINT ( 'NONE',  ( -7.717505791104999346, 1516.857914730730045, 201.4043401791270185 ) ) ;
#52747=CARTESIAN_POINT ( 'NONE',  ( -15.84317036476499929, 1513.136578080079744, 223.4420747407669978 ) ) ;
#52752=CARTESIAN_POINT ( 'NONE',  ( 2.283570633165000086, 1516.909589401870107, 206.2402975076569760 ) ) ;
#52786=EDGE_CURVE ( 'NONE', #72650, #28577, #19837, .T. ) ;
#52794=B_SPLINE_SURFACE_WITH_KNOTS ( 'NONE', 5, 5, ( 
 ( #21765, #82254, #55966, #6649, #92301, #22316, #73312, #13373, #6095 ),
 ( #31848, #72767, #23442, #32411, #13928, #106895, #22871, #81683, #39134 ),
 ( #66034, #107998, #31295, #100157, #107448, #64925, #99038, #40802, #56518 ),
 ( #99588, #90645, #57080, #8843, #77725, #59832, #75533, #109668, #92855 ),
 ( #43026, #69344, #18342, #17777, #32944, #25085, #1038, #16131, #33485 ),
 ( #67134, #67687, #41915, #68250, #94504, #8294, #77184, #93406, #16671 ) ),
 .UNSPECIFIED., .F., .F., .F.,
 ( 6, 6 ),
 ( 6, 3, 6 ),
 ( 4.238752792101360356, 5.659133035218639307 ),
 ( -0.001527176327848870111, 0.5000000000000000000, 1.002061266618639923 ),
 .UNSPECIFIED. ) ;
#52807=CARTESIAN_POINT ( 'NONE',  ( -0.01306004006829850073, 1516.939762005280045, 204.5032625402269844 ) ) ;
#52809=CARTESIAN_POINT ( 'NONE',  ( 14.83698683853499922, 1514.217947259989842, 193.9974257499669932 ) ) ;
#52822=CARTESIAN_POINT ( 'NONE',  ( -3.487592469308334220, 1508.551704408389469, 213.9802063543035331 ) ) ;
#52830=CARTESIAN_POINT ( 'NONE',  ( -6.546951720715000533, 1516.606339319019980, 211.9964348928969855 ) ) ;
#52833=VECTOR ( 'NONE', #51172, 1000.000000000000114 ) ;
#52836=CARTESIAN_POINT ( 'NONE',  ( 7.284055418254999914, 1511.816633140279919, 202.4402870219569763 ) ) ;
#52844=CARTESIAN_POINT ( 'NONE',  ( -7.843966652515001137, 1513.355826799109764, 216.6951227995569980 ) ) ;
#52845=CARTESIAN_POINT ( 'NONE',  ( 16.60697870052440095, 1513.055456493448446, 197.0683699863935772 ) ) ;
#52854=CARTESIAN_POINT ( 'NONE',  ( 2.864972116015000125, 1516.859514182039902, 206.2412530031170093 ) ) ;
#52870=CARTESIAN_POINT ( 'NONE',  ( 3.456007385174999946, 1516.647534046129977, 215.6697273451470096 ) ) ;
#52872=CARTESIAN_POINT ( 'NONE',  ( 5.705922834103000163, 1511.346048414110101, 217.0427200209030048 ) ) ;
#52874=CARTESIAN_POINT ( 'NONE',  ( 3.461360093275000160, 1516.874084700499907, 212.3753080308970311 ) ) ;
#52875=VECTOR ( 'NONE', #8263, 1000.000000000000000 ) ;
#52883=CARTESIAN_POINT ( 'NONE',  ( -7.550503362009299835, 1510.480349264700180, 214.6730346447039892 ) ) ;
#52892=CARTESIAN_POINT ( 'NONE',  ( 3.449777315724999571, 1516.974592746400049, 204.1104779853070283 ) ) ;
#52929=CARTESIAN_POINT ( 'NONE',  ( 6.483466624646080589, 1516.674728680589396, 205.3469896361293365 ) ) ;
#52935=CARTESIAN_POINT ( 'NONE',  ( 7.716878902974999122, 1516.833976295079992, 201.7919207096969672 ) ) ;
#52950=CARTESIAN_POINT ( 'NONE',  ( -8.016996095914999287, 1511.645462744430006, 212.5548212549570053 ) ) ;
#52971=CARTESIAN_POINT ( 'NONE',  ( -3.255340964424999761, 1516.962555622980062, 213.7459452615670159 ) ) ;
#52972=CARTESIAN_POINT ( 'NONE',  ( 2.838446966914999869, 1511.534866634170157, 216.7374015997870060 ) ) ;
#52975=ORIENTED_EDGE ( 'NONE', *, *, #28120, .F. ) ;
#52978=CARTESIAN_POINT ( 'NONE',  ( -7.720650173434999708, 1516.977993847330026, 203.3422188780170075 ) ) ;
#52983=FACE_OUTER_BOUND ( 'NONE', #51181, .T. ) ;
#52986=VERTEX_POINT ( 'NONE', #100085 ) ;
#52993=CARTESIAN_POINT ( 'NONE',  ( 1.715704490974999885, 1516.757508073510053, 212.3732403323669757 ) ) ;
#52999=CARTESIAN_POINT ( 'NONE',  ( 5.775625077365000415, 1516.745833913490060, 208.3665194962490261 ) ) ;
#53014=CARTESIAN_POINT ( 'NONE',  ( 1.130607463874999885, 1516.632821972880038, 215.6700465578769865 ) ) ;
#53016=DIRECTION ( 'NONE',  ( 0.000000000000000000, 6.123233995736769734E-17, 1.000000000000000000 ) ) ;
#53017=CARTESIAN_POINT ( 'NONE',  ( 0.01010282929720150019, 1516.939452820819952, 216.8414868732370167 ) ) ;
#53024=CARTESIAN_POINT ( 'NONE',  ( 8.452787181503049752, 1511.603576927810082, 203.2583637611789982 ) ) ;
#53051=CARTESIAN_POINT ( 'NONE',  ( -2.325909182683589815, 1516.529980546390107, 201.4129274379639867 ) ) ;
#53086=CARTESIAN_POINT ( 'NONE',  ( -4.487358987605787775, 1509.034510030707679, 212.9235704655121424 ) ) ;
#53096=CARTESIAN_POINT ( 'NONE',  ( -1.701850495234999983, 1516.908147884120126, 210.2591426210370003 ) ) ;
#53097=CARTESIAN_POINT ( 'NONE',  ( -7.512750246095000861, 1509.038615934159907, 203.6084103740969908 ) ) ;
#53105=CARTESIAN_POINT ( 'NONE',  ( 3.415238410854999795, 1511.775527460079957, 205.7066075212470082 ) ) ;
#53108=DIRECTION ( 'NONE',  ( -0.8164965809278529330, 0.5773502691894464300, 0.000000000000000000 ) ) ;
#53114=CARTESIAN_POINT ( 'NONE',  ( 1.701850457105000158, 1516.908147884120126, 207.9845492812970065 ) ) ;
#53129=CARTESIAN_POINT ( 'NONE',  ( -4.987078454525000204, 1508.551704408389924, 209.1218459511669892 ) ) ;
#53130=CARTESIAN_POINT ( 'NONE',  ( 4.996642160164999957, 1516.697242742309982, 206.2447328616370044 ) ) ;
#53148=CARTESIAN_POINT ( 'NONE',  ( 4.329791490734999471, 1515.051704408389924, 205.7917117663469924 ) ) ;
#53150=CARTESIAN_POINT ( 'NONE',  ( 4.040527303974999818, 1516.815231249920089, 213.7327841816070020 ) ) ;
#53165=CARTESIAN_POINT ( 'NONE',  ( -1.906499758064230099E-08, 1515.051704408389924, 209.1218459511669892 ) ) ;
#53195=B_SPLINE_CURVE_WITH_KNOTS ( 'NONE', 5,
 ( #73665, #22100, #20460, #46273, #29425, #12638 ),
 .UNSPECIFIED., .F., .F.,
 ( 6, 6 ),
 ( 0.000000000000000000, 1.000000000000000000 ),
 .UNSPECIFIED. ) ;
#53224=CARTESIAN_POINT ( 'NONE',  ( 0.7351097711180020200, 1516.977504706749869, 206.6301902066870184 ) ) ;
#53237=CARTESIAN_POINT ( 'NONE',  ( 6.949574947644999945, 1517.102359858469754, 212.3809477691169718 ) ) ;
#53262=VECTOR ( 'NONE', #37642, 1000.000000000000000 ) ;
#53267=CARTESIAN_POINT ( 'NONE',  ( 6.940473334145000450, 1516.833525648419936, 202.5658237375970145 ) ) ;
#53268=CARTESIAN_POINT ( 'NONE',  ( -4.997718276504999224, 1516.693851263360102, 210.2547950466569944 ) ) ;
#53289=CARTESIAN_POINT ( 'NONE',  ( -6.262845595265000398, 1511.198876514819858, 201.6723168475869841 ) ) ;
#53311=CARTESIAN_POINT ( 'NONE',  ( -2.299656354225000143, 1516.843453247299749, 206.6453952679669896 ) ) ;
#53327=CARTESIAN_POINT ( 'NONE',  ( 5.761500013727863134, 1510.554407338701822, 216.6633153120424424 ) ) ;
#53361=LINE ( 'NONE', #80199, #53262 ) ;
#53363=CARTESIAN_POINT ( 'NONE',  ( 3.449149195745000007, 1516.947419719950176, 204.4980579627370219 ) ) ;
#53383=CARTESIAN_POINT ( 'NONE',  ( -6.935133418554999096, 1516.613881697390070, 212.3834819030570031 ) ) ;
#53403=CARTESIAN_POINT ( 'NONE',  ( 1.700706776364999895, 1516.923170579120097, 206.8211163054370161 ) ) ;
#53412=CARTESIAN_POINT ( 'NONE',  ( 15.15436960869729965, 1512.305164330070056, 196.2951117818919897 ) ) ;
#53422=CARTESIAN_POINT ( 'NONE',  ( 3.263521904354999670, 1516.676340709600026, 214.8942497445370066 ) ) ;
#53429=CARTESIAN_POINT ( 'NONE',  ( 0.01328393942530149870, 1516.939580991450157, 212.3834982571270018 ) ) ;
#53450=CARTESIAN_POINT ( 'NONE',  ( -5.784008673325000238, 1516.911981270829983, 204.1205073037870079 ) ) ;
#53478=CARTESIAN_POINT ( 'NONE',  ( -12.10384762496500066, 1512.631076693560090, 217.6901596511270043 ) ) ;
#53491=CARTESIAN_POINT ( 'NONE',  ( -1.128757599205000073, 1516.608208975040043, 201.4108789544669946 ) ) ;
#53495=CARTESIAN_POINT ( 'NONE',  ( -5.551188713984379852, 1510.480349263560129, 201.5713426139130320 ) ) ;
#53508=CARTESIAN_POINT ( 'NONE',  ( -8.245978546805000420, 1511.399604276809896, 214.2323161589669951 ) ) ;
#53528=CARTESIAN_POINT ( 'NONE',  ( 0.7553264358530019651, 1516.745833913490060, 214.8974710475970085 ) ) ;
#53529=CARTESIAN_POINT ( 'NONE',  ( 2.412416358654999815, 1511.982868782460173, 216.7116937071870097 ) ) ;
#53535=CARTESIAN_POINT ( 'NONE',  ( -2.489617576474999705, 1516.665179208830068, 204.1258511445269903 ) ) ;
#53542=VERTEX_POINT ( 'NONE', #42659 ) ;
#53549=CARTESIAN_POINT ( 'NONE',  ( -7.321455911854999776, 1516.545806094630279, 211.6076919691270177 ) ) ;
#53556=CARTESIAN_POINT ( 'NONE',  ( 2.297629621054999571, 1516.970035769810011, 209.8568691683980205 ) ) ;
#53565=CARTESIAN_POINT ( 'NONE',  ( 7.734617087614999775, 1513.613303996360173, 201.3001138717470155 ) ) ;
#53573=CARTESIAN_POINT ( 'NONE',  ( 2.874588922665000545, 1516.606339319019980, 215.6687976528169770 ) ) ;
#53585=CARTESIAN_POINT ( 'NONE',  ( 8.600792717434700307, 1511.535603804869879, 203.3761131401680018 ) ) ;
#53587=PLANE ( 'NONE',  #103292 ) ;
#53592=CARTESIAN_POINT ( 'NONE',  ( -13.40786186986500006, 1517.051704408389924, 199.6217297329870064 ) ) ;
#53616=CARTESIAN_POINT ( 'NONE',  ( -1.398549609401959826, 1516.583792872650065, 201.4115183126079955 ) ) ;
#53651=CARTESIAN_POINT ( 'NONE',  ( -2.782343519255962239, 1516.553084368694726, 201.4123224916152424 ) ) ;
#53661=CARTESIAN_POINT ( 'NONE',  ( -7.326072182274999456, 1516.714320817460020, 209.8751461055349807 ) ) ;
#53664=FACE_OUTER_BOUND ( 'NONE', #10733, .T. ) ;
#53672=( BOUNDED_CURVE ( )  B_SPLINE_CURVE ( 3, ( #15957, #5380, #31125, #50160 ),
 .UNSPECIFIED., .F., .F. ) 
 B_SPLINE_CURVE_WITH_KNOTS ( ( 4, 4 ),
 ( 0.9002477009694579424, 1.144704973640545909 ),
 .UNSPECIFIED. ) 
 CURVE ( )  GEOMETRIC_REPRESENTATION_ITEM ( )  RATIONAL_B_SPLINE_CURVE ( ( 1.000000000000000000, 0.9950262503666102987, 0.9950262503666102987, 1.000000000000000000 ) ) 
 REPRESENTATION_ITEM ( '' )  );
#53681=CARTESIAN_POINT ( 'NONE',  ( 2.868112131164999745, 1516.855632454399938, 208.3641823986619954 ) ) ;
#53699=CARTESIAN_POINT ( 'NONE',  ( -6.950214971414999887, 1517.129577905929864, 206.2502655435069983 ) ) ;
#53711=CARTESIAN_POINT ( 'NONE',  ( 7.457021537675000644, 1517.051697240460271, 213.5019697367769993 ) ) ;
#53720=CARTESIAN_POINT ( 'NONE',  ( -2.287084308194999860, 1517.068517094990057, 214.1351209316169957 ) ) ;
#53784=CIRCLE ( 'NONE', #84113, 1.000000000000000000 ) ;
#53793=CARTESIAN_POINT ( 'NONE',  ( -3.268859434184999913, 1516.922519270759949, 206.6438591998669949 ) ) ;
#53797=FACE_OUTER_BOUND ( 'NONE', #40960, .T. ) ;
#53804=CARTESIAN_POINT ( 'NONE',  ( -7.321455911854999776, 1516.545806094630279, 211.6076919691270177 ) ) ;
#53814=CARTESIAN_POINT ( 'NONE',  ( 14.09486193512188557, 1514.059034343702706, 225.7345132044199545 ) ) ;
#53831=CARTESIAN_POINT ( 'NONE',  ( -5.008848238024999233, 1516.858456333729919, 204.1217621043670079 ) ) ;
#53832=CARTESIAN_POINT ( 'NONE',  ( 3.463767257884999839, 1517.014196759610059, 210.8246003415769962 ) ) ;
#53836=CARTESIAN_POINT ( 'NONE',  ( 5.129994116337838861, 1511.406468244438429, 217.6882656312603785 ) ) ;
#53856=CARTESIAN_POINT ( 'NONE',  ( -7.569982699715000152, 1513.743447518339963, 202.8797921858770223 ) ) ;
#53861=EDGE_CURVE ( 'NONE', #21042, #30294, #65270, .T. ) ;
#53866=EDGE_LOOP ( 'NONE', ( #50301, #28320, #2178, #56259 ) ) ;
#53872=CARTESIAN_POINT ( 'NONE',  ( 14.76985291543500090, 1513.863307887919973, 224.0959146767670234 ) ) ;
#53881=CARTESIAN_POINT ( 'NONE',  ( -7.338411997524999286, 1517.170512887980067, 206.6372682748769876 ) ) ;
#53900=CARTESIAN_POINT ( 'NONE',  ( 5.707844853767014115, 1510.531931295588947, 216.6676495880327309 ) ) ;
#53934=CARTESIAN_POINT ( 'NONE',  ( -2.295485539174999978, 1516.651306816259876, 204.1261199623870368 ) ) ;
#53954=CARTESIAN_POINT ( 'NONE',  ( 6.949265646015000186, 1517.089216728169959, 212.5747629931370000 ) ) ;
#53964=EDGE_LOOP ( 'NONE', ( #78842, #21932, #41123, #43227, #16554 ) ) ;
#53974=CARTESIAN_POINT ( 'NONE',  ( -5.371346839171279974, 1516.551188146539971, 218.7599618298110045 ) ) ;
#53976=CARTESIAN_POINT ( 'NONE',  ( 3.251394362135000105, 1516.757508073510053, 207.4061414411269766 ) ) ;
#53981=CARTESIAN_POINT ( 'NONE',  ( -7.512750272452770162, 1509.038617453179995, 203.6086426773880191 ) ) ;
#53994=CARTESIAN_POINT ( 'NONE',  ( 2.874588922665000545, 1516.606339319019980, 215.6687976528169770 ) ) ;
#53996=CARTESIAN_POINT ( 'NONE',  ( 5.523053254439029836, 1510.639750819960000, 216.6759469071630235 ) ) ;
#53999=CARTESIAN_POINT ( 'NONE',  ( -4.997250192034999650, 1516.727068157269969, 212.3866247496169990 ) ) ;
#54018=CARTESIAN_POINT ( 'NONE',  ( 3.449149195745000007, 1516.947419719950176, 204.4980579627370219 ) ) ;
#54055=CARTESIAN_POINT ( 'NONE',  ( -14.74158148776499999, 1513.636261293280086, 193.1162984930670063 ) ) ;
#54061=CARTESIAN_POINT ( 'NONE',  ( 15.18044682233499998, 1511.791180387469922, 197.3654389570669991 ) ) ;
#54066=EDGE_LOOP ( 'NONE', ( #35130, #85717, #80908, #71976, #4397, #110073, #45015, #74238 ) ) ;
#54072=CARTESIAN_POINT ( 'NONE',  ( -8.652776140254999859, 1511.435001052829875, 214.5073691319269926 ) ) ;
#54092=CARTESIAN_POINT ( 'NONE',  ( -4.613762395014999740, 1516.939574742129935, 214.9064842900469898 ) ) ;
#54093=CARTESIAN_POINT ( 'NONE',  ( 2.841932018395000092, 1512.089957059379913, 216.8946056602869703 ) ) ;
#54098=CARTESIAN_POINT ( 'NONE',  ( 3.449149195745000007, 1516.947419719950176, 204.4980579627370219 ) ) ;
#54110=CARTESIAN_POINT ( 'NONE',  ( -1.119439127814999990, 1517.026534522949987, 212.3908711059869745 ) ) ;
#54116=CARTESIAN_POINT ( 'NONE',  ( -5.000330033664999618, 1516.770163853809890, 209.8779366980180328 ) ) ;
#54124=EDGE_CURVE ( 'NONE', #66885, #27633, #105121, .T. ) ;
#54130=CARTESIAN_POINT ( 'NONE',  ( 3.263521904354999670, 1516.676340709600026, 214.8942497445370066 ) ) ;
#54134=CARTESIAN_POINT ( 'NONE',  ( 3.260357128764999946, 1517.133889586189980, 201.3971135232069969 ) ) ;
#54139=CARTESIAN_POINT ( 'NONE',  ( 7.679314465743660278, 1511.182265711489890, 203.2312592673829670 ) ) ;
#54193=VERTEX_POINT ( 'NONE', #87586 ) ;
#54197=ADVANCED_FACE ( 'NONE', ( #43373 ), #1938, .F. ) ;
#54215=CARTESIAN_POINT ( 'NONE',  ( 5.011551368014999674, 1517.080322339569875, 209.8587501411369942 ) ) ;
#54223=CARTESIAN_POINT ( 'NONE',  ( -6.942344729965000738, 1516.810037859429940, 201.4055938791270250 ) ) ;
#54229=CARTESIAN_POINT ( 'NONE',  ( -2.299668004004999933, 1516.965971551240045, 208.0037412025070012 ) ) ;
#54233=EDGE_LOOP ( 'NONE', ( #13786, #30136, #82269, #104325 ) ) ;
#54246=CARTESIAN_POINT ( 'NONE',  ( 7.709032137684999952, 1516.534320418310244, 206.6366287381669906 ) ) ;
#54262=CARTESIAN_POINT ( 'NONE',  ( -0.7386049428049979992, 1517.122674412569950, 215.6839400395269877 ) ) ;
#54264=EDGE_LOOP ( 'NONE', ( #55748, #72337, #52581, #84085 ) ) ;
#54270=CARTESIAN_POINT ( 'NONE',  ( 8.656023402515000242, 1514.496907775660020, 214.3647812291569892 ) ) ;
#54284=EDGE_CURVE ( 'NONE', #68646, #37961, #26832, .T. ) ;
#54287=CARTESIAN_POINT ( 'NONE',  ( -7.512750246095000861, 1509.038615934159907, 203.6084103740969908 ) ) ;
#54328=DIRECTION ( 'NONE',  ( 0.01484500364079635246, -0.5669078173018518019, -0.8236474686107856380 ) ) ;
#54334=CARTESIAN_POINT ( 'NONE',  ( -5.012938901904998801, 1517.051603658920158, 206.6410320471169939 ) ) ;
#54343=EDGE_LOOP ( 'NONE', ( #94266, #95380, #43769, #59160 ) ) ;
#54355=CARTESIAN_POINT ( 'NONE',  ( 11.65717857212529296, 1512.939392324944947, 225.5530975207334166 ) ) ;
#54376=CARTESIAN_POINT ( 'NONE',  ( 7.325541787135000149, 1516.710692850270107, 204.1167749238070144 ) ) ;
#54379=CARTESIAN_POINT ( 'NONE',  ( 5.513435558552500559, 1508.551704408428805, 201.9802063542013855 ) ) ;
#54382=CARTESIAN_POINT ( 'NONE',  ( 4.487358956434530199, 1509.034509900239300, 212.9235808158116470 ) ) ;
#54398=CARTESIAN_POINT ( 'NONE',  ( -6.760013159984999298, 1512.520476835120007, 201.4807483541169972 ) ) ;
#54414=CARTESIAN_POINT ( 'NONE',  ( 14.46755550443499949, 1513.509764667529907, 224.2886214921669819 ) ) ;
#54418=B_SPLINE_CURVE_WITH_KNOTS ( 'NONE', 5,
 ( #33760, #76332, #92028, #23708, #40516, #83614, #84715, #58436, #75246 ),
 .UNSPECIFIED., .F., .F.,
 ( 6, 3, 6 ),
 ( 0.8631819983265639484, 2.053866004040000082, 3.194083030974049997 ),
 .UNSPECIFIED. ) ;
#54424=CARTESIAN_POINT ( 'NONE',  ( -4.044321718124999521, 1517.001127920769704, 206.8363583507369867 ) ) ;
#54437=ADVANCED_FACE ( 'NONE', ( #26411 ), #67899, .F. ) ;
#54479=CARTESIAN_POINT ( 'NONE',  ( 3.255967386345000047, 1516.989560013210166, 204.1101670940770134 ) ) ;
#54490=ORIENTED_EDGE ( 'NONE', *, *, #2861, .F. ) ;
#54501=CARTESIAN_POINT ( 'NONE',  ( 2.879642153204999833, 1516.812046502680005, 212.5681757458869754 ) ) ;
#54510=CARTESIAN_POINT ( 'NONE',  ( -7.381112355834999583, 1512.341575225279939, 215.8975307908470143 ) ) ;
#54511=CARTESIAN_POINT ( 'NONE',  ( 16.27599025125675070, 1514.537600256206815, 194.3631480892788943 ) ) ;
#54524=CARTESIAN_POINT ( 'NONE',  ( -5.788436372295000076, 1517.116049120239950, 206.8334885244969712 ) ) ;
#54535=CARTESIAN_POINT ( 'NONE',  ( -6.127742290290780325, 1511.645100227919784, 200.3268099136730314 ) ) ;
#54542=CARTESIAN_POINT ( 'NONE',  ( 0.01171160595180150039, 1516.939568781210028, 215.6786969668069958 ) ) ;
#54544=CARTESIAN_POINT ( 'NONE',  ( 5.987023787224379667, 1511.685461860059831, 217.5892553512100278 ) ) ;
#54546=CARTESIAN_POINT ( 'NONE',  ( 5.011678838024999472, 1516.989560013210166, 212.3778133565769792 ) ) ;
#54563=CARTESIAN_POINT ( 'NONE',  ( 1.704794803334999997, 1517.096587378560116, 204.4952540647470016 ) ) ;
#54593=ORIENTED_EDGE ( 'NONE', *, *, #76944, .T. ) ;
#54599=CARTESIAN_POINT ( 'NONE',  ( -14.28353075656500160, 1513.113451381389950, 193.4746005378669906 ) ) ;
#54617=CARTESIAN_POINT ( 'NONE',  ( -7.548872338225000256, 1510.418062979269962, 214.3032561208869993 ) ) ;
#54627=FACE_OUTER_BOUND ( 'NONE', #90014, .T. ) ;
#54637=CARTESIAN_POINT ( 'NONE',  ( 7.719392382375000139, 1516.929962200689943, 215.6766245038770080 ) ) ;
#54638=CARTESIAN_POINT ( 'NONE',  ( 2.566007165815000324, 1512.021995456199875, 216.7432650908669984 ) ) ;
#54644=CARTESIAN_POINT ( 'NONE',  ( -15.17646696946499851, 1516.904916668740043, 225.0580773729669772 ) ) ;
#54645=CARTESIAN_POINT ( 'NONE',  ( -3.266349512195000138, 1516.797038924770050, 205.0935381919470046 ) ) ;
#54656=CARTESIAN_POINT ( 'NONE',  ( -13.33054336736499934, 1517.051704408389924, 207.1218459511669892 ) ) ;
#54659=CARTESIAN_POINT ( 'NONE',  ( 7.724423394095000894, 1517.122088787240045, 212.5760185856570104 ) ) ;
#54663=VECTOR ( 'NONE', #43395, 1000.000000000000000 ) ;
#54665=CARTESIAN_POINT ( 'NONE',  ( 3.267039691854999983, 1517.012231669750008, 209.8574146130079896 ) ) ;
#54673=CARTESIAN_POINT ( 'NONE',  ( -7.396545081224999763, 1511.069621805459974, 215.4940135707269917 ) ) ;
#54676=CARTESIAN_POINT ( 'NONE',  ( 7.583791906034999641, 1511.751588929339960, 206.7961148284170179 ) ) ;
#54679=CARTESIAN_POINT ( 'NONE',  ( -4.033653302454999867, 1517.028034847769959, 215.6825881955670070 ) ) ;
#54684=CARTESIAN_POINT ( 'NONE',  ( 7.717505752974999744, 1516.857914730730045, 201.4043401791270185 ) ) ;
#54685=CARTESIAN_POINT ( 'NONE',  ( -16.11904265886499843, 1512.169992403149990, 220.5902712816669862 ) ) ;
#54706=DIRECTION ( 'NONE',  ( 0.7063774289747313251, 0.04540766091858271930, -0.7063774289747313251 ) ) ;
#54722=CARTESIAN_POINT ( 'NONE',  ( 13.52455577884570026, 1512.715996828750121, 224.4318246187129944 ) ) ;
#54741=ORIENTED_EDGE ( 'NONE', *, *, #24912, .T. ) ;
#54758=CARTESIAN_POINT ( 'NONE',  ( -4.997718276504999224, 1516.693851263360102, 210.2547950466569944 ) ) ;
#54764=CARTESIAN_POINT ( 'NONE',  ( 3.454172615424999648, 1517.122088787240045, 201.3974225380069925 ) ) ;
#54776=CARTESIAN_POINT ( 'NONE',  ( 8.790084679516168009, 1511.590044791230184, 203.1124153264186418 ) ) ;
#54784=CARTESIAN_POINT ( 'NONE',  ( -7.725372170364999569, 1517.158319634930194, 206.2490093095770192 ) ) ;
#54786=CARTESIAN_POINT ( 'NONE',  ( -2.234897892418939769, 1512.314859079350072, 200.5229006381079842 ) ) ;
#54800=CARTESIAN_POINT ( 'NONE',  ( 1.130607463874999885, 1516.632821972880038, 215.6700465578769865 ) ) ;
#54802=ORIENTED_EDGE ( 'NONE', *, *, #15076, .T. ) ;
#54848=EDGE_CURVE ( 'NONE', #39742, #89980, #98984, .T. ) ;
#54876=CARTESIAN_POINT ( 'NONE',  ( -2.494758036134999912, 1516.937508036699910, 207.4208181092269854 ) ) ;
#54895=CARTESIAN_POINT ( 'NONE',  ( 12.83556472445637731, 1513.363094763115669, 225.9021281388779698 ) ) ;
#54913=EDGE_LOOP ( 'NONE', ( #37169, #51743, #15000, #67257, #100867, #86848, #29073, #22159, #4642 ) ) ;
#54914=CARTESIAN_POINT ( 'NONE',  ( 2.480187016714999970, 1517.025470194390209, 204.4964864072570094 ) ) ;
#54918=CARTESIAN_POINT ( 'NONE',  ( 5.385523159618170297, 1511.435001054559962, 217.7746220610370074 ) ) ;
#54925=CARTESIAN_POINT ( 'NONE',  ( 11.95631296123499965, 1516.551704408390151, 202.1152804391970221 ) ) ;
#54936=CARTESIAN_POINT ( 'NONE',  ( -6.329634402605000432, 1512.038636172069801, 200.9147609774469743 ) ) ;
#54959=CARTESIAN_POINT ( 'NONE',  ( 11.75640697505575538, 1511.791180387471059, 224.3022927925875365 ) ) ;
#54963=CARTESIAN_POINT ( 'NONE',  ( -0.7579844201469989606, 1516.883361325900069, 206.8353730456769881 ) ) ;
#54966=AXIS2_PLACEMENT_3D ( 'NONE', #9875, #18259, #43495 ) ;
#54990=VECTOR ( 'NONE', #61052, 1000.000000000000000 ) ;
#55021=CARTESIAN_POINT ( 'NONE',  ( -6.946748557085000719, 1516.983995446890049, 204.1186252050270014 ) ) ;
#55050=CARTESIAN_POINT ( 'NONE',  ( -6.852741844795000148, 1514.298059036119867, 217.0646729429169852 ) ) ;
#55051=CARTESIAN_POINT ( 'NONE',  ( 16.78503325280423297, 1513.553906385955088, 195.8943387144314840 ) ) ;
#55059=CARTESIAN_POINT ( 'NONE',  ( -2.229731647334999955, 1512.142919181319940, 201.5278066827870020 ) ) ;
#55062=ORIENTED_EDGE ( 'NONE', *, *, #4288, .F. ) ;
#55063=CARTESIAN_POINT ( 'NONE',  ( -2.881548462575000080, 1516.909589401870107, 206.8382752989369919 ) ) ;
#55078=CARTESIAN_POINT ( 'NONE',  ( 16.87207549522816308, 1516.551188142743058, 222.4161009436613483 ) ) ;
#55083=CARTESIAN_POINT ( 'NONE',  ( 5.005071008295000290, 1516.710692850270107, 216.4473877573669824 ) ) ;
#55084=CARTESIAN_POINT ( 'NONE',  ( 7.717505752974999744, 1516.857914730730045, 201.4043401791270185 ) ) ;
#55087=CARTESIAN_POINT ( 'NONE',  ( 2.880592928985000079, 1516.859514182039902, 211.9868180862470126 ) ) ;
#55107=CARTESIAN_POINT ( 'NONE',  ( 7.710610402995000001, 1516.594591938570147, 205.6677260153969939 ) ) ;
#55115=CARTESIAN_POINT ( 'NONE',  ( -7.649034438594999763, 1514.243099272629934, 203.4721261815869866 ) ) ;
#55139=CARTESIAN_POINT ( 'NONE',  ( 8.412796040255942742, 1511.396722025158397, 204.4533818147023965 ) ) ;
#55148=CARTESIAN_POINT ( 'NONE',  ( -14.64758698596499897, 1513.486273623730085, 193.6399990342670208 ) ) ;
#55152=CARTESIAN_POINT ( 'NONE',  ( -4.035490750684999739, 1516.630499592039996, 201.4102952541169884 ) ) ;
#55165=CARTESIAN_POINT ( 'NONE',  ( -7.552141952424999971, 1510.542924508009946, 212.9021323590669965 ) ) ;
#55184=VECTOR ( 'NONE', #41728, 1000.000000000000000 ) ;
#55185=CARTESIAN_POINT ( 'NONE',  ( 4.038637462725000127, 1516.734985836460055, 214.8955147850770118 ) ) ;
#55193=CARTESIAN_POINT ( 'NONE',  ( -6.948321743994999800, 1517.049325831759916, 205.0875650164470017 ) ) ;
#55204=CARTESIAN_POINT ( 'NONE',  ( 0.7572979362240020995, 1516.829948096479939, 212.5714934102470011 ) ) ;
#55209=CARTESIAN_POINT ( 'NONE',  ( -7.708901244349819493, 1516.529320347400244, 211.1219528266759937 ) ) ;
#55210=CARTESIAN_POINT ( 'NONE',  ( 7.726684687535000151, 1517.208444099459939, 210.2479840788170122 ) ) ;
#55214=ORIENTED_EDGE ( 'NONE', *, *, #106560, .F. ) ;
#55223=CARTESIAN_POINT ( 'NONE',  ( 3.261007131564999995, 1516.596789218710001, 216.4445556570670135 ) ) ;
#55228=CARTESIAN_POINT ( 'NONE',  ( -4.036119682645000317, 1516.647924054489977, 201.7978713257969900 ) ) ;
#55230=ORIENTED_EDGE ( 'NONE', *, *, #78090, .F. ) ;
#55271=EDGE_LOOP ( 'NONE', ( #14149, #4306, #91440, #73389 ) ) ;
#55306=CARTESIAN_POINT ( 'NONE',  ( -7.321169269124999879, 1516.531533746980131, 210.8305669548069829 ) ) ;
#55313=ORIENTED_EDGE ( 'NONE', *, *, #109673, .F. ) ;
#55315=CARTESIAN_POINT ( 'NONE',  ( 0.7403205670290020635, 1517.139320148880188, 201.3969713189170250 ) ) ;
#55316=AXIS2_PLACEMENT_3D ( 'NONE', #51545, #43150, #59414 ) ;
#55336=CARTESIAN_POINT ( 'NONE',  ( 8.370528965525000586, 1511.388520542559945, 204.5794305421269996 ) ) ;
#55337=CARTESIAN_POINT ( 'NONE',  ( -7.337793750624999944, 1517.145312756229941, 206.2496372219370073 ) ) ;
#55340=CARTESIAN_POINT ( 'NONE',  ( -1.781283055790834124, 1516.548117337739768, 201.8347555902114152 ) ) ;
#55341=ORIENTED_EDGE ( 'NONE', *, *, #76138, .F. ) ;
#55353=CARTESIAN_POINT ( 'NONE',  ( -5.776491133374999976, 1516.858301627840092, 214.9045953718370185 ) ) ;
#55355=CARTESIAN_POINT ( 'NONE',  ( 7.708856534992840182, 1516.527614422059742, 207.0328371564550025 ) ) ;
#55366=EDGE_CURVE ( 'NONE', #17126, #89621, #109753, .T. ) ;
#55375=CARTESIAN_POINT ( 'NONE',  ( -6.036760179694757866, 1509.035273794851719, 201.6612099679530843 ) ) ;
#55385=VERTEX_POINT ( 'NONE', #58804 ) ;
#55399=CARTESIAN_POINT ( 'NONE',  ( -4.329791550921825660, 1515.051704408389924, 213.0376480771455761 ) ) ;
#55421=CARTESIAN_POINT ( 'NONE',  ( 3.253301381255000013, 1516.790374942449944, 207.9863856151469861 ) ) ;
#55437=CARTESIAN_POINT ( 'NONE',  ( -5.513435596746664835, 1508.909942010400982, 216.6312267329172130 ) ) ;
#55447=CARTESIAN_POINT ( 'NONE',  ( 14.59148176577614286, 1514.407859707509942, 225.5030876066963685 ) ) ;
#55461=FACE_OUTER_BOUND ( 'NONE', #63696, .T. ) ;
#55463=CARTESIAN_POINT ( 'NONE',  ( 7.713117802984999827, 1516.690345681169902, 204.1174038931170003 ) ) ;
#55486=CARTESIAN_POINT ( 'NONE',  ( -7.719525633314999524, 1513.939092156080051, 202.0215813447470055 ) ) ;
#55497=DIRECTION ( 'NONE',  ( 0.5224574779883525144, -0.7067418228232951183, -0.4770263929453549823 ) ) ;
#55501=CARTESIAN_POINT ( 'NONE',  ( 14.64758694783500026, 1513.486273623730085, 224.6036928680670144 ) ) ;
#55507=CARTESIAN_POINT ( 'NONE',  ( -5.013274999515000552, 1517.068517094990057, 206.8347616620369820 ) ) ;
#55528=CARTESIAN_POINT ( 'NONE',  ( 6.023224921602742477, 1510.704533479030715, 216.6230964488122765 ) ) ;
#55532=LINE ( 'NONE', #56070, #24985 ) ;
#55566=CARTESIAN_POINT ( 'NONE',  ( -0.7568987378019988999, 1516.805675336850072, 205.0906771642370074 ) ) ;
#55569=ORIENTED_EDGE ( 'NONE', *, *, #82960, .F. ) ;
#55583=CARTESIAN_POINT ( 'NONE',  ( -4.997718276504999224, 1516.693851263360102, 210.2547950466569944 ) ) ;
#55601=CARTESIAN_POINT ( 'NONE',  ( -6.321172872105000451, 1513.830194289070278, 216.6922650853570076 ) ) ;
#55614=CARTESIAN_POINT ( 'NONE',  ( 6.546001350565000543, 1516.557392317769882, 207.4118413833070065 ) ) ;
#55626=CARTESIAN_POINT ( 'NONE',  ( -5.570674267431350302, 1511.275365984429982, 201.2227656140939871 ) ) ;
#55629=CARTESIAN_POINT ( 'NONE',  ( -5.707844849875344906, 1510.531931279475430, 201.5760423114203377 ) ) ;
#55633=CARTESIAN_POINT ( 'NONE',  ( 7.718763505904999711, 1516.905946377369901, 216.0642002436470079 ) ) ;
#55638=CARTESIAN_POINT ( 'NONE',  ( 5.786527562335000319, 1517.025653221279981, 212.5728793591970032 ) ) ;
#55655=CARTESIAN_POINT ( 'NONE',  ( -4.622842882315000068, 1516.901952101700090, 205.0913314195169903 ) ) ;
#55678=CARTESIAN_POINT ( 'NONE',  ( -11.11248229347330430, 1512.836812602111877, 193.0596162085393814 ) ) ;
#55681=CARTESIAN_POINT ( 'NONE',  ( -3.727807290641250049, 1517.051706635029859, 215.7383534543289727 ) ) ;
#55684=CARTESIAN_POINT ( 'NONE',  ( 8.335839316101193219, 1511.410080502129176, 204.6879527979276929 ) ) ;
#55688=EDGE_CURVE ( 'NONE', #85013, #21616, #57039, .T. ) ;
#55696=CARTESIAN_POINT ( 'NONE',  ( -11.92849872886499973, 1511.839858410419993, 194.1166199672670132 ) ) ;
#55700=CARTESIAN_POINT ( 'NONE',  ( -6.555393155154999540, 1516.809497469189864, 201.7937966518470034 ) ) ;
#55731=VERTEX_POINT ( 'NONE', #102308 ) ;
#55737=CARTESIAN_POINT ( 'NONE',  ( -3.449777353855000062, 1516.974592746400049, 214.1332139170270068 ) ) ;
#55747=CARTESIAN_POINT ( 'NONE',  ( -5.785582951674999919, 1516.981965530290154, 205.0894480302270040 ) ) ;
#55748=ORIENTED_EDGE ( 'NONE', *, *, #49017, .F. ) ;
#55754=EDGE_CURVE ( 'NONE', #98450, #44161, #43534, .T. ) ;
#55762=CARTESIAN_POINT ( 'NONE',  ( -3.253462098795000035, 1516.874084700499907, 212.5832060635069922 ) ) ;
#55769=CARTESIAN_POINT ( 'NONE',  ( -1.117840124865000062, 1516.949031626070109, 210.8389850543470061 ) ) ;
#55782=CARTESIAN_POINT ( 'NONE',  ( 5.005071008295000290, 1516.710692850270107, 216.4473877573669824 ) ) ;
#55786=CARTESIAN_POINT ( 'NONE',  ( 6.941727252324999320, 1516.882217593000178, 201.7906628411569727 ) ) ;
#55787=CARTESIAN_POINT ( 'NONE',  ( -15.90990259576500065, 1512.830284628050094, 220.0820010595669771 ) ) ;
#55816=CYLINDRICAL_SURFACE ( 'NONE', #10746, 7.500000000000000000 ) ;
#55862=CARTESIAN_POINT ( 'NONE',  ( -2.282622950494999969, 1516.861367446839949, 211.4218295478370067 ) ) ;
#55864=CARTESIAN_POINT ( 'NONE',  ( -4.608417544644999531, 1516.691389976299888, 211.6120918846570191 ) ) ;
#55871=CARTESIAN_POINT ( 'NONE',  ( -0.01010286742719850028, 1516.939452820819952, 201.4022050290969901 ) ) ;
#55885=CARTESIAN_POINT ( 'NONE',  ( 0.01265818781360149997, 1516.959716008189844, 210.8316124642570060 ) ) ;
#55890=CARTESIAN_POINT ( 'NONE',  ( 7.937216453355000034, 1511.802450769970164, 205.9560045756870181 ) ) ;
#55891=CARTESIAN_POINT ( 'NONE',  ( -2.493073867885000183, 1516.826109302209943, 206.2575198447970024 ) ) ;
#55895=CARTESIAN_POINT ( 'NONE',  ( -3.254300203878770503, 1516.622698719769687, 202.3553198114061047 ) ) ;
#55907=CARTESIAN_POINT ( 'NONE',  ( -3.257220640824999958, 1517.040132827679827, 214.9086836491569841 ) ) ;
#55909=CARTESIAN_POINT ( 'NONE',  ( 7.709748394418160622, 1516.561673159430029, 207.5610261272159960 ) ) ;
#55931=CARTESIAN_POINT ( 'NONE',  ( -4.826478521064999860, 1511.220390575160081, 201.2328893641169714 ) ) ;
#55946=CARTESIAN_POINT ( 'NONE',  ( 3.487592428935230249, 1508.551704408389924, 214.1089243929580164 ) ) ;
#55966=CARTESIAN_POINT ( 'NONE',  ( -8.474723756492620552, 1511.779111711370206, 215.2118351801979941 ) ) ;
#55970=CARTESIAN_POINT ( 'NONE',  ( 4.608021669135000664, 1516.660388280709867, 207.4085285224269910 ) ) ;
#55992=CARTESIAN_POINT ( 'NONE',  ( 13.24891926068781878, 1513.564960623643401, 225.9057560452617963 ) ) ;
#55999=CARTESIAN_POINT ( 'NONE',  ( 3.487586041942699833, 1508.611352721110052, 204.4436967962270160 ) ) ;
#56007=CARTESIAN_POINT ( 'NONE',  ( 1.705466410464999916, 1517.120861839400050, 204.1076508302870138 ) ) ;
#56027=CARTESIAN_POINT ( 'NONE',  ( -7.891962451154999059, 1514.771170611759999, 203.1042818683069981 ) ) ;
#56040=CARTESIAN_POINT ( 'NONE',  ( 14.32514190893500050, 1513.248517198770060, 225.3451382666669929 ) ) ;
#56041=CARTESIAN_POINT ( 'NONE',  ( -17.15254157612219643, 1516.551704399882283, 221.3246399025400706 ) ) ;
#56046=CARTESIAN_POINT ( 'NONE',  ( 7.321169230994999388, 1516.531533746980131, 207.4131249475269954 ) ) ;
#56059=CARTESIAN_POINT ( 'NONE',  ( 2.248963467334999855, 1512.851027015570025, 217.7347704682469782 ) ) ;
#56070=CARTESIAN_POINT ( 'NONE',  ( -2.234923479105000332, 1512.341036988540054, 201.5226187854269995 ) ) ;
#56089=FILL_AREA_STYLE_COLOUR ( '', #51719 ) ;
#56102=CARTESIAN_POINT ( 'NONE',  ( -0.01322039564809850132, 1516.939819969850078, 205.0847949345169923 ) ) ;
#56107=ORIENTED_EDGE ( 'NONE', *, *, #68632, .F. ) ;
#56115=CARTESIAN_POINT ( 'NONE',  ( -7.323390445344999833, 1516.613712827999962, 210.2512321725070024 ) ) ;
#56140=CARTESIAN_POINT ( 'NONE',  ( -4.625790014595000166, 1517.104192383289956, 208.0004623403669939 ) ) ;
#56154=FACE_OUTER_BOUND ( 'NONE', #44704, .T. ) ;
#56158=CARTESIAN_POINT ( 'NONE',  ( 2.873958851594999864, 1516.588006113850042, 216.0563744999969913 ) ) ;
#56162=CARTESIAN_POINT ( 'NONE',  ( 0.7568986996720019622, 1516.805675336850072, 213.1530147380969993 ) ) ;
#56180=CARTESIAN_POINT ( 'NONE',  ( -2.490245952555000031, 1516.691389976299888, 204.5134284255869943 ) ) ;
#56187=CARTESIAN_POINT ( 'NONE',  ( -7.150360519070535936, 1512.239113741255551, 202.0236829662010791 ) ) ;
#56190=FACE_OUTER_BOUND ( 'NONE', #33041, .T. ) ;
#56208=FACE_OUTER_BOUND ( 'NONE', #32284, .T. ) ;
#56225=CARTESIAN_POINT ( 'NONE',  ( -11.46842534956499904, 1512.169992403149990, 193.0028033113669892 ) ) ;
#56227=EDGE_CURVE ( 'NONE', #51438, #53542, #98150, .T. ) ;
#56229=CARTESIAN_POINT ( 'NONE',  ( 1.124894050234999998, 1517.194816588360027, 202.1703287997270309 ) ) ;
#56237=CARTESIAN_POINT ( 'NONE',  ( 3.487592431604999987, 1508.551704408389924, 204.1347675156769981 ) ) ;
#56245=CARTESIAN_POINT ( 'NONE',  ( -7.684243113244999535, 1511.930588878439949, 211.8885908927369996 ) ) ;
#56259=ORIENTED_EDGE ( 'NONE', *, *, #64711, .F. ) ;
#56265=CARTESIAN_POINT ( 'NONE',  ( -7.716252091104999877, 1516.810037859429940, 216.0641906620670056 ) ) ;
#56273=CARTESIAN_POINT ( 'NONE',  ( 4.611879685325000366, 1516.858533673840157, 204.4999481076869756 ) ) ;
#56275=CARTESIAN_POINT ( 'NONE',  ( -0.7468175536419978666, 1517.006509894990131, 209.1289748073840258 ) ) ;
#56278=CARTESIAN_POINT ( 'NONE',  ( 6.681558910155000142, 1511.816633140289923, 216.4059013884869955 ) ) ;
#56289=CARTESIAN_POINT ( 'NONE',  ( 6.561686423234999843, 1517.069378699710114, 212.5741351528070027 ) ) ;
#56296=CARTESIAN_POINT ( 'NONE',  ( -6.546001388695000145, 1516.557392317769882, 210.8318505190270002 ) ) ;
#56301=ORIENTED_EDGE ( 'NONE', *, *, #15964, .F. ) ;
#56310=CARTESIAN_POINT ( 'NONE',  ( -3.453544863754999472, 1517.106845464700200, 216.4586906126469898 ) ) ;
#56315=CARTESIAN_POINT ( 'NONE',  ( -4.617490504904999682, 1516.685667699390024, 201.7969310139470167 ) ) ;
#56316=CARTESIAN_POINT ( 'NONE',  ( -15.00522600296499931, 1511.839858410419993, 221.0503446609669993 ) ) ;
#56348=CARTESIAN_POINT ( 'NONE',  ( -4.987078467906759904, 1508.551704408389924, 213.0804802153340063 ) ) ;
#56357=CARTESIAN_POINT ( 'NONE',  ( 14.35493910357529934, 1513.426431439630278, 224.2887426523980139 ) ) ;
#56395=ORIENTED_EDGE ( 'NONE', *, *, #2861, .T. ) ;
#56397=CARTESIAN_POINT ( 'NONE',  ( 4.625693865015000128, 1517.042661899400173, 211.4082922958669997 ) ) ;
#56400=CARTESIAN_POINT ( 'NONE',  ( -6.934528567894999718, 1516.588006113850042, 211.9958048218269937 ) ) ;
#56408=CARTESIAN_POINT ( 'NONE',  ( 7.328676169885000036, 1516.833844030519913, 202.1788723028969912 ) ) ;
#56412=( BOUNDED_CURVE ( )  B_SPLINE_CURVE ( 3, ( #23585, #65619, #58860, #16266 ),
 .UNSPECIFIED., .F., .T. ) 
 B_SPLINE_CURVE_WITH_KNOTS ( ( 4, 4 ),
 ( 5.447131716497097820, 6.315249268837944463 ),
 .UNSPECIFIED. ) 
 CURVE ( )  GEOMETRIC_REPRESENTATION_ITEM ( )  RATIONAL_B_SPLINE_CURVE ( ( 1.000000000000000000, 0.9381775213689819148, 0.9381775213689819148, 1.000000000000000000 ) ) 
 REPRESENTATION_ITEM ( '' )  );
#56424=CARTESIAN_POINT ( 'NONE',  ( 2.882325979385000014, 1516.969638403840008, 210.8235757905769674 ) ) ;
#56429=CARTESIAN_POINT ( 'NONE',  ( 7.556166211784999476, 1510.696675236759802, 204.6602201360370259 ) ) ;
#56430=CARTESIAN_POINT ( 'NONE',  ( 6.935801261535000428, 1516.621991115350056, 207.9918434378369909 ) ) ;
#56433=CARTESIAN_POINT ( 'NONE',  ( -1.275439650553358728, 1516.597747113053174, 201.7236143332039546 ) ) ;
#56436=EDGE_CURVE ( 'NONE', #27843, #56695, #24496, .T. ) ;
#56446=CARTESIAN_POINT ( 'NONE',  ( -1.708102627415000185, 1517.199196846569976, 215.6864246554469844 ) ) ;
#56448=CARTESIAN_POINT ( 'NONE',  ( 7.708922318049459932, 1516.530126575629993, 206.7990132384589970 ) ) ;
#56449=CARTESIAN_POINT ( 'NONE',  ( -7.722580352405000070, 1517.051704408389924, 207.5526846776770071 ) ) ;
#56473=ADVANCED_FACE ( 'NONE', ( #56208 ), #87188, .T. ) ;
#56478=CARTESIAN_POINT ( 'NONE',  ( -3.173602190014999991, 1510.830536680500245, 201.5621726280170094 ) ) ;
#56511=CARTESIAN_POINT ( 'NONE',  ( -6.766140062282060441, 1508.878901399440110, 216.3823901328790100 ) ) ;
#56518=CARTESIAN_POINT ( 'NONE',  ( -7.494431781837549877, 1510.714321716100130, 215.2145461046430057 ) ) ;
#56522=CARTESIAN_POINT ( 'NONE',  ( -2.881325412095000260, 1517.003078582959688, 208.0029426616869728 ) ) ;
#56550=CARTESIAN_POINT ( 'NONE',  ( 3.958644637644479491, 1508.551704408389924, 204.1347649932010029 ) ) ;
#56551=CARTESIAN_POINT ( 'NONE',  ( -9.126915939008458878, 1516.551188146008599, 204.3103848001327663 ) ) ;
#56557=CARTESIAN_POINT ( 'NONE',  ( -3.801724410738229754, 1509.034524880150002, 204.6344874940000125 ) ) ;
#56559=CARTESIAN_POINT ( 'NONE',  ( -0.01322039564809850132, 1516.939819969850078, 205.0847949345169923 ) ) ;
#56563=ORIENTED_EDGE ( 'NONE', *, *, #104723, .T. ) ;
#56573=FACE_OUTER_BOUND ( 'NONE', #81529, .T. ) ;
#56650=CARTESIAN_POINT ( 'NONE',  ( -4.873140598966017478, 1511.395875706939250, 200.6411893189262798 ) ) ;
#56657=CARTESIAN_POINT ( 'NONE',  ( 3.447264348965000558, 1516.858765657450249, 205.6607986404769974 ) ) ;
#56671=CARTESIAN_POINT ( 'NONE',  ( 5.788691325514999875, 1517.157901477309906, 210.2449475486469908 ) ) ;
#56683=CARTESIAN_POINT ( 'NONE',  ( -7.100264625464999924, 1513.939092156100060, 216.8413715654270106 ) ) ;
#56695=VERTEX_POINT ( 'NONE', #70979 ) ;
#56697=CARTESIAN_POINT ( 'NONE',  ( 1.701850457105000158, 1516.908147884120126, 207.9845492812970065 ) ) ;
#56716=CARTESIAN_POINT ( 'NONE',  ( -2.872836660654999985, 1517.158319634930194, 216.8472181024670249 ) ) ;
#56721=CARTESIAN_POINT ( 'NONE',  ( 6.561686423234999843, 1517.069378699710114, 212.5741351528070027 ) ) ;
#56724=CARTESIAN_POINT ( 'NONE',  ( 3.487587010931929576, 1508.884219112060009, 213.6131341179649894 ) ) ;
#56739=VERTEX_POINT ( 'NONE', #45208 ) ;
#56740=CARTESIAN_POINT ( 'NONE',  ( -5.009478105444999940, 1516.886345593249871, 204.5093386581970094 ) ) ;
#56770=CARTESIAN_POINT ( 'NONE',  ( 8.100258108500456800, 1511.553933485576636, 205.4225227818773476 ) ) ;
#56776=CARTESIAN_POINT ( 'NONE',  ( -7.428892777654675150, 1510.947107019768737, 215.4107650370616795 ) ) ;
#56783=CARTESIAN_POINT ( 'NONE',  ( -4.618119704395000191, 1516.706638732659940, 202.1845071865270143 ) ) ;
#56787=CARTESIAN_POINT ( 'NONE',  ( 15.56957301243500069, 1512.571022561229938, 195.5563796964669905 ) ) ;
#56792=EDGE_LOOP ( 'NONE', ( #100280, #65597, #9507, #28240, #56395, #90132, #12443, #7105, #24380 ) ) ;
#56799=CARTESIAN_POINT ( 'NONE',  ( -7.594504679555000415, 1512.160709093490141, 211.5076181542869733 ) ) ;
#56820=CARTESIAN_POINT ( 'NONE',  ( -2.290256301855000398, 1517.170721208160103, 216.0730210990169837 ) ) ;
#56828=CARTESIAN_POINT ( 'NONE',  ( 1.702754371344999962, 1517.014196759610059, 205.6580786742169948 ) ) ;
#56830=CARTESIAN_POINT ( 'NONE',  ( -2.480427292634999947, 1516.872851364150165, 209.8797317620669673 ) ) ;
#56837=ORIENTED_EDGE ( 'NONE', *, *, #37742, .T. ) ;
#56844=CARTESIAN_POINT ( 'NONE',  ( 3.265407117845000151, 1516.754149861460064, 213.7315192116670062 ) ) ;
#56850=CARTESIAN_POINT ( 'NONE',  ( -7.708745685915000756, 1516.523379810429788, 210.8299382363969983 ) ) ;
#56859=DIRECTION ( 'NONE',  ( 0.7384854939282339270, -4.299975059343909233E-13, -0.6742693640212139572 ) ) ;
#56865=CARTESIAN_POINT ( 'NONE',  ( 7.329925222404999552, 1516.833976295079992, 216.8387248732070134 ) ) ;
#56871=CARTESIAN_POINT ( 'NONE',  ( 4.034908559714999399, 1517.068717944079935, 201.7859449365070077 ) ) ;
#56898=DIRECTION ( 'NONE',  ( 0.000000000000000000, -1.000000000000000000, -2.307067265786200309E-16 ) ) ;
#56905=CARTESIAN_POINT ( 'NONE',  ( 12.57832847022450018, 1512.205851781549882, 224.1512894226670198 ) ) ;
#56909=CARTESIAN_POINT ( 'NONE',  ( 6.354226016189142179, 1516.697111559987889, 205.1358369536649775 ) ) ;
#56931=ORIENTED_EDGE ( 'NONE', *, *, #25623, .F. ) ;
#56951=CARTESIAN_POINT ( 'NONE',  ( -6.935801299664999142, 1516.621991115350056, 210.2518484644969874 ) ) ;
#56956=CARTESIAN_POINT ( 'NONE',  ( -6.547556969464999987, 1516.633288330999903, 212.3841106205370011 ) ) ;
#56964=CARTESIAN_POINT ( 'NONE',  ( -3.456007423304999993, 1516.647534046129977, 202.5739645571870255 ) ) ;
#56965=CARTESIAN_POINT ( 'NONE',  ( 1.999999980934999977, 1520.551704408390151, 195.7913026028670060 ) ) ;
#56974=PLANE ( 'NONE',  #38601 ) ;
#56980=CARTESIAN_POINT ( 'NONE',  ( -2.477975353594999763, 1516.839862955080207, 210.2583935552169976 ) ) ;
#56986=CARTESIAN_POINT ( 'NONE',  ( 7.983219816825001480, 1511.369014903080142, 203.7222546344770251 ) ) ;
#56987=CARTESIAN_POINT ( 'NONE',  ( 2.476450664134999702, 1516.843453247299749, 206.8221896160070230 ) ) ;
#56991=ADVANCED_FACE ( 'NONE', ( #39690 ), #65466, .F. ) ;
#56994=DIRECTION ( 'NONE',  ( -0.9996573249755574819, -0.02617694830786557875, 0.000000000000000000 ) ) ;
#57008=CARTESIAN_POINT ( 'NONE',  ( 3.261007131564999995, 1516.596789218710001, 216.4445556570670135 ) ) ;
#57010=CARTESIAN_POINT ( 'NONE',  ( 7.709220066765960055, 1516.541497140389993, 207.3539078949219743 ) ) ;
#57039=LINE ( 'NONE', #73268, #50480 ) ;
#57041=CARTESIAN_POINT ( 'NONE',  ( -4.542415428115000431, 1511.388520542559945, 200.7513169665770079 ) ) ;
#57056=LINE ( 'NONE', #80588, #26150 ) ;
#57080=CARTESIAN_POINT ( 'NONE',  ( -8.424736004331359496, 1511.534310205860038, 214.8401254943979950 ) ) ;
#57086=CARTESIAN_POINT ( 'NONE',  ( 1.117840086735000016, 1516.949031626070109, 207.4047068479870006 ) ) ;
#57096=CARTESIAN_POINT ( 'NONE',  ( -15.00007760880209950, 1512.191474810040063, 221.6539140102569831 ) ) ;
#57108=ORIENTED_EDGE ( 'NONE', *, *, #34951, .T. ) ;
#57120=CARTESIAN_POINT ( 'NONE',  ( -4.115862995762159748, 1509.032029411810072, 204.7576468414000033 ) ) ;
#57122=CARTESIAN_POINT ( 'NONE',  ( -4.622842882315000068, 1516.901952101700090, 205.0913314195169903 ) ) ;
#57125=CARTESIAN_POINT ( 'NONE',  ( 14.82736035860130031, 1512.135905030570029, 196.8226469024940002 ) ) ;
#57131=CARTESIAN_POINT ( 'NONE',  ( -12.26154103078309987, 1512.129944624190102, 194.3268994079789991 ) ) ;
#57210=SURFACE_STYLE_USAGE ( .BOTH. , #5688 ) ;
#57224=CARTESIAN_POINT ( 'NONE',  ( -6.561686461364999445, 1517.069378699710114, 205.6695567495270041 ) ) ;
#57238=CARTESIAN_POINT ( 'NONE',  ( 7.726684687535000151, 1517.208444099459939, 210.2479840788170122 ) ) ;
#57256=CARTESIAN_POINT ( 'NONE',  ( -7.179127119344999919, 1513.978875661350230, 216.9309098834470149 ) ) ;
#57263=EDGE_CURVE ( 'NONE', #12028, #84553, #83213, .T. ) ;
#57271=CARTESIAN_POINT ( 'NONE',  ( 5.778999773775000293, 1516.955859323880077, 201.7887757972170277 ) ) ;
#57272=CARTESIAN_POINT ( 'NONE',  ( -2.299668004004999933, 1516.965971551240045, 208.0037412025070012 ) ) ;
#57278=CYLINDRICAL_SURFACE ( 'NONE', #5507, 0.9999999999999988898 ) ;
#57282=DIRECTION ( 'NONE',  ( 0.000000000000000000, -1.000000000000000000, 6.123233995736769734E-17 ) ) ;
#57292=CARTESIAN_POINT ( 'NONE',  ( -7.717505791104999346, 1516.857914730730045, 216.8393517232070167 ) ) ;
#57294=DIRECTION ( 'NONE',  ( 0.000000000000000000, 0.06174578541841399537, -0.9980919085851078787 ) ) ;
#57297=CARTESIAN_POINT ( 'NONE',  ( 3.267291605165000057, 1516.842852731759876, 212.5687880419470162 ) ) ;
#57300=CARTESIAN_POINT ( 'NONE',  ( 2.344512076345889984, 1516.526058371499857, 216.8306617650070223 ) ) ;
#57309=CARTESIAN_POINT ( 'NONE',  ( -1.906499758064230099E-08, 1508.551704408389924, 201.6218459511669892 ) ) ;
#57314=CARTESIAN_POINT ( 'NONE',  ( -2.298048961635000165, 1516.764084769670262, 205.6764383981169715 ) ) ;
#57322=VECTOR ( 'NONE', #15437, 1000.000000000000000 ) ;
#57343=CARTESIAN_POINT ( 'NONE',  ( 8.480624627922136227, 1511.395873689150676, 204.2487940905495236 ) ) ;
#57350=CARTESIAN_POINT ( 'NONE',  ( -7.481780884509355189, 1510.769285161464495, 215.2273066580793852 ) ) ;
#57358=CARTESIAN_POINT ( 'NONE',  ( 4.033653264325000265, 1517.028034847769959, 202.5611037067669997 ) ) ;
#57361=CARTESIAN_POINT ( 'NONE',  ( 15.25940256903500014, 1512.044075975079977, 196.5523931850670181 ) ) ;
#57370=ORIENTED_EDGE ( 'NONE', *, *, #11025, .F. ) ;
#57373=CARTESIAN_POINT ( 'NONE',  ( -7.599119446864999183, 1512.336926113599930, 211.5138630182570125 ) ) ;
#57385=ORIENTED_EDGE ( 'NONE', *, *, #80132, .F. ) ;
#57388=ORIENTED_EDGE ( 'NONE', *, *, #105951, .F. ) ;
#57392=CARTESIAN_POINT ( 'NONE',  ( 6.556022194504999234, 1516.833525648419936, 216.0623193043769845 ) ) ;
#57400=CARTESIAN_POINT ( 'NONE',  ( 4.609996581545000360, 1516.769879638719885, 205.6626893540170329 ) ) ;
#57402=CARTESIAN_POINT ( 'NONE',  ( -6.556851034704999748, 1516.939568781210028, 209.1335575761840175 ) ) ;
#57407=CARTESIAN_POINT ( 'NONE',  ( 6.843878216475000720, 1512.371933174400056, 217.6246419884270153 ) ) ;
#57415=CARTESIAN_POINT ( 'NONE',  ( 5.009478067315000338, 1516.886345593249871, 213.7343532441369973 ) ) ;
#57419=CARTESIAN_POINT ( 'NONE',  ( -7.708976442096130199, 1516.532192033489991, 211.5084644598540251 ) ) ;
#57420=CARTESIAN_POINT ( 'NONE',  ( 7.339749335215000059, 1517.224900789629828, 210.8312305431869902 ) ) ;
#57436=CARTESIAN_POINT ( 'NONE',  ( 6.942344691835000248, 1516.810037859429940, 216.8380980232070101 ) ) ;
#57440=ORIENTED_EDGE ( 'NONE', *, *, #92589, .T. ) ;
#57441=CARTESIAN_POINT ( 'NONE',  ( -4.618119704395000191, 1516.706638732659940, 202.1845071865270143 ) ) ;
#57442=CARTESIAN_POINT ( 'NONE',  ( -15.40521419186499941, 1513.907445464710236, 224.1476389979669932 ) ) ;
#57449=VECTOR ( 'NONE', #7567, 1000.000000000000000 ) ;
#57470=CARTESIAN_POINT ( 'NONE',  ( 4.805077557904999352, 1510.399296111369949, 216.6702268425969748 ) ) ;
#57512=CARTESIAN_POINT ( 'NONE',  ( -7.321455911854999776, 1516.545806094630279, 211.6076919691270177 ) ) ;
#57516=CARTESIAN_POINT ( 'NONE',  ( 6.561686423234999843, 1517.069378699710114, 212.5741351528070027 ) ) ;
#57522=CARTESIAN_POINT ( 'NONE',  ( 2.870951667784999994, 1517.111322026010157, 202.5592101095969895 ) ) ;
#57524=EDGE_CURVE ( 'NONE', #46347, #33692, #32500, .T. ) ;
#57538=CARTESIAN_POINT ( 'NONE',  ( 4.625359524845000792, 1517.025470194390209, 211.6020329869469947 ) ) ;
#57544=CARTESIAN_POINT ( 'NONE',  ( 7.888956567984999779, 1511.220390575160081, 204.2953674491570268 ) ) ;
#57545=CARTESIAN_POINT ( 'NONE',  ( -2.494758036134999912, 1516.937508036699910, 207.4208181092269854 ) ) ;
#57554=LINE ( 'NONE', #91677, #12757 ) ;
#57562=CARTESIAN_POINT ( 'NONE',  ( -7.500000019064997581, 1516.051704408390151, 209.1218459511669892 ) ) ;
#57563=CARTESIAN_POINT ( 'NONE',  ( -6.552897405075000847, 1516.858146885269889, 215.6784973415170157 ) ) ;
#57565=CARTESIAN_POINT ( 'NONE',  ( 7.714629857204999830, 1516.748088702300038, 208.4722268118290174 ) ) ;
#57580=ORIENTED_EDGE ( 'NONE', *, *, #990, .T. ) ;
#57593=CARTESIAN_POINT ( 'NONE',  ( -5.399591335754999832, 1511.369014903080142, 201.1386261152769919 ) ) ;
#57637=FACE_OUTER_BOUND ( 'NONE', #12044, .T. ) ;
#57643=CARTESIAN_POINT ( 'NONE',  ( 4.612671339784999880, 1516.783665406140017, 208.3654117178780041 ) ) ;
#57669=CARTESIAN_POINT ( 'NONE',  ( 3.822989240696690327, 1508.729442775010057, 204.5649349260539793 ) ) ;
#57675=CARTESIAN_POINT ( 'NONE',  ( -4.668116808335850187, 1508.551704407329908, 204.7884564220910022 ) ) ;
#57678=CARTESIAN_POINT ( 'NONE',  ( -6.560742263465000335, 1517.028034847769959, 205.0881926677770082 ) ) ;
#57681=CARTESIAN_POINT ( 'NONE',  ( 15.27803604049760011, 1512.526687531830021, 195.8825387542129874 ) ) ;
#57686=CARTESIAN_POINT ( 'NONE',  ( -13.77006425889850050, 1512.900351074040145, 193.8161084199589936 ) ) ;
#57707=LINE ( 'NONE', #92366, #20902 ) ;
#57755=ADVANCED_FACE ( 'NONE', ( #47022 ), #81147, .F. ) ;
#57761=DIRECTION ( 'NONE',  ( 0.000000000000000000, -1.000000000000000000, 6.123233995736769734E-17 ) ) ;
#57767=CARTESIAN_POINT ( 'NONE',  ( -4.584004161252830833, 1511.400228778165001, 200.7368584331096599 ) ) ;
#57772=CARTESIAN_POINT ( 'NONE',  ( 4.029572640705000985, 1516.858649670339901, 205.0803734583570019 ) ) ;
#57786=CARTESIAN_POINT ( 'NONE',  ( 1.718203463455000080, 1516.898441858519845, 210.8221056461869978 ) ) ;
#57797=ORIENTED_EDGE ( 'NONE', *, *, #180, .F. ) ;
#57806=CARTESIAN_POINT ( 'NONE',  ( 3.956111774270300696, 1516.693880335250014, 215.4951837019553977 ) ) ;
#57811=CARTESIAN_POINT ( 'NONE',  ( -0.01073133209419849937, 1516.939491476980038, 201.7897819926569980 ) ) ;
#57812=CARTESIAN_POINT ( 'NONE',  ( -2.493697079054999932, 1516.977201124959947, 208.0034927161370035 ) ) ;
#57813=ORIENTED_EDGE ( 'NONE', *, *, #45442, .F. ) ;
#57829=CARTESIAN_POINT ( 'NONE',  ( -3.259729335964999919, 1517.119374999550018, 216.4589997383470177 ) ) ;
#57832=CYLINDRICAL_SURFACE ( 'NONE', #71458, 1.000000000000070166 ) ;
#57834=CARTESIAN_POINT ( 'NONE',  ( 4.042417777704999438, 1516.904492006980036, 212.5700528489170154 ) ) ;
#57852=CARTESIAN_POINT ( 'NONE',  ( 7.710285837685000310, 1516.582197289609894, 205.8614676770269796 ) ) ;
#57872=CARTESIAN_POINT ( 'NONE',  ( -12.83553538817613671, 1513.363077551962306, 192.3415662781734454 ) ) ;
#57890=CARTESIAN_POINT ( 'NONE',  ( -15.12442022026499977, 1514.217947259989842, 194.2848590935669790 ) ) ;
#57895=CARTESIAN_POINT ( 'NONE',  ( -5.780232115465000042, 1516.760434454289907, 201.7950504087270076 ) ) ;
#57896=CARTESIAN_POINT ( 'NONE',  ( -8.793958255968036042, 1511.660055404817513, 215.2685923549327924 ) ) ;
#57898=CARTESIAN_POINT ( 'NONE',  ( 15.69395956763500166, 1511.900571936589813, 196.7363318035669977 ) ) ;
#57913=( BOUNDED_CURVE ( )  B_SPLINE_CURVE ( 3, ( #51870, #103339, #77072, #381 ),
 .UNSPECIFIED., .F., .T. ) 
 B_SPLINE_CURVE_WITH_KNOTS ( ( 4, 4 ),
 ( 0.5395807524033044977, 1.539014399147148771 ),
 .UNSPECIFIED. ) 
 CURVE ( )  GEOMETRIC_REPRESENTATION_ITEM ( )  RATIONAL_B_SPLINE_CURVE ( ( 1.000000000000000000, 0.9184788592065064039, 0.9184788592065064039, 1.000000000000000000 ) ) 
 REPRESENTATION_ITEM ( '' )  );
#57919=DIRECTION ( 'NONE',  ( 0.6742693640212139572, 4.521919481779822175E-17, 0.7384854939282339270 ) ) ;
#57932=CARTESIAN_POINT ( 'NONE',  ( 7.718763505904999711, 1516.905946377369901, 216.0642002436470079 ) ) ;
#57934=B_SPLINE_SURFACE_WITH_KNOTS ( 'NONE', 5, 5, ( 
 ( #99245, #56724, #62967, #90860, #14148, #48334 ),
 ( #82474, #39916, #28764, #108768, #100370, #16876 ),
 ( #91964, #7410, #85207, #15772, #7956, #99800 ),
 ( #66250, #48891, #49432, #83019, #49974, #51081 ),
 ( #15240, #41008, #76271, #74633, #92505, #24731 ),
 ( #23094, #8497, #25287, #23655, #101441, #109337 ) ),
 .UNSPECIFIED., .F., .F., .F.,
 ( 6, 6 ),
 ( 6, 6 ),
 ( 4.250940516431700011, 7.082035122218299783 ),
 ( -9.670478296250548992E-06, 0.5000000000000000000 ),
 .UNSPECIFIED. ) ;
#57939=ORIENTED_EDGE ( 'NONE', *, *, #65330, .T. ) ;
#57940=CARTESIAN_POINT ( 'NONE',  ( -2.879642191334999879, 1516.812046502680005, 205.6755161564470313 ) ) ;
#57942=CARTESIAN_POINT ( 'NONE',  ( -6.944466780504999548, 1516.939530130779985, 209.1331108864249870 ) ) ;
#57953=CARTESIAN_POINT ( 'NONE',  ( 2.296124850935000072, 1516.677239312369920, 213.7299927514870319 ) ) ;
#57957=CARTESIAN_POINT ( 'NONE',  ( -7.721293097101060710, 1517.002586324550066, 208.8777730749319801 ) ) ;
#57958=CARTESIAN_POINT ( 'NONE',  ( -4.610079871555000430, 1516.713079096360161, 210.2553629353369899 ) ) ;
#57971=CARTESIAN_POINT ( 'NONE',  ( 12.56945274703499926, 1512.044075975079977, 224.3812485392670055 ) ) ;
#57973=CARTESIAN_POINT ( 'NONE',  ( -6.554778571775000451, 1516.929962200689943, 216.8412383526069789 ) ) ;
#57978=CARTESIAN_POINT ( 'NONE',  ( 2.289624432225000117, 1517.154223579619838, 202.5582500624169882 ) ) ;
#57979=CARTESIAN_POINT ( 'NONE',  ( -16.65017492986500258, 1513.596256836690145, 223.2301996313669861 ) ) ;
#58000=CARTESIAN_POINT ( 'NONE',  ( -4.802243959118389860, 1508.551704408389924, 213.5515878908929892 ) ) ;
#58006=FACE_OUTER_BOUND ( 'NONE', #35818, .T. ) ;
#58054=CARTESIAN_POINT ( 'NONE',  ( 4.624736859184999993, 1516.994127245590107, 211.9896495963369887 ) ) ;
#58058=CARTESIAN_POINT ( 'NONE',  ( 4.622842844184999578, 1516.901952101700090, 213.1523604828169880 ) ) ;
#58066=CARTESIAN_POINT ( 'NONE',  ( 2.483322453895000059, 1517.139039350860003, 202.5585910412470128 ) ) ;
#58068=DIRECTION ( 'NONE',  ( -1.577721810442025012E-32, -1.000000000000000000, 6.123233995736769734E-17 ) ) ;
#58080=CARTESIAN_POINT ( 'NONE',  ( -6.933587693644999383, 1516.542957540330008, 210.8312046333570038 ) ) ;
#58086=CARTESIAN_POINT ( 'NONE',  ( 4.026614479655000522, 1516.699825673279975, 207.4075116849170115 ) ) ;
#58096=B_SPLINE_CURVE_WITH_KNOTS ( 'NONE', 3,
 ( #4584, #38717, #89134, #61755, #12960, #87495 ),
 .UNSPECIFIED., .F., .F.,
 ( 4, 2, 4 ),
 ( 0.000000000000000000, 0.5000000000000000000, 1.000000000000000000 ),
 .UNSPECIFIED. ) ;
#58102=CARTESIAN_POINT ( 'NONE',  ( -4.611879723454999969, 1516.858533673840157, 213.7437437946470027 ) ) ;
#58104=CARTESIAN_POINT ( 'NONE',  ( -7.508706911753730395, 1508.884207225577029, 214.6352815288312570 ) ) ;
#58105=CARTESIAN_POINT ( 'NONE',  ( -5.003220765204999587, 1516.983995446890049, 216.0685944891870065 ) ) ;
#58127=CARTESIAN_POINT ( 'NONE',  ( 9.500116199115000271, 1517.051704408389924, 195.7139841003669858 ) ) ;
#58135=CARTESIAN_POINT ( 'NONE',  ( -4.820945246504999560, 1510.984078637139874, 201.4521197723069861 ) ) ;
#58178=CARTESIAN_POINT ( 'NONE',  ( -7.724874651314999952, 1517.139320148880188, 208.3815253650730028 ) ) ;
#58186=CARTESIAN_POINT ( 'NONE',  ( -15.15436964682470133, 1512.305164330070056, 221.9485801204349968 ) ) ;
#58213=CARTESIAN_POINT ( 'NONE',  ( -0.01306004006829850073, 1516.939762005280045, 204.5032625402269844 ) ) ;
#58221=ADVANCED_FACE ( 'NONE', ( #76901 ), #94225, .T. ) ;
#58224=CARTESIAN_POINT ( 'NONE',  ( -12.72383577362860052, 1512.260118274579781, 194.0134362855580150 ) ) ;
#58301=CARTESIAN_POINT ( 'NONE',  ( -3.059258307290346313, 1511.948750846285975, 201.2117255214971294 ) ) ;
#58307=CARTESIAN_POINT ( 'NONE',  ( -4.624099329465000352, 1516.962555622980062, 205.8665050058069994 ) ) ;
#58316=CARTESIAN_POINT ( 'NONE',  ( -16.06220695246549113, 1512.836811624631537, 220.2343054163481781 ) ) ;
#58321=CARTESIAN_POINT ( 'NONE',  ( -4.608146819384999482, 1516.677239312369920, 211.4179708211670174 ) ) ;
#58327=PRODUCT_CONTEXT ( 'NONE', #70655, 'mechanical' ) ;
#58333=ORIENTED_EDGE ( 'NONE', *, *, #11251, .F. ) ;
#58343=CARTESIAN_POINT ( 'NONE',  ( 2.446740381308137646, 1516.554415856208834, 216.2144072986330343 ) ) ;
#58349=CARTESIAN_POINT ( 'NONE',  ( -1.129386240404999908, 1516.613712827999962, 201.7984555248870038 ) ) ;
#58350=CARTESIAN_POINT ( 'NONE',  ( 6.550870144104999682, 1516.727502608469877, 208.3674577492799926 ) ) ;
#58354=CARTESIAN_POINT ( 'NONE',  ( 4.433893130974031038, 1511.410080502447272, 217.4576852855098252 ) ) ;
#58370=CARTESIAN_POINT ( 'NONE',  ( 3.260378255074999565, 1516.582197289609894, 216.8321318079170226 ) ) ;
#58376=CARTESIAN_POINT ( 'NONE',  ( -7.711550716115000093, 1516.630499592039996, 213.1573366827869904 ) ) ;
#58394=CARTESIAN_POINT ( 'NONE',  ( 4.028307740155000261, 1516.797038924770050, 205.8554964580370097 ) ) ;
#58411=DIRECTION ( 'NONE',  ( 0.7071067811865490160, 0.000000000000000000, -0.7071067811865461294 ) ) ;
#58416=CARTESIAN_POINT ( 'NONE',  ( -13.24074056834217217, 1513.560729025362889, 192.3374869004694574 ) ) ;
#58431=CARTESIAN_POINT ( 'NONE',  ( -7.461942747583736768, 1510.835436364141515, 215.2999418035631152 ) ) ;
#58436=CARTESIAN_POINT ( 'NONE',  ( -6.616507082082380364, 1517.051706634759967, 205.3940390167639976 ) ) ;
#58440=CARTESIAN_POINT ( 'NONE',  ( -4.038637500854999729, 1516.734985836460055, 203.3481771172569950 ) ) ;
#58443=CARTESIAN_POINT ( 'NONE',  ( 15.38132086023500023, 1512.167884426309911, 196.2735975057670146 ) ) ;
#58477=AXIS2_PLACEMENT_3D ( 'NONE', #28751, #105461, #97066 ) ;
#58478=CARTESIAN_POINT ( 'NONE',  ( -3.259101837015000225, 1517.102359858469754, 216.0714209178769920 ) ) ;
#58479=CARTESIAN_POINT ( 'NONE',  ( -7.891777529692960869, 1512.314860027450095, 212.0638759934929851 ) ) ;
#58485=CARTESIAN_POINT ( 'NONE',  ( 2.478306819944999795, 1516.938330505699923, 205.6592251139969960 ) ) ;
#58487=CARTESIAN_POINT ( 'NONE',  ( 1.127928333405000094, 1516.989863902050047, 209.1117210464550169 ) ) ;
#58491=CARTESIAN_POINT ( 'NONE',  ( 7.779264690585000253, 1514.199187793469946, 215.8377718132869916 ) ) ;
#58501=CARTESIAN_POINT ( 'NONE',  ( 3.264778779384999829, 1516.727068157269969, 214.1190961241369735 ) ) ;
#58507=CARTESIAN_POINT ( 'NONE',  ( 2.881548424445000034, 1516.909589401870107, 211.4054166033970148 ) ) ;
#58524=DIRECTION ( 'NONE',  ( -0.7071067811865475727, 2.497298964526426743E-16, 0.7071067811865475727 ) ) ;
#58528=CARTESIAN_POINT ( 'NONE',  ( 6.939219482805000005, 1516.783701990830195, 203.3409846960470020 ) ) ;
#58546=ORIENTED_EDGE ( 'NONE', *, *, #78200, .T. ) ;
#58575=CYLINDRICAL_SURFACE ( 'NONE', #5375, 1.999999999999997335 ) ;
#58603=CARTESIAN_POINT ( 'NONE',  ( 4.329791490734999471, 1515.051704408389924, 212.4519801359869859 ) ) ;
#58605=CARTESIAN_POINT ( 'NONE',  ( 3.267291605165000057, 1516.842852731759876, 212.5687880419470162 ) ) ;
#58607=CARTESIAN_POINT ( 'NONE',  ( 5.110470188734999475, 1511.399604276809896, 217.3678244789069822 ) ) ;
#58612=CARTESIAN_POINT ( 'NONE',  ( 6.940473334145000450, 1516.833525648419936, 202.5658237375970145 ) ) ;
#58615=LINE ( 'NONE', #9306, #90975 ) ;
#58628=CARTESIAN_POINT ( 'NONE',  ( 2.881222757585000238, 1516.891731298979948, 211.5992195760969707 ) ) ;
#58633=CARTESIAN_POINT ( 'NONE',  ( 6.546001350565000543, 1516.557392317769882, 207.4118413833070065 ) ) ;
#58643=DIRECTION ( 'NONE',  ( -0.7044160264027579110, -0.08715574274766998975, 0.7044160264027579110 ) ) ;
#58648=CARTESIAN_POINT ( 'NONE',  ( -7.713117841115000317, 1516.690345681169902, 214.1262880092169780 ) ) ;
#58651=CARTESIAN_POINT ( 'NONE',  ( -5.778372601744999670, 1516.932669162149978, 216.0673360190369863 ) ) ;
#58654=ADVANCED_FACE ( 'NONE', ( #54627 ), #64124, .T. ) ;
#58658=ADVANCED_FACE ( 'NONE', ( #81425 ), #29382, .F. ) ;
#58671=EDGE_LOOP ( 'NONE', ( #95040, #60697, #107673, #97737, #100456, #93053, #34045, #96144 ) ) ;
#58725=CARTESIAN_POINT ( 'NONE',  ( -2.486220139904999904, 1516.939658295650133, 209.1350829839039989 ) ) ;
#58733=CARTESIAN_POINT ( 'NONE',  ( -14.95092673998889943, 1512.169469372310004, 221.5792698019450029 ) ) ;
#58758=CARTESIAN_POINT ( 'NONE',  ( -4.041472511874999896, 1516.858649670339901, 205.0922732913970208 ) ) ;
#58764=VERTEX_POINT ( 'NONE', #3675 ) ;
#58804=CARTESIAN_POINT ( 'NONE',  ( -1.569161292555000031, 1517.051704408389924, 216.8444262845069943 ) ) ;
#58848=CARTESIAN_POINT ( 'NONE',  ( 15.00522596485355287, 1511.839858410422266, 197.1933472413483912 ) ) ;
#58856=CARTESIAN_POINT ( 'NONE',  ( -1.715704529104999931, 1516.757508073510053, 205.8704515699670026 ) ) ;
#58857=AXIS2_PLACEMENT_3D ( 'NONE', #56965, #58068, #4884 ) ;
#58860=CARTESIAN_POINT ( 'NONE',  ( -16.87207556298167077, 1516.551188142742376, 195.8275909262277708 ) ) ;
#58870=CARTESIAN_POINT ( 'NONE',  ( -1.701027861004999808, 1516.937508036699910, 211.6166039682370013 ) ) ;
#58883=ORIENTED_EDGE ( 'NONE', *, *, #50103, .T. ) ;
#58892=CARTESIAN_POINT ( 'NONE',  ( 1.781283018236084148, 1516.548117337700205, 216.4089363120791347 ) ) ;
#58899=CARTESIAN_POINT ( 'NONE',  ( 2.871580388595000422, 1517.129577905929864, 202.1716309988170224 ) ) ;
#58900=CARTESIAN_POINT ( 'NONE',  ( 6.949703334655000120, 1517.130100026000036, 209.8609679372960102 ) ) ;
#58920=CARTESIAN_POINT ( 'NONE',  ( -3.454172653555000139, 1517.122088787240045, 216.8462693643270143 ) ) ;
#58922=VECTOR ( 'NONE', #60615, 1000.000000000000227 ) ;
#58925=CARTESIAN_POINT ( 'NONE',  ( -2.480187054844999572, 1517.025470194390209, 213.7472054950769973 ) ) ;
#58938=ADVANCED_FACE ( 'NONE', ( #49523 ), #91213, .F. ) ;
#58944=CARTESIAN_POINT ( 'NONE',  ( 2.478306819944999795, 1516.938330505699923, 205.6592251139969960 ) ) ;
#58986=CARTESIAN_POINT ( 'NONE',  ( -6.140127969266069741, 1508.880864730590019, 216.6292689825000082 ) ) ;
#58994=CARTESIAN_POINT ( 'NONE',  ( 8.181958942834999249, 1517.051704408389924, 212.1568108385370124 ) ) ;
#58998=CARTESIAN_POINT ( 'NONE',  ( -6.945490086935000029, 1516.932669162149978, 203.3434733684869968 ) ) ;
#59001=CARTESIAN_POINT ( 'NONE',  ( 16.46592301883499943, 1512.456207068040158, 197.3724380419670297 ) ) ;
#59008=ORIENTED_EDGE ( 'NONE', *, *, #23852, .F. ) ;
#59027=CARTESIAN_POINT ( 'NONE',  ( 6.055196916395000351, 1514.134513140259969, 201.4763673648269844 ) ) ;
#59037=CARTESIAN_POINT ( 'NONE',  ( 1.708720984574999768, 1516.531533746980131, 216.4430152012269843 ) ) ;
#59038=CARTESIAN_POINT ( 'NONE',  ( -8.609273301071175055, 1511.418042823250744, 214.3800210669276112 ) ) ;
#59044=CARTESIAN_POINT ( 'NONE',  ( 0.7353365397730019515, 1516.995911393979895, 206.2425275143270085 ) ) ;
#59047=AXIS2_PLACEMENT_3D ( 'NONE', #46775, #80907, #20422 ) ;
#59050=CARTESIAN_POINT ( 'NONE',  ( 7.643022747455000321, 1513.886778334019937, 216.1363302133069908 ) ) ;
#59058=CARTESIAN_POINT ( 'NONE',  ( 2.489617538345000103, 1516.665179208830068, 214.1178407578070164 ) ) ;
#59063=CARTESIAN_POINT ( 'NONE',  ( 7.725990161824999980, 1517.181921232829836, 211.6070516194370157 ) ) ;
#59081=CARTESIAN_POINT ( 'NONE',  ( -1.126138146715000010, 1517.208444099459939, 216.8485306577670144 ) ) ;
#59083=CARTESIAN_POINT ( 'NONE',  ( 2.956070248525000110, 1512.851027015570025, 217.0276636870669904 ) ) ;
#59086=CARTESIAN_POINT ( 'NONE',  ( -3.261635970955000019, 1516.613881697390070, 202.1867125516770045 ) ) ;
#59105=CARTESIAN_POINT ( 'NONE',  ( -3.958644675774470212, 1508.551704408389924, 214.1089269091330038 ) ) ;
#59112=DIRECTION ( 'NONE',  ( -0.4999999999998399058, 0.7071067811867739472, -0.4999999999998399058 ) ) ;
#59160=ORIENTED_EDGE ( 'NONE', *, *, #99298, .T. ) ;
#59169=CARTESIAN_POINT ( 'NONE',  ( -5.774609660074999873, 1516.777260590120022, 213.7418541773069762 ) ) ;
#59175=CARTESIAN_POINT ( 'NONE',  ( 7.715625202974999652, 1516.786099423779888, 202.5670817708370066 ) ) ;
#59188=CARTESIAN_POINT ( 'NONE',  ( -15.20279581456499862, 1516.814170398969964, 193.2119433744669834 ) ) ;
#59190=CARTESIAN_POINT ( 'NONE',  ( 0.01323701367210150005, 1516.939658295650133, 211.6080660720070341 ) ) ;
#59195=CARTESIAN_POINT ( 'NONE',  ( 3.447128460625000113, 1516.778853242349896, 207.9866608880570027 ) ) ;
#59197=LINE ( 'NONE', #109041, #88490 ) ;
#59210=CARTESIAN_POINT ( 'NONE',  ( -5.774609660074999873, 1516.777260590120022, 213.7418541773069762 ) ) ;
#59213=CARTESIAN_POINT ( 'NONE',  ( 6.554764161265000055, 1516.786099423779888, 216.8374711732070068 ) ) ;
#59248=VECTOR ( 'NONE', #67035, 1000.000000000000114 ) ;
#59295=CARTESIAN_POINT ( 'NONE',  ( -2.873919040654999701, 1516.940252185109784, 209.1351185066319829 ) ) ;
#59301=CIRCLE ( 'NONE', #93237, 1.000000000028000047 ) ;
#59306=CARTESIAN_POINT ( 'NONE',  ( -15.13723823385460143, 1513.497693043359959, 223.5461030115109793 ) ) ;
#59329=CARTESIAN_POINT ( 'NONE',  ( -6.561686461364999445, 1517.069378699710114, 205.6695567495270041 ) ) ;
#59332=CARTESIAN_POINT ( 'NONE',  ( 14.86025862469639947, 1514.013728164689837, 194.2524291478609939 ) ) ;
#59335=ORIENTED_EDGE ( 'NONE', *, *, #28798, .F. ) ;
#59378=CARTESIAN_POINT ( 'NONE',  ( -2.479246885834999858, 1516.983612918759945, 213.1658362778269691 ) ) ;
#59405=EDGE_CURVE ( 'NONE', #12190, #22497, #2522, .T. ) ;
#59414=DIRECTION ( 'NONE',  ( -1.000000000000000000, 0.000000000000000000, 0.000000000000000000 ) ) ;
#59417=CARTESIAN_POINT ( 'NONE',  ( -3.052975934615000053, 1516.551704408390151, 201.1191225673069880 ) ) ;
#59421=CARTESIAN_POINT ( 'NONE',  ( -2.493073867885000183, 1516.826109302209943, 206.2575198447970024 ) ) ;
#59429=CARTESIAN_POINT ( 'NONE',  ( -16.66011982862587715, 1513.969110094344160, 223.0773383146762114 ) ) ;
#59433=CARTESIAN_POINT ( 'NONE',  ( 6.950833530105000158, 1517.156142772249950, 211.6057959108269984 ) ) ;
#59448=ORIENTED_EDGE ( 'NONE', *, *, #98682, .F. ) ;
#59453=AXIS2_PLACEMENT_3D ( 'NONE', #16590, #68172, #60872 ) ;
#59462=CARTESIAN_POINT ( 'NONE',  ( 2.483949940595000516, 1517.156142772249950, 202.1710124019969896 ) ) ;
#59463=CARTESIAN_POINT ( 'NONE',  ( 3.460866170685000132, 1517.020847257979995, 209.8575449048190080 ) ) ;
#59466=CARTESIAN_POINT ( 'NONE',  ( 4.726342638545708574, 1511.395336166597417, 217.5537869467808605 ) ) ;
#59485=B_SPLINE_CURVE_WITH_KNOTS ( 'NONE', 3,
 ( #75154, #40424, #101404, #33120, #67308, #85177, #68414, #57806, #15739, #24696, #25808, #49940, #42089, #58343, #84623, #17398, #58892, #84078, #34228, #93025, #7919, #76238 ),
 .UNSPECIFIED., .F., .F.,
 ( 4, 2, 2, 2, 2, 2, 2, 2, 2, 2, 4 ),
 ( 0.000000000000000000, 0.2500000000000107137, 0.3750000000000233147, 0.4375000000000259237, 0.4687500000000261458, 0.5000000000000263123, 0.6250000000000224265, 0.6875000000000186517, 0.7500000000000148770, 0.8750000000000075495, 1.000000000000000000 ),
 .UNSPECIFIED. ) ;
#59501=CARTESIAN_POINT ( 'NONE',  ( 5.771797426184999580, 1516.647618671360078, 206.2459958378869942 ) ) ;
#59546=CARTESIAN_POINT ( 'NONE',  ( -7.331812124104999384, 1516.906641539930206, 202.5676945058570197 ) ) ;
#59572=CARTESIAN_POINT ( 'NONE',  ( 6.964055579694999665, 1512.881909847360021, 201.9408257871969852 ) ) ;
#59581=CARTESIAN_POINT ( 'NONE',  ( -1.710012758625000018, 1517.232977404109988, 216.8491730849570160 ) ) ;
#59582=CARTESIAN_POINT ( 'NONE',  ( -8.392728068336928970, 1511.399179795969530, 213.7293764352533287 ) ) ;
#59587=CARTESIAN_POINT ( 'NONE',  ( -5.787477032644999575, 1517.070197312179971, 206.2521524731670013 ) ) ;
#59593=CARTESIAN_POINT ( 'NONE',  ( 8.027449271465000535, 1514.605246816809768, 215.6121524902470128 ) ) ;
#59601=CARTESIAN_POINT ( 'NONE',  ( -4.612507312034999529, 1516.886345593249871, 214.1313240375470173 ) ) ;
#59604=CARTESIAN_POINT ( 'NONE',  ( 7.266080978071760121, 1509.032013615249980, 215.8915072422500145 ) ) ;
#59606=CARTESIAN_POINT ( 'NONE',  ( -1.118104767724999782, 1516.965971551240045, 211.4215139361070044 ) ) ;
#59618=CARTESIAN_POINT ( 'NONE',  ( -7.559673342214999536, 1510.830536680500245, 212.2954481221070182 ) ) ;
#59629=CARTESIAN_POINT ( 'NONE',  ( -1.130002532395000037, 1516.621991115350056, 202.1860446705670142 ) ) ;
#59652=CARTESIAN_POINT ( 'NONE',  ( -4.426499592775540393, 1508.728286212990042, 213.2816877793200092 ) ) ;
#59689=CARTESIAN_POINT ( 'NONE',  ( 7.541469341541871430, 1510.554407339950330, 203.3603459154996358 ) ) ;
#59710=CARTESIAN_POINT ( 'NONE',  ( 6.947377783174999877, 1517.009964551830080, 213.7374907746170152 ) ) ;
#59715=CARTESIAN_POINT ( 'NONE',  ( -0.7560907659159991079, 1516.770163853809890, 204.1215159365669933 ) ) ;
#59730=CARTESIAN_POINT ( 'NONE',  ( 5.013274961385000061, 1517.068517094990057, 211.4089302402969963 ) ) ;
#59736=CARTESIAN_POINT ( 'NONE',  ( -2.299668004004999933, 1516.965971551240045, 208.0037412025070012 ) ) ;
#59749=B_SPLINE_CURVE_WITH_KNOTS ( 'NONE', 5,
 ( #77678, #105089, #79342, #52492, #35116, #88288 ),
 .UNSPECIFIED., .F., .F.,
 ( 6, 6 ),
 ( 0.000000000000000000, 1.000000000000000000 ),
 .UNSPECIFIED. ) ;
#59754=CARTESIAN_POINT ( 'NONE',  ( -4.031142389804999837, 1516.929569650079884, 214.1322689334670031 ) ) ;
#59832=CARTESIAN_POINT ( 'NONE',  ( -7.683752594814639458, 1511.083508941950186, 214.8842481327019982 ) ) ;
#59838=CARTESIAN_POINT ( 'NONE',  ( -1.709766532154999963, 1516.959716008189844, 209.1345041580460133 ) ) ;
#59872=CARTESIAN_POINT ( 'NONE',  ( -5.011678876155000850, 1516.989560013210166, 205.8658785457569991 ) ) ;
#59930=CARTESIAN_POINT ( 'NONE',  ( -3.448206916814999801, 1516.904492006980036, 213.1642637479369853 ) ) ;
#59948=B_SPLINE_CURVE_WITH_KNOTS ( 'NONE', 3,
 ( #86400, #52822, #9688, #42200, #86952, #24809 ),
 .UNSPECIFIED., .F., .F.,
 ( 4, 2, 4 ),
 ( 0.000000000000000000, 0.5000000000000000000, 1.000000000000000000 ),
 .UNSPECIFIED. ) ;
#59972=CARTESIAN_POINT ( 'NONE',  ( 3.446329775655000205, 1516.812046502680005, 206.2422037788969931 ) ) ;
#59980=CARTESIAN_POINT ( 'NONE',  ( -16.52212295123237240, 1514.209381233995373, 223.4393621722829266 ) ) ;
#59985=CARTESIAN_POINT ( 'NONE',  ( 1.717084711415000076, 1516.819260244609950, 211.5980165671369946 ) ) ;
#60001=CARTESIAN_POINT ( 'NONE',  ( -15.84449006176500241, 1515.383078152259941, 195.2224200989670067 ) ) ;
#60011=CARTESIAN_POINT ( 'NONE',  ( 2.482067860225000366, 1517.099836525840146, 203.3337487049469985 ) ) ;
#60012=CARTESIAN_POINT ( 'NONE',  ( 0.7533003524100010395, 1516.992029636990083, 209.8620668306199946 ) ) ;
#60038=CARTESIAN_POINT ( 'NONE',  ( 1.114056763157479590, 1516.634548230098289, 216.8335026655383899 ) ) ;
#60045=EDGE_CURVE ( 'NONE', #97701, #88321, #19496, .T. ) ;
#60051=CARTESIAN_POINT ( 'NONE',  ( -15.19327425026499867, 1512.300546902530186, 221.9778556009669899 ) ) ;
#60056=EDGE_LOOP ( 'NONE', ( #62740, #46500, #4507, #74648 ) ) ;
#60057=CARTESIAN_POINT ( 'NONE',  ( -4.043990345725000601, 1516.983612918759945, 206.6425990843970055 ) ) ;
#60081=CARTESIAN_POINT ( 'NONE',  ( -12.24389445090430328, 1513.118416466450981, 192.4462725802613932 ) ) ;
#60098=CARTESIAN_POINT ( 'NONE',  ( 13.92686551478569967, 1517.051704405520013, 192.0624604828410043 ) ) ;
#60105=CARTESIAN_POINT ( 'NONE',  ( 6.550389432124999800, 1516.755758396839838, 204.1155163507169732 ) ) ;
#60107=CARTESIAN_POINT ( 'NONE',  ( 14.96231789283499936, 1514.242353506929931, 193.9066102308669883 ) ) ;
#60113=ORIENTED_EDGE ( 'NONE', *, *, #74024, .T. ) ;
#60128=CARTESIAN_POINT ( 'NONE',  ( 1.717084711415000076, 1516.819260244609950, 211.5980165671369946 ) ) ;
#60131=CARTESIAN_POINT ( 'NONE',  ( 7.532473168254999685, 1513.265135866630089, 201.8177576823970014 ) ) ;
#60138=CARTESIAN_POINT ( 'NONE',  ( 3.415238410854999795, 1511.801704408389924, 204.7069501962670017 ) ) ;
#60139=CARTESIAN_POINT ( 'NONE',  ( 2.291676273424999799, 1516.534976163889951, 216.4430396779769978 ) ) ;
#60140=CARTESIAN_POINT ( 'NONE',  ( -8.184208294724300004, 1511.478961034980102, 213.0871669047343175 ) ) ;
#60145=CARTESIAN_POINT ( 'NONE',  ( 7.709681268295000223, 1516.559109716219837, 206.2491454149069909 ) ) ;
#60151=CARTESIAN_POINT ( 'NONE',  ( 7.891962413025000345, 1514.771170611759999, 215.1394100340270086 ) ) ;
#60160=CARTESIAN_POINT ( 'NONE',  ( 5.781490544344999982, 1516.807958722750072, 215.6734893570070142 ) ) ;
#60163=CARTESIAN_POINT ( 'NONE',  ( 6.089577284407799773, 1511.778877376279979, 217.5949564134380125 ) ) ;
#60165=ADVANCED_FACE ( 'NONE', ( #107367 ), #48326, .T. ) ;
#60167=CARTESIAN_POINT ( 'NONE',  ( -0.7350232362959980836, 1516.970035769810011, 211.4194755912870107 ) ) ;
#60177=CARTESIAN_POINT ( 'NONE',  ( -7.548872338225000256, 1510.418062979269962, 214.3032561208869993 ) ) ;
#60186=CARTESIAN_POINT ( 'NONE',  ( 2.867803626105000170, 1516.994127245590107, 204.4971090729170271 ) ) ;
#60203=CARTESIAN_POINT ( 'NONE',  ( -4.429773136856780091, 1508.551704408389924, 213.9240780803189921 ) ) ;
#60223=CARTESIAN_POINT ( 'NONE',  ( 7.170479361814977359, 1516.544351102706287, 206.9184616573184314 ) ) ;
#60260=CARTESIAN_POINT ( 'NONE',  ( 5.008848199894999631, 1516.858456333729919, 214.1219297979669989 ) ) ;
#60267=CARTESIAN_POINT ( 'NONE',  ( -6.559168674874999105, 1516.960844870249957, 204.1192525727769862 ) ) ;
#60281=CARTESIAN_POINT ( 'NONE',  ( -1.118903308544999975, 1517.003078582959688, 212.0031713441969998 ) ) ;
#60286=CARTESIAN_POINT ( 'NONE',  ( -2.491655763544999846, 1516.977504706749869, 208.3867361609839861 ) ) ;
#60296=EDGE_CURVE ( 'NONE', #90411, #100324, #44840, .T. ) ;
#60302=CARTESIAN_POINT ( 'NONE',  ( -7.712490991114999694, 1516.666407245520077, 213.7387074786470009 ) ) ;
#60306=VECTOR ( 'NONE', #84094, 1000.000000000000114 ) ;
#60308=CARTESIAN_POINT ( 'NONE',  ( 7.718949774015209542, 1516.913059669559971, 209.0472627469650035 ) ) ;
#60320=CARTESIAN_POINT ( 'NONE',  ( -5.385523200472070116, 1511.435001055929888, 200.4690698413500058 ) ) ;
#60342=CARTESIAN_POINT ( 'NONE',  ( -1.695768267810110030, 1516.547466091170008, 201.4124695628590018 ) ) ;
#60389=VERTEX_POINT ( 'NONE', #62207 ) ;
#60390=CARTESIAN_POINT ( 'NONE',  ( 2.491655725414999800, 1516.977504706749869, 209.8569557413499922 ) ) ;
#60395=EDGE_CURVE ( 'NONE', #71004, #39998, #45611, .T. ) ;
#60400=CARTESIAN_POINT ( 'NONE',  ( -15.21580404780189966, 1513.293387712810045, 223.3414678796779924 ) ) ;
#60409=CARTESIAN_POINT ( 'NONE',  ( 6.548200587644999793, 1516.632821972880038, 207.9912384682270101 ) ) ;
#60427=CARTESIAN_POINT ( 'NONE',  ( -7.724732447025000504, 1517.133889586189980, 205.8614888033369823 ) ) ;
#60430=CARTESIAN_POINT ( 'NONE',  ( -6.186741296575624993, 1516.987734611996530, 204.8208301658942219 ) ) ;
#60432=ORIENTED_EDGE ( 'NONE', *, *, #42532, .F. ) ;
#60477=CARTESIAN_POINT ( 'NONE',  ( -6.547881413045000265, 1516.647534046129977, 212.5778533554070293 ) ) ;
#60524=CARTESIAN_POINT ( 'NONE',  ( 4.026777485955000735, 1516.718889242609976, 206.8247602162870180 ) ) ;
#60525=AXIS2_PLACEMENT_3D ( 'NONE', #15002, #75508, #49201 ) ;
#60530=ORIENTED_EDGE ( 'NONE', *, *, #96732, .F. ) ;
#60535=CARTESIAN_POINT ( 'NONE',  ( -16.53526713099472900, 1514.188985850001018, 223.4099743505789490 ) ) ;
#60539=CARTESIAN_POINT ( 'NONE',  ( -2.863787893864999656, 1516.788317650260069, 210.8382387120070121 ) ) ;
#60542=AXIS2_PLACEMENT_3D ( 'NONE', #27882, #45811, #19464 ) ;
#60565=CARTESIAN_POINT ( 'NONE',  ( 6.648384424976800489, 1508.610125760119899, 202.0257673391629964 ) ) ;
#60570=CARTESIAN_POINT ( 'NONE',  ( 2.870951667784999994, 1517.111322026010157, 202.5592101095969895 ) ) ;
#60571=CARTESIAN_POINT ( 'NONE',  ( -1.704170752255000032, 1516.927039499179955, 209.8797722570040207 ) ) ;
#60574=CARTESIAN_POINT ( 'NONE',  ( 3.864344981488097908, 1511.505229895790080, 217.2740327373093976 ) ) ;
#60607=CARTESIAN_POINT ( 'NONE',  ( -15.62010811736499782, 1514.600163677630007, 224.4888522828669863 ) ) ;
#60612=CARTESIAN_POINT ( 'NONE',  ( 4.608146781254999880, 1516.677239312369920, 206.8257210811669893 ) ) ;
#60615=DIRECTION ( 'NONE',  ( -0.02616798426619638615, -0.9993150019883495494, -0.02616798426453448637 ) ) ;
#60630=CARTESIAN_POINT ( 'NONE',  ( -2.996785070334999634, 1512.020737142380085, 201.2284348500070053 ) ) ;
#60663=CARTESIAN_POINT ( 'NONE',  ( -2.875850132345000087, 1516.647618671360078, 203.3500485059169876 ) ) ;
#60686=STYLED_ITEM ( 'NONE', ( #39832 ), #11085 ) ;
#60690=CARTESIAN_POINT ( 'NONE',  ( -7.321193745875000047, 1516.534976163889951, 211.4135222436570132 ) ) ;
#60693=CARTESIAN_POINT ( 'NONE',  ( 5.919280288264999079, 1513.965983108850196, 201.4800680737670007 ) ) ;
#60697=ORIENTED_EDGE ( 'NONE', *, *, #21983, .T. ) ;
#60699=CARTESIAN_POINT ( 'NONE',  ( -7.532473206385000175, 1513.265135866640094, 216.4259342199370053 ) ) ;
#60700=CARTESIAN_POINT ( 'NONE',  ( 16.50477753120586755, 1512.979858876954040, 197.3152680210698122 ) ) ;
#60702=CARTESIAN_POINT ( 'NONE',  ( -5.003848160104999998, 1517.005755693489846, 216.4561742428970206 ) ) ;
#60713=CARTESIAN_POINT ( 'NONE',  ( 0.7351097711180020200, 1516.977504706749869, 206.6301902066870184 ) ) ;
#60718=CARTESIAN_POINT ( 'NONE',  ( -5.513225751105480299, 1508.611141565010030, 201.8002151886680053 ) ) ;
#60729=AXIS2_PLACEMENT_3D ( 'NONE', #61553, #49427, #83549 ) ;
#60731=CARTESIAN_POINT ( 'NONE',  ( 2.488360629304999794, 1516.616791731099966, 214.8929950451170043 ) ) ;
#60735=CARTESIAN_POINT ( 'NONE',  ( 2.881222757585000238, 1516.891731298979948, 211.5992195760969707 ) ) ;
#60751=CARTESIAN_POINT ( 'NONE',  ( -4.620008245204999753, 1516.777260590120022, 203.3472363101570011 ) ) ;
#60768=CIRCLE ( 'NONE', #92935, 0.9999999999999972244 ) ;
#60791=CARTESIAN_POINT ( 'NONE',  ( 7.500396670941167798, 1516.934665496271919, 209.1219157010845322 ) ) ;
#60808=CARTESIAN_POINT ( 'NONE',  ( 7.461942709067347579, 1510.835436365588748, 202.9437500974225657 ) ) ;
#60826=B_SPLINE_SURFACE_WITH_KNOTS ( 'NONE', 5, 5, ( 
 ( #16998, #6982, #7535, #108893, #32186, #110547 ),
 ( #41133, #102133, #50109, #67467, #75314, #76394 ),
 ( #101572, #25412, #84234, #66370, #269, #59604 ),
 ( #50649, #66916, #32736, #84780, #41691, #8625 ),
 ( #8076, #100489, #68570, #75850, #42247, #93721 ),
 ( #51198, #85328, #17562, #42800, #76960, #101025 ) ),
 .UNSPECIFIED., .F., .F., .F.,
 ( 6, 6 ),
 ( 6, 6 ),
 ( 5.893388896115880016, 9.819930328984119328 ),
 ( -0.0002947352041177890396, 0.5000000000000000000 ),
 .UNSPECIFIED. ) ;
#60831=CARTESIAN_POINT ( 'NONE',  ( -6.548821979184999975, 1516.688761843659904, 213.1592242262869945 ) ) ;
#60836=CARTESIAN_POINT ( 'NONE',  ( -2.294209667535000108, 1516.603620185149794, 203.3509623682169831 ) ) ;
#60853=CARTESIAN_POINT ( 'NONE',  ( 2.880592928985000079, 1516.859514182039902, 211.9868180862470126 ) ) ;
#60858=SHAPE_REPRESENTATION ( 'Cutting Blade', ( #21632 ), #78983 ) ;
#60859=CARTESIAN_POINT ( 'NONE',  ( 1.122033391945000069, 1516.972341476009888, 208.3659064338399673 ) ) ;
#60872=DIRECTION ( 'NONE',  ( 1.000000000000000000, 0.000000000000000000, 0.000000000000000000 ) ) ;
#60874=CARTESIAN_POINT ( 'NONE',  ( -1.706797824074999914, 1517.164987839469859, 214.9112406324369999 ) ) ;
#60877=CARTESIAN_POINT ( 'NONE',  ( -6.941727290454999810, 1516.882217593000178, 216.4530290611770056 ) ) ;
#60879=CARTESIAN_POINT ( 'NONE',  ( 1.126138108584999964, 1517.208444099459939, 201.3951612445669923 ) ) ;
#60946=EDGE_CURVE ( 'NONE', #60389, #89576, #18775, .T. ) ;
#60956=CARTESIAN_POINT ( 'NONE',  ( 3.269025135755000200, 1517.026534522949987, 210.2412850599169758 ) ) ;
#60958=LINE ( 'NONE', #95084, #26936 ) ;
#60965=CARTESIAN_POINT ( 'NONE',  ( -15.31239857737409871, 1512.759354980449871, 222.7072629143739846 ) ) ;
#60967=VECTOR ( 'NONE', #27529, 999.9999999999998863 ) ;
#60973=CARTESIAN_POINT ( 'NONE',  ( -4.042388539304999640, 1517.045004075700035, 208.3857484934819979 ) ) ;
#60989=CARTESIAN_POINT ( 'NONE',  ( -2.879956963085000154, 1516.827328999679821, 205.8693153165069702 ) ) ;
#60990=ORIENTED_EDGE ( 'NONE', *, *, #18594, .F. ) ;
#61010=CARTESIAN_POINT ( 'NONE',  ( 5.784638319815000429, 1516.939574742129935, 213.7356083271170064 ) ) ;
#61021=ADVANCED_FACE ( 'NONE', ( #52983 ), #50159, .F. ) ;
#61043=CARTESIAN_POINT ( 'NONE',  ( -1.119717754394999876, 1517.038650117239968, 212.5846815975970117 ) ) ;
#61052=DIRECTION ( 'NONE',  ( 0.7063774289747313251, 0.04540766091858271930, -0.7063774289747313251 ) ) ;
#61062=( NAMED_UNIT ( * ) PLANE_ANGLE_UNIT ( ) SI_UNIT ( $, .RADIAN. ) );
#61087=CARTESIAN_POINT ( 'NONE',  ( -7.068319539573729493, 1516.559613835828259, 211.6298318704503174 ) ) ;
#61092=CARTESIAN_POINT ( 'NONE',  ( 0.7350231981660010350, 1516.970035769810011, 206.8242163110469960 ) ) ;
#61099=FACE_OUTER_BOUND ( 'NONE', #72033, .T. ) ;
#61104=CARTESIAN_POINT ( 'NONE',  ( 7.337153768115000751, 1517.119374999550018, 212.3815752680669959 ) ) ;
#61106=AXIS2_PLACEMENT_3D ( 'NONE', #88791, #38373, #64719 ) ;
#61129=CARTESIAN_POINT ( 'NONE',  ( 6.032863516324240116, 1508.551565390750284, 201.9555854317009960 ) ) ;
#61134=CARTESIAN_POINT ( 'NONE',  ( 3.451033388965000004, 1517.025653221279981, 203.3353183697670090 ) ) ;
#61135=CARTESIAN_POINT ( 'NONE',  ( 3.455495833855000143, 1516.939877939420057, 209.1085718841020196 ) ) ;
#61140=CARTESIAN_POINT ( 'NONE',  ( 5.399591216012582962, 1511.369014876942174, 217.1050657725866415 ) ) ;
#61157=CARTESIAN_POINT ( 'NONE',  ( -6.088832748515000226, 1511.778199792620171, 200.6487770440270140 ) ) ;
#61175=CARTESIAN_POINT ( 'NONE',  ( -14.96231793096499985, 1514.242353506929931, 224.3370816714669900 ) ) ;
#61180=CARTESIAN_POINT ( 'NONE',  ( -3.268235758764999943, 1516.890356958860139, 206.2562572478169898 ) ) ;
#61196=CARTESIAN_POINT ( 'NONE',  ( -2.942029669205000086, 1512.314860029340025, 201.2300684455470048 ) ) ;
#61225=CARTESIAN_POINT ( 'NONE',  ( 14.28619591199671390, 1517.015067828388510, 192.2953432750010165 ) ) ;
#61232=CARTESIAN_POINT ( 'NONE',  ( -2.489617576474999705, 1516.665179208830068, 204.1258511445269903 ) ) ;
#61242=ORIENTED_EDGE ( 'NONE', *, *, #3502, .T. ) ;
#61255=CARTESIAN_POINT ( 'NONE',  ( -3.251888867474999945, 1516.793978928989873, 211.6142896211370044 ) ) ;
#61258=CARTESIAN_POINT ( 'NONE',  ( 7.263042179585000646, 1512.240414293140020, 202.3122947996570247 ) ) ;
#61265=CARTESIAN_POINT ( 'NONE',  ( -8.191860474865000796, 1512.696049264750172, 216.1202668200969867 ) ) ;
#61269=CARTESIAN_POINT ( 'NONE',  ( -7.717505791104999346, 1516.857914730730045, 216.8393517232070167 ) ) ;
#61276=CARTESIAN_POINT ( 'NONE',  ( 5.771149074885000729, 1516.616791731099966, 206.6334853027970269 ) ) ;
#61281=EDGE_LOOP ( 'NONE', ( #69550, #14344, #67630, #12609 ) ) ;
#61292=CARTESIAN_POINT ( 'NONE',  ( 7.331812085974999782, 1516.906641539930206, 215.6759973964769870 ) ) ;
#61294=CARTESIAN_POINT ( 'NONE',  ( 6.170974574032440430, 1511.326458810320219, 216.6586639964210121 ) ) ;
#61296=CARTESIAN_POINT ( 'NONE',  ( -0.7355686809059980291, 1517.012231669750008, 212.3888856620870058 ) ) ;
#61314=CARTESIAN_POINT ( 'NONE',  ( -5.008848238024999233, 1516.858456333729919, 204.1217621043670079 ) ) ;
#61337=DIRECTION ( 'NONE',  ( 0.9147450530333530727, 0.03449475076686789321, -0.4025563316115395862 ) ) ;
#61344=EDGE_LOOP ( 'NONE', ( #41103, #79925, #51095, #56931, #57580, #43588 ) ) ;
#61349=CARTESIAN_POINT ( 'NONE',  ( 6.564931535518120143, 1516.660079020903368, 205.4906681412120406 ) ) ;
#61355=CARTESIAN_POINT ( 'NONE',  ( -5.779603138255000161, 1516.738222552470233, 201.4074744291170020 ) ) ;
#61363=EDGE_LOOP ( 'NONE', ( #52975, #83784, #10599, #57797, #34472, #56563, #59335, #9949, #70874 ) ) ;
#61364=CARTESIAN_POINT ( 'NONE',  ( 7.481780845334932373, 1510.769285165366227, 203.0163852401010729 ) ) ;
#61384=CARTESIAN_POINT ( 'NONE',  ( -2.286446363765000100, 1517.042661899400173, 213.7475398352470108 ) ) ;
#61385=CARTESIAN_POINT ( 'NONE',  ( 3.991161783265000818, 1511.207707629420156, 216.9064051716169956 ) ) ;
#61390=CARTESIAN_POINT ( 'NONE',  ( -2.488360667435000284, 1516.616791731099966, 203.3506968572170308 ) ) ;
#61392=CARTESIAN_POINT ( 'NONE',  ( -5.181410188784999704, 1510.418062979269962, 201.5729736320070060 ) ) ;
#61397=CARTESIAN_POINT ( 'NONE',  ( -12.07722023368130593, 1511.957228877181251, 194.2728863314506214 ) ) ;
#61400=FACE_OUTER_BOUND ( 'NONE', #23002, .T. ) ;
#61403=CARTESIAN_POINT ( 'NONE',  ( 7.725372132234999967, 1517.158319634930194, 211.9946825927569876 ) ) ;
#61408=CARTESIAN_POINT ( 'NONE',  ( -2.879318455905000018, 1516.995911393979895, 208.3865093923290033 ) ) ;
#61423=CARTESIAN_POINT ( 'NONE',  ( 1.711311228545000063, 1516.591755933730155, 214.8926661113670207 ) ) ;
#61426=CARTESIAN_POINT ( 'NONE',  ( 1.128757561074999805, 1516.608208975040043, 216.8328129478670121 ) ) ;
#61428=CARTESIAN_POINT ( 'NONE',  ( 4.035536225084999984, 1517.086065052259983, 201.3983658527070020 ) ) ;
#61434=CARTESIAN_POINT ( 'NONE',  ( 8.792772900901731248, 1511.562335007999991, 203.1497331793660237 ) ) ;
#61488=FACE_OUTER_BOUND ( 'NONE', #23546, .T. ) ;
#61503=CARTESIAN_POINT ( 'NONE',  ( 0.7559394982620020187, 1516.972341476009888, 210.2438793621770117 ) ) ;
#61504=CARTESIAN_POINT ( 'NONE',  ( 6.391938807520832988, 1508.551704408389696, 202.1089244633390365 ) ) ;
#61506=DIRECTION ( 'NONE',  ( -0.02616798426453448984, -0.9993150019883495494, 0.02616798426619649023 ) ) ;
#61521=CARTESIAN_POINT ( 'NONE',  ( -4.044319925355000400, 1517.073005577650065, 208.0013022344469960 ) ) ;
#61536=CARTESIAN_POINT ( 'NONE',  ( -0.01327408612949850138, 1516.939877939420057, 205.6663500982469941 ) ) ;
#61538=CARTESIAN_POINT ( 'NONE',  ( 5.649719750514999639, 1514.243099272629934, 201.4728115316369781 ) ) ;
#61546=CARTESIAN_POINT ( 'NONE',  ( 6.805044835120149571, 1517.051704409849890, 212.9954169445540231 ) ) ;
#61553=CARTESIAN_POINT ( 'NONE',  ( -7.500000019064999357, 1508.551704408389924, 209.1218459511669892 ) ) ;
#61555=CARTESIAN_POINT ( 'NONE',  ( -3.255340964424999761, 1516.962555622980062, 213.7459452615670159 ) ) ;
#61556=DIRECTION ( 'NONE',  ( 0.000000000000000000, -1.000000000000000000, 0.000000000000000000 ) ) ;
#61569=FACE_OUTER_BOUND ( 'NONE', #11487, .T. ) ;
#61573=CARTESIAN_POINT ( 'NONE',  ( 11.75704293633499908, 1511.932705841380084, 199.9008530307569913 ) ) ;
#61574=CARTESIAN_POINT ( 'NONE',  ( -7.460636413916523324, 1509.035273822891668, 203.0850875598481196 ) ) ;
#61582=CARTESIAN_POINT ( 'NONE',  ( -3.447264387095000160, 1516.858765657450249, 212.5828932618570093 ) ) ;
#61608=DIRECTION ( 'NONE',  ( 0.000000000000000000, -1.000000000000000000, 0.000000000000000000 ) ) ;
#61609=VERTEX_POINT ( 'NONE', #31892 ) ;
#61620=CARTESIAN_POINT ( 'NONE',  ( -4.148213077643431390, 1517.003210141817590, 215.3943059606615122 ) ) ;
#61623=CARTESIAN_POINT ( 'NONE',  ( -8.756942758513574177, 1511.516807858200764, 214.9135418063871725 ) ) ;
#61625=CARTESIAN_POINT ( 'NONE',  ( 5.770883563884999568, 1516.603620185149794, 206.8276363026970159 ) ) ;
#61640=CARTESIAN_POINT ( 'NONE',  ( -3.251888867474999945, 1516.793978928989873, 211.6142896211370044 ) ) ;
#61646=EDGE_CURVE ( 'NONE', #19916, #68294, #27915, .T. ) ;
#61666=CARTESIAN_POINT ( 'NONE',  ( 6.141397696570729536, 1509.034509440879901, 201.6091292273739839 ) ) ;
#61672=CARTESIAN_POINT ( 'NONE',  ( 4.032397901875000024, 1516.981965530290154, 203.3362630185569913 ) ) ;
#61673=CARTESIAN_POINT ( 'NONE',  ( -7.323390445344999833, 1516.613712827999962, 210.2512321725070024 ) ) ;
#61708=DIRECTION ( 'NONE',  ( -0.9980919085851078787, 0.06174578541841399537, 0.000000000000000000 ) ) ;
#61709=CARTESIAN_POINT ( 'NONE',  ( 12.61087482253499914, 1512.195694528090144, 224.2019839780669770 ) ) ;
#61718=CARTESIAN_POINT ( 'NONE',  ( -3.461995196814999787, 1516.906233342200039, 206.2559344154570056 ) ) ;
#61735=CARTESIAN_POINT ( 'NONE',  ( 5.671687374334005938, 1510.518062812720245, 216.6698829330774458 ) ) ;
#61755=CARTESIAN_POINT ( 'NONE',  ( 3.487592429898332291, 1508.783371651612924, 204.5758637223170808 ) ) ;
#61770=CARTESIAN_POINT ( 'NONE',  ( -4.621897862544999569, 1516.858533673840157, 204.5099662467769974 ) ) ;
#61773=EDGE_CURVE ( 'NONE', #68158, #107607, #25876, .T. ) ;
#61780=ORIENTED_EDGE ( 'NONE', *, *, #107789, .T. ) ;
#61786=EDGE_CURVE ( 'NONE', #93671, #51820, #4379, .T. ) ;
#61796=CARTESIAN_POINT ( 'NONE',  ( -7.710285875814999912, 1516.582197289609894, 212.3822242253069987 ) ) ;
#61818=CARTESIAN_POINT ( 'NONE',  ( -1.717432486395000124, 1516.836638729160086, 206.8395443540670158 ) ) ;
#61832=CARTESIAN_POINT ( 'NONE',  ( 16.67046851633390148, 1516.551188146170034, 222.1952932998519827 ) ) ;
#61837=CARTESIAN_POINT ( 'NONE',  ( -1.706797824074999914, 1517.164987839469859, 214.9112406324369999 ) ) ;
#61840=CARTESIAN_POINT ( 'NONE',  ( 5.495614718128320142, 1510.802068165409992, 216.7138213142690120 ) ) ;
#61842=CARTESIAN_POINT ( 'NONE',  ( 4.042729802795000715, 1516.919782530640077, 212.3762473738369749 ) ) ;
#61844=CARTESIAN_POINT ( 'NONE',  ( 4.329791490734999471, 1515.051704408389924, 212.4519801359869859 ) ) ;
#61858=EDGE_LOOP ( 'NONE', ( #60530, #75097, #58333, #4070 ) ) ;
#61859=CARTESIAN_POINT ( 'NONE',  ( 0.7369041709050019318, 1517.080322339569875, 204.1102945640870132 ) ) ;
#61878=ADVANCED_FACE ( 'NONE', ( #32324 ), #824, .F. ) ;
#61889=CARTESIAN_POINT ( 'NONE',  ( 7.889086915934699462, 1512.111360402248920, 206.1534947800682289 ) ) ;
#61907=CARTESIAN_POINT ( 'NONE',  ( 7.891777486555000110, 1512.314860029340025, 206.1798163010270173 ) ) ;
#61911=ORIENTED_EDGE ( 'NONE', *, *, #18926, .F. ) ;
#61918=CARTESIAN_POINT ( 'NONE',  ( -7.784559239514999618, 1511.207707629420156, 213.1130077534970155 ) ) ;
#61921=EDGE_CURVE ( 'NONE', #43145, #29266, #59197, .T. ) ;
#61938=CARTESIAN_POINT ( 'NONE',  ( -5.000083865865000199, 1516.858456333729919, 214.1306941701269864 ) ) ;
#61939=CARTESIAN_POINT ( 'NONE',  ( 4.427981723884999887, 1510.423579818969984, 216.6708627338570068 ) ) ;
#61946=CARTESIAN_POINT ( 'NONE',  ( 7.713117802984999827, 1516.690345681169902, 204.1174038931170003 ) ) ;
#61961=CARTESIAN_POINT ( 'NONE',  ( -4.608417544644999531, 1516.691389976299888, 211.6120918846570191 ) ) ;
#61966=CARTESIAN_POINT ( 'NONE',  ( 1.709766494024999917, 1516.959716008189844, 209.1091877442879934 ) ) ;
#61973=PLANE ( 'NONE',  #88910 ) ;
#61979=CARTESIAN_POINT ( 'NONE',  ( 4.037378256055000669, 1516.688761843659904, 215.6706679112870120 ) ) ;
#61990=CARTESIAN_POINT ( 'NONE',  ( 7.936754916012690231, 1511.432897564909808, 203.2990511617569780 ) ) ;
#62000=DIRECTION ( 'NONE',  ( -0.7063774289747313251, 0.04540766091858271930, -0.7063774289747313251 ) ) ;
#62016=CARTESIAN_POINT ( 'NONE',  ( -1.730531345579879865, 1516.544444245470004, 201.4125486926729991 ) ) ;
#62061=CARTESIAN_POINT ( 'NONE',  ( -2.477975353594999763, 1516.839862955080207, 210.2583935552169976 ) ) ;
#62078=CARTESIAN_POINT ( 'NONE',  ( 7.710966977635000497, 1516.608208975040043, 207.9930883710269711 ) ) ;
#62085=CARTESIAN_POINT ( 'NONE',  ( 8.710714953028380947, 1511.457792576163911, 203.5654966221206905 ) ) ;
#62088=CIRCLE ( 'NONE', #22695, 1.000004583512053902 ) ;
#62095=CARTESIAN_POINT ( 'NONE',  ( 7.708770007014999592, 1516.524310051880093, 206.8307984429870032 ) ) ;
#62114=CARTESIAN_POINT ( 'NONE',  ( 3.265407117845000151, 1516.754149861460064, 213.7315192116670062 ) ) ;
#62132=DIRECTION ( 'NONE',  ( 0.000000000000000000, -0.02617694830808806397, 0.9996573249755517088 ) ) ;
#62155=CARTESIAN_POINT ( 'NONE',  ( -15.55634920516500053, 1516.551704408390151, 224.6781951372670108 ) ) ;
#62170=ORIENTED_EDGE ( 'NONE', *, *, #107452, .F. ) ;
#62180=CARTESIAN_POINT ( 'NONE',  ( -6.003502551534990239, 1516.754677662452423, 213.6177932582572794 ) ) ;
#62184=CARTESIAN_POINT ( 'NONE',  ( -6.951175166914999259, 1517.170721208160103, 206.8315896683770063 ) ) ;
#62197=CARTESIAN_POINT ( 'NONE',  ( -6.546302780145000000, 1516.577434278289957, 211.6089493897669911 ) ) ;
#62203=DIRECTION ( 'NONE',  ( -0.9980919085851078787, -0.06174578541841399537, 0.000000000000000000 ) ) ;
#62207=CARTESIAN_POINT ( 'NONE',  ( 4.487249753806469954, 1509.038615938009798, 205.6342535008409982 ) ) ;
#62220=CARTESIAN_POINT ( 'NONE',  ( 5.513207778675930371, 1508.731180391300086, 201.6768823099739905 ) ) ;
#62226=CARTESIAN_POINT ( 'NONE',  ( -6.556022232634999725, 1516.833525648419936, 202.1813725979570222 ) ) ;
#62227=CARTESIAN_POINT ( 'NONE',  ( -4.612671377915000370, 1516.783665406140017, 209.8782801844560026 ) ) ;
#62230=CARTESIAN_POINT ( 'NONE',  ( 5.381311896276537610, 1511.468585895425122, 217.4468093684960763 ) ) ;
#62231=ORIENTED_EDGE ( 'NONE', *, *, #27476, .F. ) ;
#62248=CARTESIAN_POINT ( 'NONE',  ( -7.181020183025000669, 1512.881909847350016, 202.1577903523970008 ) ) ;
#62262=CARTESIAN_POINT ( 'NONE',  ( 15.12442018213500106, 1514.217947259989842, 223.9588328087669993 ) ) ;
#62271=CARTESIAN_POINT ( 'NONE',  ( 6.933879402874999265, 1516.560253536979872, 206.6353711893569880 ) ) ;
#62291=CARTESIAN_POINT ( 'NONE',  ( 5.773315218126072068, 1510.559702728265165, 216.6621837239362947 ) ) ;
#62328=CARTESIAN_POINT ( 'NONE',  ( 5.773668814845000163, 1516.734985836460055, 205.0832084693769843 ) ) ;
#62344=B_SPLINE_CURVE_WITH_KNOTS ( 'NONE', 5,
 ( #76506, #110656, #33949, #68143, #93842, #79283, #104467, #61397, #45699 ),
 .UNSPECIFIED., .F., .F.,
 ( 6, 3, 6 ),
 ( 0.000000000000000000, 0.5000000000000000000, 1.000000000000000000 ),
 .UNSPECIFIED. ) ;
#62349=CARTESIAN_POINT ( 'NONE',  ( 0.01328393942530149870, 1516.939580991450157, 212.3834982571270018 ) ) ;
#62360=CARTESIAN_POINT ( 'NONE',  ( 16.78936285056073885, 1513.473960732874730, 196.0527388798289223 ) ) ;
#62369=CARTESIAN_POINT ( 'NONE',  ( 2.282622912365000367, 1516.861367446839949, 206.8218623544969716 ) ) ;
#62388=CARTESIAN_POINT ( 'NONE',  ( 6.556022194504999234, 1516.833525648419936, 216.0623193043769845 ) ) ;
#62391=CARTESIAN_POINT ( 'NONE',  ( 5.385694280313019000, 1511.434991102970116, 217.4429023633459792 ) ) ;
#62392=VECTOR ( 'NONE', #64314, 1000.000000000000000 ) ;
#62394=CARTESIAN_POINT ( 'NONE',  ( 7.725372132234999967, 1517.158319634930194, 211.9946825927569876 ) ) ;
#62411=CARTESIAN_POINT ( 'NONE',  ( 7.324914918154999732, 1516.685667699390024, 204.5043554653269950 ) ) ;
#62460=CARTESIAN_POINT ( 'NONE',  ( -2.485217232065000115, 1516.534320418310244, 201.4128137944169907 ) ) ;
#62464=CARTESIAN_POINT ( 'NONE',  ( 15.00522596483500060, 1511.839858410419993, 197.1933472413670074 ) ) ;
#62465=CARTESIAN_POINT ( 'NONE',  ( 7.594039249315000184, 1512.142919181319940, 206.8921143228970152 ) ) ;
#62477=CARTESIAN_POINT ( 'NONE',  ( -7.933914964464999109, 1511.279956263560052, 214.2433585108670115 ) ) ;
#62497=CARTESIAN_POINT ( 'NONE',  ( 1.131796810615000037, 1516.659138130710289, 214.8948242487770131 ) ) ;
#62498=CARTESIAN_POINT ( 'NONE',  ( 4.824494990945000339, 1511.382391139620040, 217.5855882746469945 ) ) ;
#62505=CARTESIAN_POINT ( 'NONE',  ( -6.559798094425000059, 1516.987478262539980, 204.5068286042669854 ) ) ;
#62508=CARTESIAN_POINT ( 'NONE',  ( 4.115882860026048640, 1509.032014410905504, 204.7576542507069064 ) ) ;
#62515=DIRECTION ( 'NONE',  ( 0.000000000000000000, -1.000000000000000000, 6.123233995736769734E-17 ) ) ;
#62518=CARTESIAN_POINT ( 'NONE',  ( 5.011367946795000528, 1516.974592746400049, 212.5716232859570027 ) ) ;
#62524=CARTESIAN_POINT ( 'NONE',  ( -2.480427292634999947, 1516.872851364150165, 209.8797317620669673 ) ) ;
#62541=CARTESIAN_POINT ( 'NONE',  ( -1.124289693584999972, 1517.184063036290127, 215.6857614941170027 ) ) ;
#62563=CARTESIAN_POINT ( 'NONE',  ( 7.012921468763117616, 1508.551704408389924, 215.5137847777533580 ) ) ;
#62570=EDGE_CURVE ( 'NONE', #42748, #21389, #20073, .T. ) ;
#62571=CARTESIAN_POINT ( 'NONE',  ( 12.10384758683500017, 1512.631076693560090, 200.5535322512070024 ) ) ;
#62631=CARTESIAN_POINT ( 'NONE',  ( -4.028611259245000298, 1516.744381837270112, 210.2562039408269925 ) ) ;
#62638=CARTESIAN_POINT ( 'NONE',  ( -6.554764199395000546, 1516.786099423779888, 201.4062207291269999 ) ) ;
#62643=CARTESIAN_POINT ( 'NONE',  ( 1.704170714124999986, 1516.927039499179955, 208.3639196453299860 ) ) ;
#62659=CARTESIAN_POINT ( 'NONE',  ( 3.445407533985000104, 1516.764084769670262, 206.8237970085970119 ) ) ;
#62677=CARTESIAN_POINT ( 'NONE',  ( -7.714371541114999786, 1516.738222552470233, 214.9014490703569891 ) ) ;
#62679=ORIENTED_EDGE ( 'NONE', *, *, #68157, .F. ) ;
#62690=EDGE_CURVE ( 'NONE', #29266, #71450, #78806, .T. ) ;
#62722=ORIENTED_EDGE ( 'NONE', *, *, #85806, .F. ) ;
#62740=ORIENTED_EDGE ( 'NONE', *, *, #109673, .T. ) ;
#62753=CARTESIAN_POINT ( 'NONE',  ( -7.338411997524999286, 1517.170512887980067, 206.6372682748769876 ) ) ;
#62793=CARTESIAN_POINT ( 'NONE',  ( -7.334328310795000583, 1517.005755693489846, 204.1179978101270081 ) ) ;
#62819=CARTESIAN_POINT ( 'NONE',  ( -6.911190420815000124, 1512.677556571440164, 201.0605893814370120 ) ) ;
#62824=CARTESIAN_POINT ( 'NONE',  ( -7.445038021963170216, 1508.731359867031642, 214.6352815288127545 ) ) ;
#62835=ADVANCED_FACE ( 'NONE', ( #27797 ), #109138, .F. ) ;
#62836=CARTESIAN_POINT ( 'NONE',  ( 14.49215842413499900, 1514.088841912139969, 225.6376920165670015 ) ) ;
#62844=CARTESIAN_POINT ( 'NONE',  ( 4.608021669135000664, 1516.660388280709867, 207.4085285224269910 ) ) ;
#62865=ORIENTED_EDGE ( 'NONE', *, *, #104723, .F. ) ;
#62866=CARTESIAN_POINT ( 'NONE',  ( -3.367054167445000079, 1511.558654537720031, 201.2679619493769962 ) ) ;
#62903=CARTESIAN_POINT ( 'NONE',  ( -1.713317447804999949, 1516.660388280709867, 204.5138242629670060 ) ) ;
#62923=CARTESIAN_POINT ( 'NONE',  ( 3.461047291624999911, 1516.858765657450249, 212.5691103191969944 ) ) ;
#62932=CARTESIAN_POINT ( 'NONE',  ( -8.526415774054999730, 1512.074228085009963, 215.5845765956869968 ) ) ;
#62943=CARTESIAN_POINT ( 'NONE',  ( 6.546039395294999785, 1516.565291103010168, 206.8289057630870218 ) ) ;
#62960=CARTESIAN_POINT ( 'NONE',  ( -2.290256301855000398, 1517.170721208160103, 216.0730210990169837 ) ) ;
#62962=CARTESIAN_POINT ( 'NONE',  ( 5.730039660753280195, 1510.523965798400013, 216.6735546448169885 ) ) ;
#62964=CARTESIAN_POINT ( 'NONE',  ( 5.786837678925000006, 1517.040132827679827, 212.3790665729270017 ) ) ;
#62967=CARTESIAN_POINT ( 'NONE',  ( 3.487586588140600075, 1508.731366866819826, 213.6768007754070027 ) ) ;
#62981=ORIENTED_EDGE ( 'NONE', *, *, #47307, .T. ) ;
#62982=CARTESIAN_POINT ( 'NONE',  ( -3.266349512195000138, 1516.797038924770050, 205.0935381919470046 ) ) ;
#63006=VECTOR ( 'NONE', #99383, 1000.000000000000000 ) ;
#63015=VERTEX_POINT ( 'NONE', #20310 ) ;
#63020=CARTESIAN_POINT ( 'NONE',  ( -12.53415180646500104, 1512.123798513659949, 192.8669541650669998 ) ) ;
#63024=CARTESIAN_POINT ( 'NONE',  ( -0.01010286742719850028, 1516.939452820819952, 201.4022050290969901 ) ) ;
#63031=CARTESIAN_POINT ( 'NONE',  ( -4.487249792034999629, 1509.038615934169911, 205.6342535031670025 ) ) ;
#63037=CARTESIAN_POINT ( 'NONE',  ( -7.557029945415000505, 1510.729589429620091, 214.2821637710270011 ) ) ;
#63055=CARTESIAN_POINT ( 'NONE',  ( -6.551643424905000401, 1516.807958722750072, 214.9033365145770063 ) ) ;
#63056=CARTESIAN_POINT ( 'NONE',  ( 2.234922648835000025, 1512.341036949130057, 216.7210731158769761 ) ) ;
#63057=VERTEX_POINT ( 'NONE', #1900 ) ;
#63064=CARTESIAN_POINT ( 'NONE',  ( 7.323974606304999746, 1516.647924054489977, 205.0857262875869935 ) ) ;
#63077=CARTESIAN_POINT ( 'NONE',  ( -4.997250192034999650, 1516.727068157269969, 212.3866247496169990 ) ) ;
#63083=CARTESIAN_POINT ( 'NONE',  ( -3.261652325025000021, 1516.939580991450157, 209.1351299096569960 ) ) ;
#63096=CARTESIAN_POINT ( 'NONE',  ( 3.487592428935230249, 1508.551704408389924, 214.1089243929580164 ) ) ;
#63098=CARTESIAN_POINT ( 'NONE',  ( 7.331183090945000203, 1516.882217593000178, 216.0635732225570109 ) ) ;
#63115=DIRECTION ( 'NONE',  ( -0.6742693640212139572, -4.521919481779819710E-17, -0.7384854939282339270 ) ) ;
#63119=EDGE_LOOP ( 'NONE', ( #37568, #69777, #14117, #37804 ) ) ;
#63128=CARTESIAN_POINT ( 'NONE',  ( -7.487063421429379417, 1517.051703294439903, 208.6815157772669806 ) ) ;
#63139=CARTESIAN_POINT ( 'NONE',  ( 13.34643004641739950, 1512.594488815719842, 224.4167555860190078 ) ) ;
#63177=CARTESIAN_POINT ( 'NONE',  ( 7.338753830235000386, 1517.184383877180153, 211.4127322367170052 ) ) ;
#63187=CARTESIAN_POINT ( 'NONE',  ( 1.125509850285000280, 1517.203017563489766, 201.7827387294869936 ) ) ;
#63207=DIRECTION ( 'NONE',  ( 0.000000000000000000, 6.123233995736769734E-17, 1.000000000000000000 ) ) ;
#63208=CARTESIAN_POINT ( 'NONE',  ( -5.787477032644999575, 1517.070197312179971, 206.2521524731670013 ) ) ;
#63222=EDGE_CURVE ( 'NONE', #98450, #2901, #15372, .T. ) ;
#63225=CARTESIAN_POINT ( 'NONE',  ( 5.007588646914999941, 1516.804776704140068, 214.8970827629769644 ) ) ;
#63239=CARTESIAN_POINT ( 'NONE',  ( 6.499999980935001531, 1515.051704408389924, 209.1218459511669892 ) ) ;
#63244=CARTESIAN_POINT ( 'NONE',  ( -1.906498070525230022E-08, 1509.051704408389924, 216.1347675157070114 ) ) ;
#63266=DIRECTION ( 'NONE',  ( -0.02616798426672899136, -0.9993150019883406676, 0.02616798426434139430 ) ) ;
#63280=CARTESIAN_POINT ( 'NONE',  ( -7.012524266536320106, 1508.551704613440052, 215.1061919086760099 ) ) ;
#63291=CARTESIAN_POINT ( 'NONE',  ( -1.718203501584999904, 1516.898441858519845, 207.4215862561470090 ) ) ;
#63311=CARTESIAN_POINT ( 'NONE',  ( 14.78591727178930171, 1514.559393050746394, 225.3792123963893630 ) ) ;
#63331=CARTESIAN_POINT ( 'NONE',  ( 5.000083827734999709, 1516.858456333729919, 204.1129977322069919 ) ) ;
#63354=CARTESIAN_POINT ( 'NONE',  ( -7.908505719245000343, 1514.005261957169978, 201.8728991555269943 ) ) ;
#63357=AXIS2_PLACEMENT_3D ( 'NONE', #65308, #39538, #73143 ) ;
#63372=CARTESIAN_POINT ( 'NONE',  ( 15.09659336983500033, 1514.030803186779849, 224.8374594117669858 ) ) ;
#63380=CARTESIAN_POINT ( 'NONE',  ( 0.7352271172030020452, 1516.963431999339946, 207.4067364850470199 ) ) ;
#63409=CARTESIAN_POINT ( 'NONE',  ( 7.703229013340137321, 1511.126521620285303, 203.6801736527461628 ) ) ;
#63419=CARTESIAN_POINT ( 'NONE',  ( 7.717505752974999744, 1516.857914730730045, 201.4043401791270185 ) ) ;
#63434=CARTESIAN_POINT ( 'NONE',  ( 7.711550677984999602, 1516.630499592039996, 205.0863552195469879 ) ) ;
#63454=EDGE_CURVE ( 'NONE', #94671, #42670, #81720, .T. ) ;
#63455=CARTESIAN_POINT ( 'NONE',  ( -5.771797464315000070, 1516.647618671360078, 211.9976960644470125 ) ) ;
#63464=CARTESIAN_POINT ( 'NONE',  ( -6.124171364995000033, 1514.216129015430170, 216.7908301805069868 ) ) ;
#63465=CARTESIAN_POINT ( 'NONE',  ( 16.52740840709205372, 1514.201209519783333, 194.8160859650000987 ) ) ;
#63479=CARTESIAN_POINT ( 'NONE',  ( -2.494758036134999912, 1516.937508036699910, 207.4208181092269854 ) ) ;
#63495=B_SPLINE_SURFACE_WITH_KNOTS ( 'NONE', 5, 5, ( 
 ( #84878, #24422, #84343, #7631, #101671, #24960 ),
 ( #42342, #58607, #76495, #72001, #70898, #97160 ),
 ( #62498, #36159, #106114, #70343, #3133, #87669 ),
 ( #9844, #19886, #44009, #96619, #52421, #61939 ),
 ( #103903, #2024, #61385, #11512, #35594, #95504 ),
 ( #27747, #96058, #46237, #78148, #104455, #20431 ),
 ( #80370, #12053, #1449, #69785, #19327, #27203 ),
 ( #3686, #78711, #18774, #52972, #105015, #105575 ),
 ( #37812, #79826, #87104, #37263, #18226, #79272 ),
 ( #28863, #54093, #28305, #54638, #53529, #88769 ),
 ( #2582, #10958, #29391, #10392, #88218, #44562 ),
 ( #45687, #94956, #36704, #86548, #71461, #63056 ) ),
 .UNSPECIFIED., .F., .F., .F.,
 ( 6, 3, 3, 6 ),
 ( 6, 6 ),
 ( 3.672001930560000016, 6.062162762929999893, 7.801458206499999548, 8.912489289840001661 ),
 ( 0.000000000000000000, 1.000000000000000000 ),
 .UNSPECIFIED. ) ;
#63497=CARTESIAN_POINT ( 'NONE',  ( -1.708747662384999977, 1517.213554313520035, 216.0740123525270064 ) ) ;
#63501=CARTESIAN_POINT ( 'NONE',  ( 7.724732408895000013, 1517.133889586189980, 212.3822030989969960 ) ) ;
#63521=CARTESIAN_POINT ( 'NONE',  ( 2.865911516645000212, 1516.906233342200039, 205.6598507734169914 ) ) ;
#63529=CARTESIAN_POINT ( 'NONE',  ( 4.811461131969293703, 1516.551188146008599, 199.9949300312234755 ) ) ;
#63540=CARTESIAN_POINT ( 'NONE',  ( -11.97304278378637576, 1513.029508366000300, 192.5452993188944504 ) ) ;
#63544=DIRECTION ( 'NONE',  ( -0.7071067811865492381, 0.000000000000000000, -0.7071067811865457964 ) ) ;
#63556=CARTESIAN_POINT ( 'NONE',  ( -12.80694037396500029, 1512.080583811389943, 193.5218228818669957 ) ) ;
#63559=CARTESIAN_POINT ( 'NONE',  ( -4.616861546545000472, 1516.666407245520077, 201.4093549791169835 ) ) ;
#63591=CARTESIAN_POINT ( 'NONE',  ( -0.7369042090349989804, 1517.080322339569875, 214.1333973382469935 ) ) ;
#63599=CARTESIAN_POINT ( 'NONE',  ( -4.040527342105000308, 1516.815231249920089, 204.5109077207270047 ) ) ;
#63611=B_SPLINE_CURVE_WITH_KNOTS ( 'NONE', 3,
 ( #449, #9376, #44092, #34570, #78230, #102859, #44651, #69864, #18855, #95586, #53051, #11040, #10481, #79348, #78792, #85507, #2662, #2108, #69306, #86080, #26156, #36234, #27836, #62016, #35124, #60342, #96136, #17737, #51938, #36787, #19415, #70980, #43539, #53616, #26718, #25601, #93913, #77684, #997, #103413, #81523, #11589, #3764, #89935, #20509, #97236, #88295, #12129, #38427, #5386, #46864, #80451, #22152, #80994, #30585, #79902, #4824, #4300, #12684, #82083, #88845, #29476, #46323, #21611 ),
 .UNSPECIFIED., .F., .F.,
 ( 4, 3, 3, 3, 3, 3, 3, 3, 3, 3, 3, 3, 3, 3, 3, 3, 3, 3, 3, 3, 3, 4 ),
 ( -14.97205155145559985, -14.82652002214629938, -14.54016898290000093, -14.44422383253650111, -14.18616176382849936, -13.96389086917469946, -13.75628494548289993, -13.55954878687630050, -13.48778832326109978, -13.41168605665509972, -13.29681976037920066, -13.03955770695989891, -12.77367886414240061, -12.48588961213089910, -12.17406815308810053, -11.81735425579999976, -11.73764647089110014, -11.37242228474149996, -11.02426971002140021, -10.95328097456370031, -10.66065571756510089, -10.38571964170729878 ),
 .UNSPECIFIED. ) ;
#63613=CARTESIAN_POINT ( 'NONE',  ( 4.623787969365000805, 1516.947419719950176, 212.5709951659769956 ) ) ;
#63619=CARTESIAN_POINT ( 'NONE',  ( -7.708918532268509871, 1516.529980546400111, 211.4477551148110024 ) ) ;
#63620=CARTESIAN_POINT ( 'NONE',  ( -7.332063977575000280, 1516.939491476980038, 209.1325772641960157 ) ) ;
#63634=CARTESIAN_POINT ( 'NONE',  ( 4.618119666265000589, 1516.706638732659940, 216.0591847158069925 ) ) ;
#63639=CARTESIAN_POINT ( 'NONE',  ( -3.454119954834999895, 1516.594591938570147, 201.4112355291069889 ) ) ;
#63640=CARTESIAN_POINT ( 'NONE',  ( -7.512750246095000861, 1509.038615934239942, 214.6352815282469919 ) ) ;
#63656=DIRECTION ( 'NONE',  ( 0.7071093782156816498, -3.166819169022306488E-06, 0.7071041841407837980 ) ) ;
#63676=CARTESIAN_POINT ( 'NONE',  ( 12.26154099264659969, 1512.129944624190102, 223.9167924943490107 ) ) ;
#63677=ORIENTED_EDGE ( 'NONE', *, *, #13848, .T. ) ;
#63696=EDGE_LOOP ( 'NONE', ( #64820, #18805, #26728, #33125 ) ) ;
#63712=EDGE_LOOP ( 'NONE', ( #38578, #3698, #22287, #69109 ) ) ;
#63714=ORIENTED_EDGE ( 'NONE', *, *, #86549, .F. ) ;
#63716=CARTESIAN_POINT ( 'NONE',  ( -6.548200625775000283, 1516.632821972880038, 210.2524534341069966 ) ) ;
#63722=CARTESIAN_POINT ( 'NONE',  ( -5.779603138255000161, 1516.738222552470233, 201.4074744291170020 ) ) ;
#63742=CARTESIAN_POINT ( 'NONE',  ( -3.268859434184999913, 1516.922519270759949, 206.6438591998669949 ) ) ;
#63758=CARTESIAN_POINT ( 'NONE',  ( -4.613762395014999740, 1516.939574742129935, 214.9064842900469898 ) ) ;
#63760=CARTESIAN_POINT ( 'NONE',  ( 7.709189683329709553, 1516.540336843770092, 207.3380993366749863 ) ) ;
#63778=CARTESIAN_POINT ( 'NONE',  ( -7.260306344532728495, 1509.032998971549432, 202.6015535907291110 ) ) ;
#63803=CARTESIAN_POINT ( 'NONE',  ( 4.329791490734999471, 1515.051704408389924, 209.1218459511669892 ) ) ;
#63833=CARTESIAN_POINT ( 'NONE',  ( 4.997718238375000510, 1516.693851263360102, 207.9888968556769839 ) ) ;
#63840=EDGE_CURVE ( 'NONE', #94274, #12190, #39344, .T. ) ;
#63849=PLANE ( 'NONE',  #73165 ) ;
#63853=CARTESIAN_POINT ( 'NONE',  ( 11.11245944731352964, 1512.836811624652455, 225.1840528857647996 ) ) ;
#63854=ORIENTED_EDGE ( 'NONE', *, *, #40285, .T. ) ;
#63870=CARTESIAN_POINT ( 'NONE',  ( -4.620008245204999753, 1516.777260590120022, 203.3472363101570011 ) ) ;
#63892=CARTESIAN_POINT ( 'NONE',  ( -6.580362948704999937, 1511.382498894319951, 201.8051239266270045 ) ) ;
#63907=CARTESIAN_POINT ( 'NONE',  ( 12.93225138353500192, 1513.362623229679912, 226.0086287796669922 ) ) ;
#63915=CARTESIAN_POINT ( 'NONE',  ( 1.700259675955000160, 1516.898441858519845, 207.4036424686470070 ) ) ;
#63943=AXIS2_PLACEMENT_3D ( 'NONE', #64200, #82067, #71526 ) ;
#63975=CARTESIAN_POINT ( 'NONE',  ( -1.715361130375000043, 1516.743010792419909, 205.6766444437269854 ) ) ;
#63978=EDGE_CURVE ( 'NONE', #44160, #78578, #99993, .T. ) ;
#63991=CARTESIAN_POINT ( 'NONE',  ( 2.494757998004999866, 1516.937508036699910, 210.8228737931069929 ) ) ;
#64005=CARTESIAN_POINT ( 'NONE',  ( -6.382129857305000264, 1514.500328598809801, 216.9911249345570070 ) ) ;
#64006=CARTESIAN_POINT ( 'NONE',  ( 16.38124166206986132, 1514.407859675132613, 194.5303642102901165 ) ) ;
#64017=CARTESIAN_POINT ( 'NONE',  ( -6.950833568235000648, 1517.156142772249950, 206.6378959915070084 ) ) ;
#64027=CARTESIAN_POINT ( 'NONE',  ( -5.784678387216369622, 1511.501844456730169, 200.3524772839079731 ) ) ;
#64034=CARTESIAN_POINT ( 'NONE',  ( -1.124289693584999972, 1517.184063036290127, 215.6857614941170027 ) ) ;
#64038=CARTESIAN_POINT ( 'NONE',  ( 2.492130623175000448, 1516.778761582560037, 212.5675310476169955 ) ) ;
#64055=CARTESIAN_POINT ( 'NONE',  ( -0.01306004006829850073, 1516.939762005280045, 204.5032625402269844 ) ) ;
#64080=CARTESIAN_POINT ( 'NONE',  ( -4.486733153042460565, 1517.051705360449887, 216.7144192674729766 ) ) ;
#64093=CARTESIAN_POINT ( 'NONE',  ( -11.87063488596499816, 1512.258183966700017, 192.7384874028670083 ) ) ;
#64097=CARTESIAN_POINT ( 'NONE',  ( -0.01073133209419849937, 1516.939491476980038, 201.7897819926569980 ) ) ;
#64113=CARTESIAN_POINT ( 'NONE',  ( -7.572192888655000509, 1511.308638870219966, 211.6864797536570109 ) ) ;
#64124=CYLINDRICAL_SURFACE ( 'NONE', #59047, 0.9999999999999522604 ) ;
#64135=CARTESIAN_POINT ( 'NONE',  ( 4.037378256055000669, 1516.688761843659904, 215.6706679112870120 ) ) ;
#64145=CARTESIAN_POINT ( 'NONE',  ( 6.937338745574999521, 1516.706638732659940, 204.5037262658370025 ) ) ;
#64156=VECTOR ( 'NONE', #83504, 1000.000000000000114 ) ;
#64158=CARTESIAN_POINT ( 'NONE',  ( -5.772727946874999461, 1516.691414181030041, 212.5791125756269935 ) ) ;
#64163=CARTESIAN_POINT ( 'NONE',  ( -7.717618918966349995, 1516.862251239950183, 209.3707541584199987 ) ) ;
#64164=CARTESIAN_POINT ( 'NONE',  ( 2.486220101774999858, 1516.939658295650133, 209.1086089184300079 ) ) ;
#64173=DIRECTION ( 'NONE',  ( -4.336808689942001466E-16, -0.02617694830786544691, -0.9996573249755575929 ) ) ;
#64175=CARTESIAN_POINT ( 'NONE',  ( -1.906499846882070084E-08, 1517.051704408389924, 209.1218459511669892 ) ) ;
#64176=CARTESIAN_POINT ( 'NONE',  ( 6.942973629204999497, 1516.833844030519913, 216.4505221401170161 ) ) ;
#64181=CARTESIAN_POINT ( 'NONE',  ( 2.483949940595000516, 1517.156142772249950, 202.1710124019969896 ) ) ;
#64182=CARTESIAN_POINT ( 'NONE',  ( -15.87603345926499898, 1512.359593911809952, 220.1461273412669755 ) ) ;
#64183=EDGE_LOOP ( 'NONE', ( #40392, #77225, #101031, #5525 ) ) ;
#64198=DIRECTION ( 'NONE',  ( 0.000000000000000000, 0.06174578541841399537, -0.9980919085851078787 ) ) ;
#64200=CARTESIAN_POINT ( 'NONE',  ( 4.487249753905000027, 1509.038615934239942, 209.1218459511669892 ) ) ;
#64218=CARTESIAN_POINT ( 'NONE',  ( 14.02477538797010048, 1513.114148093580070, 224.3898003711330205 ) ) ;
#64259=CARTESIAN_POINT ( 'NONE',  ( 3.269184908365000197, 1516.940296199220029, 211.4060453336370244 ) ) ;
#64261=CARTESIAN_POINT ( 'NONE',  ( -4.996642198295000448, 1516.697242742309982, 211.9989590406970024 ) ) ;
#64269=B_SPLINE_CURVE_WITH_KNOTS ( 'NONE', 3,
 ( #32959, #67148, #65493, #24545, #40816, #15041, #99603, #58733, #22886, #57096, #74995, #91221, #107464, #32426, #66605, #58186, #15585, #83921, #92870, #99054, #7764, #30759, #73329, #14502, #68266, #17237, #85016, #16687, #50884, #34073, #102373, #60965, #86135, #18357, #69361, #101809, #8310, #33499, #94519, #110782, #25101, #60400, #103471, #77199, #59306, #95640, #104035, #25656, #26778, #502, #8859, #43042, #52551, #9978, #51432 ),
 .UNSPECIFIED., .F., .F.,
 ( 4, 3, 3, 3, 3, 3, 3, 3, 3, 3, 3, 3, 3, 3, 3, 3, 3, 3, 4 ),
 ( 9.902195898180000455, 10.17210527305439882, 10.45530577770670000, 10.70141353110000004, 11.00396970307760114, 11.32322756684139975, 11.52456852350000105, 11.84989040644859948, 12.16242387756629917, 12.38020728900000123, 12.74551463659910056, 13.12275145100690033, 13.53252099859349933, 13.95359103984709925, 14.40783883437189949, 14.91487510439959863, 15.44821056985129992, 15.94145638718300084, 16.40090783169999966 ),
 .UNSPECIFIED. ) ;
#64270=CARTESIAN_POINT ( 'NONE',  ( -6.942973667334999988, 1516.833844030519913, 201.7931697622170191 ) ) ;
#64272=CYLINDRICAL_SURFACE ( 'NONE', #58857, 4.999999999999991118 ) ;
#64286=CARTESIAN_POINT ( 'NONE',  ( 5.789394662204999875, 1517.164987839469859, 210.8286437561770299 ) ) ;
#64288=CARTESIAN_POINT ( 'NONE',  ( -7.722580350941189664, 1517.051704403100075, 204.5317855550379988 ) ) ;
#64292=CARTESIAN_POINT ( 'NONE',  ( 7.784559201385000016, 1511.207707629420156, 205.1306841488269868 ) ) ;
#64294=CARTESIAN_POINT ( 'NONE',  ( 2.477373605864999995, 1516.891731298979948, 206.2406231745169976 ) ) ;
#64311=CARTESIAN_POINT ( 'NONE',  ( -4.032397940005000514, 1516.981965530290154, 214.9074288837770155 ) ) ;
#64313=CARTESIAN_POINT ( 'NONE',  ( 7.708916871849369024, 1516.529918593650109, 207.1343159654149986 ) ) ;
#64314=DIRECTION ( 'NONE',  ( 0.000000000000000000, -6.123233995736769734E-17, -1.000000000000000000 ) ) ;
#64338=CARTESIAN_POINT ( 'NONE',  ( -6.009430644317174774, 1511.590044791479613, 200.3317612525653146 ) ) ;
#64340=CARTESIAN_POINT ( 'NONE',  ( -4.987078460856490203, 1508.551704408389924, 212.6094383991630252 ) ) ;
#64354=VECTOR ( 'NONE', #47318, 1000.000000000000114 ) ;
#64379=CARTESIAN_POINT ( 'NONE',  ( 6.546001350565000543, 1516.557392317769882, 207.4118413833070065 ) ) ;
#64401=CARTESIAN_POINT ( 'NONE',  ( 14.32486855194574105, 1514.214507861885295, 225.6406290981485370 ) ) ;
#64408=CARTESIAN_POINT ( 'NONE',  ( 4.491288147733260239, 1508.884219112060009, 205.6342589211700158 ) ) ;
#64418=CARTESIAN_POINT ( 'NONE',  ( 6.550389432124999800, 1516.755758396839838, 204.1155163507169732 ) ) ;
#64419=VERTEX_POINT ( 'NONE', #3852 ) ;
#64425=ORIENTED_EDGE ( 'NONE', *, *, #47515, .T. ) ;
#64450=( BOUNDED_CURVE ( )  B_SPLINE_CURVE ( 3, ( #43703, #10658, #9535, #37936 ),
 .UNSPECIFIED., .F., .F. ) 
 B_SPLINE_CURVE_WITH_KNOTS ( ( 4, 4 ),
 ( 5.447131716497383813, 6.315249268839017383 ),
 .UNSPECIFIED. ) 
 CURVE ( )  GEOMETRIC_REPRESENTATION_ITEM ( )  RATIONAL_B_SPLINE_CURVE ( ( 1.000000000000000000, 0.9381775213688714476, 0.9381775213688714476, 1.000000000000000000 ) ) 
 REPRESENTATION_ITEM ( '' )  );
#64459=CARTESIAN_POINT ( 'NONE',  ( 12.85600963073500047, 1512.300546902530186, 224.3151201823670249 ) ) ;
#64468=CARTESIAN_POINT ( 'NONE',  ( 2.864043418315000089, 1516.811292230880099, 206.8228319013669818 ) ) ;
#64503=VERTEX_POINT ( 'NONE', #33238 ) ;
#64515=CARTESIAN_POINT ( 'NONE',  ( -2.941312998452541905, 1512.218159651617725, 201.2357107834446026 ) ) ;
#64523=CARTESIAN_POINT ( 'NONE',  ( 3.253462060665000433, 1516.874084700499907, 205.6604858388269861 ) ) ;
#64538=CARTESIAN_POINT ( 'NONE',  ( 4.044319887224999910, 1517.073005577650065, 210.2423896678870108 ) ) ;
#64552=CARTESIAN_POINT ( 'NONE',  ( -6.490306558154999905, 1514.605246816799763, 217.1492952416969899 ) ) ;
#64558=CARTESIAN_POINT ( 'NONE',  ( -3.487585887316744238, 1508.611350403811230, 204.4436907818935367 ) ) ;
#64567=CARTESIAN_POINT ( 'NONE',  ( -1.133653179125000188, 1516.978425811520083, 208.3843950493249793 ) ) ;
#64579=CARTESIAN_POINT ( 'NONE',  ( -5.424122872404329776, 1511.219705715099963, 201.2551218106839883 ) ) ;
#64586=CARTESIAN_POINT ( 'NONE',  ( -6.553524415734999664, 1516.882690742909972, 216.0660777183969969 ) ) ;
#64591=CARTESIAN_POINT ( 'NONE',  ( -4.028630622785000170, 1516.812923327049930, 212.5819478221170016 ) ) ;
#64608=CARTESIAN_POINT ( 'NONE',  ( 6.935457925184999262, 1516.627618683580067, 205.6664679548470076 ) ) ;
#64610=ADVANCED_FACE ( 'NONE', ( #97028 ), #28712, .F. ) ;
#64616=CARTESIAN_POINT ( 'NONE',  ( 5.371346801041280372, 1516.551188146539971, 199.4837300725229738 ) ) ;
#64635=CARTESIAN_POINT ( 'NONE',  ( 7.953529549975883128, 1511.798530722474197, 205.9061371885316021 ) ) ;
#64646=CARTESIAN_POINT ( 'NONE',  ( -13.06501233546500096, 1513.192861445620110, 192.2233964041670049 ) ) ;
#64651=CARTESIAN_POINT ( 'NONE',  ( -3.455378015385000001, 1516.627618683580067, 202.1863880069169852 ) ) ;
#64671=ADVANCED_FACE ( 'NONE', ( #31126 ), #22698, .T. ) ;
#64679=CARTESIAN_POINT ( 'NONE',  ( 7.597790773094999395, 1511.735270473989885, 202.7837360344269939 ) ) ;
#64689=CARTESIAN_POINT ( 'NONE',  ( -7.328049318385000177, 1516.809497469189864, 215.6772390872569929 ) ) ;
#64697=CARTESIAN_POINT ( 'NONE',  ( 1.120543697654999837, 1517.073005577650065, 205.0775260448770041 ) ) ;
#64699=CARTESIAN_POINT ( 'NONE',  ( -2.873919040654999701, 1516.940252185109784, 209.1351185066319829 ) ) ;
#64703=CARTESIAN_POINT ( 'NONE',  ( 6.098897513495000311, 1511.444830760690138, 216.7818499078069863 ) ) ;
#64711=EDGE_CURVE ( 'NONE', #88321, #65245, #85320, .T. ) ;
#64714=CARTESIAN_POINT ( 'NONE',  ( 3.266349474065000091, 1516.797038924770050, 213.1501537103870021 ) ) ;
#64719=DIRECTION ( 'NONE',  ( -1.000000000000000000, 0.000000000000000000, 0.000000000000000000 ) ) ;
#64720=CARTESIAN_POINT ( 'NONE',  ( -7.709692149626850011, 1516.559523801380010, 210.7009757622840027 ) ) ;
#64721=CARTESIAN_POINT ( 'NONE',  ( -5.770820179264999794, 1516.591755933730155, 210.8331571987770019 ) ) ;
#64735=CARTESIAN_POINT ( 'NONE',  ( 1.708720984574999768, 1516.531533746980131, 216.4430152012269843 ) ) ;
#64740=CARTESIAN_POINT ( 'NONE',  ( -2.485846037024999955, 1516.545806094630279, 201.8003900583769905 ) ) ;
#64772=DIRECTION ( 'NONE',  ( 0.000000000000000000, 0.02617694830742899742, -0.9996573249755689172 ) ) ;
#64774=DIRECTION ( 'NONE',  ( 0.000000000000000000, -1.000000000000000000, 6.123233995736769734E-17 ) ) ;
#64820=ORIENTED_EDGE ( 'NONE', *, *, #46780, .T. ) ;
#64821=CARTESIAN_POINT ( 'NONE',  ( 6.563595869685000750, 1517.154223579619838, 211.4114704024570131 ) ) ;
#64823=CARTESIAN_POINT ( 'NONE',  ( 4.624736859184999993, 1516.994127245590107, 211.9896495963369887 ) ) ;
#64829=CARTESIAN_POINT ( 'NONE',  ( -3.454119954834999895, 1516.594591938570147, 201.4112355291069889 ) ) ;
#64842=CARTESIAN_POINT ( 'NONE',  ( -6.935801299664999142, 1516.621991115350056, 210.2518484644969874 ) ) ;
#64845=EDGE_CURVE ( 'NONE', #68294, #30006, #42290, .T. ) ;
#64848=CARTESIAN_POINT ( 'NONE',  ( 7.853883982725000656, 1511.558654537720031, 205.7547918027769924 ) ) ;
#64849=CARTESIAN_POINT ( 'NONE',  ( 7.323390407215000231, 1516.613712827999962, 207.9924597298270044 ) ) ;
#64866=CARTESIAN_POINT ( 'NONE',  ( 6.556651371285000529, 1516.858146885269889, 215.6747433371770057 ) ) ;
#64870=DIRECTION ( 'NONE',  ( -0.7071067811865474617, -6.092092863024105611E-16, -0.7071067811865474617 ) ) ;
#64892=CARTESIAN_POINT ( 'NONE',  ( -5.381312013895000135, 1511.468585915670019, 200.7968825106569852 ) ) ;
#64913=DIRECTION ( 'NONE',  ( 0.7384854939282345931, 0.000000000000000000, -0.6742693640212131800 ) ) ;
#64920=DIRECTION ( 'NONE',  ( -0.01802056537744943510, 0.000000000000000000, 0.9998376164275263323 ) ) ;
#64923=CARTESIAN_POINT ( 'NONE',  ( 13.62888593203049936, 1517.051704413129983, 191.9442378289920157 ) ) ;
#64925=CARTESIAN_POINT ( 'NONE',  ( -7.679314503873669651, 1511.182265711489890, 215.0124326349510113 ) ) ;
#64929=CARTESIAN_POINT ( 'NONE',  ( 1.701850457105000158, 1516.908147884120126, 207.9845492812970065 ) ) ;
#64944=CARTESIAN_POINT ( 'NONE',  ( 7.683535900364350191, 1517.051704408389924, 209.5573457314510222 ) ) ;
#64965=CARTESIAN_POINT ( 'NONE',  ( -0.7560907659159991079, 1516.770163853809890, 204.1215159365669933 ) ) ;
#64970=ORIENTED_EDGE ( 'NONE', *, *, #78200, .F. ) ;
#64972=CARTESIAN_POINT ( 'NONE',  ( 13.78858221403500117, 1513.492015765619954, 196.0403704991670111 ) ) ;
#64973=CARTESIAN_POINT ( 'NONE',  ( -12.49443853494850032, 1512.179780174510142, 194.1456554007820330 ) ) ;
#65025=CARTESIAN_POINT ( 'NONE',  ( 5.371346801041280372, 1516.551188146539971, 199.4837300725229738 ) ) ;
#65043=EDGE_CURVE ( 'NONE', #33692, #51877, #87676, .T. ) ;
#65054=CARTESIAN_POINT ( 'NONE',  ( -4.822683201000122821, 1511.395345385124756, 200.6579470351961447 ) ) ;
#65061=CARTESIAN_POINT ( 'NONE',  ( 7.710285837685000310, 1516.582197289609894, 205.8614676770269796 ) ) ;
#65075=CARTESIAN_POINT ( 'NONE',  ( -2.284053509485000077, 1516.854133554269993, 210.2586600040969813 ) ) ;
#65076=EDGE_CURVE ( 'NONE', #63057, #1893, #94643, .T. ) ;
#65088=ORIENTED_EDGE ( 'NONE', *, *, #93993, .F. ) ;
#65105=CARTESIAN_POINT ( 'NONE',  ( 4.035536225084999984, 1517.086065052259983, 201.3983658527070020 ) ) ;
#65106=CARTESIAN_POINT ( 'NONE',  ( 2.480427254505000345, 1516.872851364150165, 208.3639601402670110 ) ) ;
#65117=CARTESIAN_POINT ( 'NONE',  ( -5.718152507175660482, 1511.533951550999973, 200.6987238893559891 ) ) ;
#65125=CARTESIAN_POINT ( 'NONE',  ( -1.710012758625000018, 1517.232977404109988, 216.8491730849570160 ) ) ;
#65129=CARTESIAN_POINT ( 'NONE',  ( 4.622842844184999578, 1516.901952101700090, 213.1523604828169880 ) ) ;
#65132=FACE_OUTER_BOUND ( 'NONE', #109991, .T. ) ;
#65147=CARTESIAN_POINT ( 'NONE',  ( 6.936398355645000180, 1516.667393516340098, 205.0850970932970085 ) ) ;
#65184=B_SPLINE_SURFACE_WITH_KNOTS ( 'NONE', 5, 5, ( 
 ( #41690, #268, #60163, #79728, #20887, #69690, #61294, #71357, #87001 ),
 ( #104357, #3585, #54544, #3037, #45587, #87575, #10289, #88129, #1927 ),
 ( #89212, #18676, #97073, #10862, #44467, #88677, #11955, #45035, #96515 ),
 ( #46141, #36065, #71910, #105471, #52872, #78611, #95412, #11418, #106026 ),
 ( #70250, #37709, #103810, #79180, #95960, #19794, #27109, #70804, #62962 ),
 ( #80270, #12507, #62391, #28758, #27654, #28203, #61840, #53996, #29301 ) ),
 .UNSPECIFIED., .F., .F., .F.,
 ( 6, 6 ),
 ( 6, 3, 6 ),
 ( 4.238752792101460720, 5.659133035218539831 ),
 ( 0.000000000000000000, 0.5000000000000000000, 1.002061266618540003 ),
 .UNSPECIFIED. ) ;
#65186=CARTESIAN_POINT ( 'NONE',  ( -7.544470660387704974, 1510.539524133948362, 214.8487628643081848 ) ) ;
#65189=CARTESIAN_POINT ( 'NONE',  ( -11.65415826906500030, 1512.679339245399888, 192.6383097548670094 ) ) ;
#65193=CARTESIAN_POINT ( 'NONE',  ( 5.778372563615000068, 1516.932669162149978, 202.1763558832970205 ) ) ;
#65196=CARTESIAN_POINT ( 'NONE',  ( 16.30040990573499826, 1513.841826332629807, 194.4616504171669931 ) ) ;
#65208=CARTESIAN_POINT ( 'NONE',  ( 15.93623140273500027, 1515.958428328729951, 224.2983129015669874 ) ) ;
#65209=CARTESIAN_POINT ( 'NONE',  ( -7.599227183775000505, 1512.341036949130057, 211.3567686190669974 ) ) ;
#65220=CARTESIAN_POINT ( 'NONE',  ( 8.502796018205000195, 1512.371933174390051, 202.2779677156470086 ) ) ;
#65230=CARTESIAN_POINT ( 'NONE',  ( 1.130002494264999990, 1516.621991115350056, 216.0576472317669925 ) ) ;
#65238=CARTESIAN_POINT ( 'NONE',  ( -0.7574260232259989456, 1516.837969789639828, 205.8660360680970030 ) ) ;
#65240=CARTESIAN_POINT ( 'NONE',  ( -2.286472924554999953, 1516.883361325900069, 209.8798303522490016 ) ) ;
#65245=VERTEX_POINT ( 'NONE', #88981 ) ;
#65253=CARTESIAN_POINT ( 'NONE',  ( -6.936398393775000670, 1516.667393516340098, 213.1585948090369698 ) ) ;
#65260=CARTESIAN_POINT ( 'NONE',  ( -7.709227547919620172, 1516.541781377989992, 210.8861241254419951 ) ) ;
#65261=CARTESIAN_POINT ( 'NONE',  ( 7.727327114725000001, 1517.232977404109988, 210.8318586907270173 ) ) ;
#65270=LINE ( 'NONE', #15919, #98570 ) ;
#65275=CARTESIAN_POINT ( 'NONE',  ( -7.716878941104999612, 1516.833976295079992, 216.4517711926369827 ) ) ;
#65279=ORIENTED_EDGE ( 'NONE', *, *, #68769, .T. ) ;
#65280=CARTESIAN_POINT ( 'NONE',  ( 5.003220727074999985, 1516.983995446890049, 202.1750974131470286 ) ) ;
#65286=CARTESIAN_POINT ( 'NONE',  ( 8.159522702327139498, 1511.384172056590160, 203.7268068870999969 ) ) ;
#65295=CARTESIAN_POINT ( 'NONE',  ( -7.512750246095000861, 1509.038615934239942, 209.1218459511669892 ) ) ;
#65308=CARTESIAN_POINT ( 'NONE',  ( 7.499999980934999755, 1508.551704408389924, 209.1218459511669892 ) ) ;
#65316=B_SPLINE_CURVE_WITH_KNOTS ( 'NONE', 5,
 ( #48604, #58104, #62824, #83835, #97476, #14959 ),
 .UNSPECIFIED., .F., .F.,
 ( 6, 6 ),
 ( 0.000000000000000000, 1.000000000000000000 ),
 .UNSPECIFIED. ) ;
#65319=CARTESIAN_POINT ( 'NONE',  ( 15.01814799273499901, 1514.214451716350140, 223.8476172842669882 ) ) ;
#65321=ORIENTED_EDGE ( 'NONE', *, *, #103887, .F. ) ;
#65330=EDGE_CURVE ( 'NONE', #42405, #39998, #88863, .T. ) ;
#65334=DIRECTION ( 'NONE',  ( 0.7071067811865474617, 5.170588477393925004E-17, 0.7071067811865474617 ) ) ;
#65357=ORIENTED_EDGE ( 'NONE', *, *, #85080, .T. ) ;
#65362=CARTESIAN_POINT ( 'NONE',  ( 2.882325979385000014, 1516.969638403840008, 210.8235757905769674 ) ) ;
#65366=CARTESIAN_POINT ( 'NONE',  ( -2.284526496774999860, 1516.956048353049937, 212.5847947667770086 ) ) ;
#65373=CARTESIAN_POINT ( 'NONE',  ( 2.483949940595000516, 1517.156142772249950, 202.1710124019969896 ) ) ;
#65388=CARTESIAN_POINT ( 'NONE',  ( 4.045182479925000685, 1517.057265928030120, 210.8256255754569963 ) ) ;
#65393=CARTESIAN_POINT ( 'NONE',  ( 8.072094028204999105, 1511.572472350439739, 205.5103833285670021 ) ) ;
#65394=CARTESIAN_POINT ( 'NONE',  ( -7.726331963605000297, 1517.194972660189933, 206.8303316343270239 ) ) ;
#65411=CARTESIAN_POINT ( 'NONE',  ( -5.777745433405000242, 1516.908489800550115, 215.6797558528670038 ) ) ;
#65412=VERTEX_POINT ( 'NONE', #66850 ) ;
#65441=CARTESIAN_POINT ( 'NONE',  ( -5.385523199825000162, 1511.435001052829875, 200.4690698299770020 ) ) ;
#65451=EDGE_CURVE ( 'NONE', #29671, #19743, #54418, .T. ) ;
#65466=CYLINDRICAL_SURFACE ( 'NONE', #83954, 4.999999999999997335 ) ;
#65484=CARTESIAN_POINT ( 'NONE',  ( 2.284053471355000031, 1516.854133554269993, 207.9850318982369970 ) ) ;
#65493=CARTESIAN_POINT ( 'NONE',  ( -14.79494656225329940, 1512.129944624190102, 221.3833869628849698 ) ) ;
#65516=VECTOR ( 'NONE', #73290, 1000.000000000000000 ) ;
#65520=CARTESIAN_POINT ( 'NONE',  ( 7.323974606304999746, 1516.647924054489977, 205.0857262875869935 ) ) ;
#65526=ORIENTED_EDGE ( 'NONE', *, *, #47307, .F. ) ;
#65529=CARTESIAN_POINT ( 'NONE',  ( -12.67335160806310057, 1512.240709848920005, 194.0399737768200055 ) ) ;
#65541=CARTESIAN_POINT ( 'NONE',  ( -8.041028958794997905, 1514.881364185380107, 203.0257501012370369 ) ) ;
#65542=VERTEX_POINT ( 'NONE', #42734 ) ;
#65558=CARTESIAN_POINT ( 'NONE',  ( 11.40944910055886119, 1511.843510977572350, 224.6458867293904405 ) ) ;
#65597=ORIENTED_EDGE ( 'NONE', *, *, #6913, .T. ) ;
#65616=CARTESIAN_POINT ( 'NONE',  ( 6.547881374914999775, 1516.647534046129977, 205.6658385469270058 ) ) ;
#65619=CARTESIAN_POINT ( 'NONE',  ( -17.05226164202473882, 1516.729020965289237, 195.6302442682282390 ) ) ;
#65624=ORIENTED_EDGE ( 'NONE', *, *, #33357, .F. ) ;
#65626=ORIENTED_EDGE ( 'NONE', *, *, #106248, .T. ) ;
#65631=CARTESIAN_POINT ( 'NONE',  ( -5.772978316675000166, 1516.659138130710289, 210.2536427808470023 ) ) ;
#65639=CARTESIAN_POINT ( 'NONE',  ( 7.891777514710270225, 1512.314860025949883, 206.1798159824890035 ) ) ;
#65655=CARTESIAN_POINT ( 'NONE',  ( -2.873329398885000163, 1516.572193931679976, 201.7997408644770019 ) ) ;
#65656=CARTESIAN_POINT ( 'NONE',  ( 5.772978278544999675, 1516.659138130710289, 207.9900491214870044 ) ) ;
#65666=CARTESIAN_POINT ( 'NONE',  ( -5.890586702848469969, 1511.182265711499895, 201.4425314663570248 ) ) ;
#65674=CARTESIAN_POINT ( 'NONE',  ( -6.554778571775000451, 1516.929962200689943, 216.8412383526069789 ) ) ;
#65679=CARTESIAN_POINT ( 'NONE',  ( 6.948321705865000197, 1517.049325831759916, 213.1561268858870051 ) ) ;
#65691=PLANE ( 'NONE',  #143 ) ;
#65698=CARTESIAN_POINT ( 'NONE',  ( 4.027697225915000345, 1516.766397346390022, 206.2431526829570032 ) ) ;
#65718=CARTESIAN_POINT ( 'NONE',  ( -11.56086350461344203, 1512.916370508231921, 192.7448627781640766 ) ) ;
#65726=CARTESIAN_POINT ( 'NONE',  ( 7.892106848066304359, 1512.076549611834707, 206.1384687351585967 ) ) ;
#65736=CARTESIAN_POINT ( 'NONE',  ( -15.27973131726499822, 1514.812393650459853, 193.2888744509670005 ) ) ;
#65741=CARTESIAN_POINT ( 'NONE',  ( 6.552897366944999469, 1516.858146885269889, 202.5651945608169910 ) ) ;
#65745=CARTESIAN_POINT ( 'NONE',  ( 15.07517727483500103, 1511.972232048389969, 196.8177839844669847 ) ) ;
#65757=CARTESIAN_POINT ( 'NONE',  ( -7.772759728185000938, 1512.089957059379913, 211.9637779886270152 ) ) ;
#65778=CARTESIAN_POINT ( 'NONE',  ( 6.555393117025000826, 1516.809497469189864, 216.4498952504870033 ) ) ;
#65785=CARTESIAN_POINT ( 'NONE',  ( -2.879956963085000154, 1516.827328999679821, 205.8693153165069702 ) ) ;
#65787=CARTESIAN_POINT ( 'NONE',  ( -7.724874651314999952, 1517.139320148880188, 208.3815253650730028 ) ) ;
#65790=CARTESIAN_POINT ( 'NONE',  ( 6.372167600554999645, 1511.069621805459974, 216.5183910133669940 ) ) ;
#65799=CARTESIAN_POINT ( 'NONE',  ( -7.324914956285000223, 1516.685667699390024, 213.7393364370070117 ) ) ;
#65805=CARTESIAN_POINT ( 'NONE',  ( -7.709335680692180226, 1516.545910801970194, 210.8355061257960017 ) ) ;
#65807=CARTESIAN_POINT ( 'NONE',  ( 4.044319887224999910, 1517.073005577650065, 210.2423896678870108 ) ) ;
#65824=CARTESIAN_POINT ( 'NONE',  ( -4.034280953785000179, 1517.049325831759916, 216.0701676760970145 ) ) ;
#65830=CARTESIAN_POINT ( 'NONE',  ( 3.259101798884999734, 1517.102359858469754, 202.1722709844570147 ) ) ;
#65831=CARTESIAN_POINT ( 'NONE',  ( -14.72576942166499947, 1512.123542805230272, 221.3115653187670091 ) ) ;
#65909=CARTESIAN_POINT ( 'NONE',  ( 6.950833530105000158, 1517.156142772249950, 211.6057959108269984 ) ) ;
#65914=CARTESIAN_POINT ( 'NONE',  ( -5.772403812434999892, 1516.676340709600026, 212.3853678745870184 ) ) ;
#65920=CARTESIAN_POINT ( 'NONE',  ( 2.289624432225000117, 1517.154223579619838, 202.5582500624169882 ) ) ;
#65921=B_SPLINE_CURVE_WITH_KNOTS ( 'NONE', 3,
 ( #17448, #68461, #33718, #43790, #76847, #18015 ),
 .UNSPECIFIED., .F., .F.,
 ( 4, 2, 4 ),
 ( 0.000000000000000000, 0.5000000000000000000, 1.000000000000000000 ),
 .UNSPECIFIED. ) ;
#65937=CARTESIAN_POINT ( 'NONE',  ( -5.770820179264999794, 1516.591755933730155, 210.8331571987770019 ) ) ;
#65944=CARTESIAN_POINT ( 'NONE',  ( 4.995623452895000760, 1516.636036526019780, 207.4092012159470073 ) ) ;
#65965=CARTESIAN_POINT ( 'NONE',  ( 1.130002494264999990, 1516.621991115350056, 216.0576472317669925 ) ) ;
#65967=CARTESIAN_POINT ( 'NONE',  ( 7.714047019527109583, 1516.725831029360052, 208.3892583435649897 ) ) ;
#65992=FACE_OUTER_BOUND ( 'NONE', #54343, .T. ) ;
#66000=FACE_OUTER_BOUND ( 'NONE', #41676, .T. ) ;
#66005=ORIENTED_EDGE ( 'NONE', *, *, #34619, .T. ) ;
#66010=VERTEX_POINT ( 'NONE', #15865 ) ;
#66034=CARTESIAN_POINT ( 'NONE',  ( -8.795269478359751147, 1511.561753607920082, 215.0949048348660142 ) ) ;
#66040=CARTESIAN_POINT ( 'NONE',  ( -4.623892098755000291, 1517.066898074209803, 208.3852847535989952 ) ) ;
#66057=DIRECTION ( 'NONE',  ( -1.000000000000000000, 0.000000000000000000, 0.000000000000000000 ) ) ;
#66067=ORIENTED_EDGE ( 'NONE', *, *, #68632, .T. ) ;
#66074=CARTESIAN_POINT ( 'NONE',  ( -4.678149174004739841, 1508.611352721110052, 205.6342598901590009 ) ) ;
#66076=CARTESIAN_POINT ( 'NONE',  ( 0.7360974386200019870, 1517.045004075700035, 205.0794574309270217 ) ) ;
#66079=CARTESIAN_POINT ( 'NONE',  ( 15.10840964654390106, 1512.260118274579781, 196.3980101966029963 ) ) ;
#66173=CARTESIAN_POINT ( 'NONE',  ( -3.965320971343086143, 1511.478961035300472, 200.9376376759473146 ) ) ;
#66179=CARTESIAN_POINT ( 'NONE',  ( -3.267291643295000103, 1516.842852731759876, 205.6749038603869906 ) ) ;
#66192=CARTESIAN_POINT ( 'NONE',  ( 2.882325979385000014, 1516.969638403840008, 210.8235757905769674 ) ) ;
#66214=CARTESIAN_POINT ( 'NONE',  ( -3.487585001760570069, 1508.551704408610021, 204.2892291422272422 ) ) ;
#66221=CARTESIAN_POINT ( 'NONE',  ( 1.124894050234999998, 1517.194816588360027, 202.1703287997270309 ) ) ;
#66222=CARTESIAN_POINT ( 'NONE',  ( 2.477975315464999717, 1516.839862955080207, 207.9852983471170091 ) ) ;
#66229=DIRECTION ( 'NONE',  ( 0.7071067811865492381, 0.000000000000000000, 0.7071067811865457964 ) ) ;
#66235=CARTESIAN_POINT ( 'NONE',  ( -5.593955164791184487, 1510.491946807396744, 201.5711409828585943 ) ) ;
#66241=CARTESIAN_POINT ( 'NONE',  ( 4.035490712554999249, 1516.630499592039996, 216.8333966482170183 ) ) ;
#66244=DIRECTION ( 'NONE',  ( 0.4770263929453174567, 0.7067418228236591604, 0.5224574779878943254 ) ) ;
#66245=EDGE_CURVE ( 'NONE', #27633, #46347, #59749, .T. ) ;
#66246=CARTESIAN_POINT ( 'NONE',  ( 0.4409583776298362512, 1516.806451497312082, 216.8380041110111733 ) ) ;
#66247=CARTESIAN_POINT ( 'NONE',  ( -2.866857931135000204, 1516.951766529250108, 213.1652121904069759 ) ) ;
#66250=CARTESIAN_POINT ( 'NONE',  ( 4.364191146503010543, 1509.032029208890208, 213.2377284900549910 ) ) ;
#66253=AXIS2_PLACEMENT_3D ( 'NONE', #68512, #16397, #42189 ) ;
#66267=CARTESIAN_POINT ( 'NONE',  ( -0.7572979743539989261, 1516.829948096479939, 205.6721984920870057 ) ) ;
#66287=CARTESIAN_POINT ( 'NONE',  ( -14.47444372044108540, 1514.320539547600902, 192.6747587196877021 ) ) ;
#66295=CARTESIAN_POINT ( 'NONE',  ( 8.003677881822152784, 1511.683950138178034, 205.7359720134772090 ) ) ;
#66305=CARTESIAN_POINT ( 'NONE',  ( -14.92730992206499785, 1514.452905717119847, 192.9094359382670234 ) ) ;
#66310=CARTESIAN_POINT ( 'NONE',  ( 6.553524377605000062, 1516.882690742909972, 202.1776141839370098 ) ) ;
#66313=CARTESIAN_POINT ( 'NONE',  ( 16.25489176703500149, 1512.123798513659949, 196.5876941637669688 ) ) ;
#66332=DIRECTION ( 'NONE',  ( 0.000000000000000000, -6.123233995736769734E-17, -1.000000000000000000 ) ) ;
#66345=CARTESIAN_POINT ( 'NONE',  ( -5.777745433405000242, 1516.908489800550115, 215.6797558528670038 ) ) ;
#66346=CARTESIAN_POINT ( 'NONE',  ( -8.374266313531483874, 1511.401872466645500, 213.6732156279371679 ) ) ;
#66352=CARTESIAN_POINT ( 'NONE',  ( -3.461047329755000401, 1516.858765657450249, 205.6745815831370123 ) ) ;
#66354=CARTESIAN_POINT ( 'NONE',  ( -3.261652325025000021, 1516.939580991450157, 209.1351299096569960 ) ) ;
#66357=CARTESIAN_POINT ( 'NONE',  ( 6.998420849865000015, 1512.696049264760177, 217.3137064069569817 ) ) ;
#66366=CARTESIAN_POINT ( 'NONE',  ( 0.7568986996720019622, 1516.805675336850072, 213.1530147380969993 ) ) ;
#66370=CARTESIAN_POINT ( 'NONE',  ( 7.203708765649230017, 1508.728101229370168, 215.8474698634739752 ) ) ;
#66371=CARTESIAN_POINT ( 'NONE',  ( 3.462835627365000057, 1517.038650117239968, 210.2415636864969883 ) ) ;
#66386=CARTESIAN_POINT ( 'NONE',  ( 5.779603100124999671, 1516.738222552470233, 216.8362174732170047 ) ) ;
#66391=CARTESIAN_POINT ( 'NONE',  ( -7.718763544034999313, 1516.905946377369901, 202.1794916586869988 ) ) ;
#66392=CARTESIAN_POINT ( 'NONE',  ( -16.74824993986500132, 1512.868709057589967, 222.4423585103670007 ) ) ;
#66412=CARTESIAN_POINT ( 'NONE',  ( -4.534010781284650626, 1508.610336716400070, 213.3588268743650076 ) ) ;
#66419=CARTESIAN_POINT ( 'NONE',  ( -1.906531099660209973E-08, 1509.038615934239942, 204.6345961781970004 ) ) ;
#66431=CARTESIAN_POINT ( 'NONE',  ( 6.218727018272192986, 1516.719877041854261, 204.9285666176960206 ) ) ;
#66441=LINE ( 'NONE', #24929, #57322 ) ;
#66445=CARTESIAN_POINT ( 'NONE',  ( -4.858360422201509543, 1508.551704408389469, 205.6342535009236485 ) ) ;
#66470=CARTESIAN_POINT ( 'NONE',  ( 1.136547584984999970, 1516.839862955080207, 211.5998212856970042 ) ) ;
#66474=CARTESIAN_POINT ( 'NONE',  ( -6.547881413045000265, 1516.647534046129977, 212.5778533554070293 ) ) ;
#66478=ORIENTED_EDGE ( 'NONE', *, *, #98695, .F. ) ;
#66481=CARTESIAN_POINT ( 'NONE',  ( -5.006329619514999330, 1516.755758396839838, 202.5714564999769891 ) ) ;
#66498=CARTESIAN_POINT ( 'NONE',  ( 2.493699768634999536, 1516.858326417339867, 211.5985794462469869 ) ) ;
#66504=CARTESIAN_POINT ( 'NONE',  ( -6.952166420425000659, 1517.213554313520035, 207.4130983078469797 ) ) ;
#66522=CARTESIAN_POINT ( 'NONE',  ( 5.780861236055000241, 1516.783701990830195, 216.0610654530370027 ) ) ;
#66541=ADVANCED_FACE ( 'NONE', ( #65992 ), #73266, .F. ) ;
#66545=DIRECTION ( 'NONE',  ( -0.9996573249755574819, 0.02617694830786558916, 0.000000000000000000 ) ) ;
#66548=DIRECTION ( 'NONE',  ( 0.000000000000000000, -1.000000000000000000, 6.123233995736769734E-17 ) ) ;
#66574=DIRECTION ( 'NONE',  ( -1.000000000000000000, 0.000000000000000000, 0.000000000000000000 ) ) ;
#66576=CARTESIAN_POINT ( 'NONE',  ( -13.33054336736499934, 1520.551704408390151, 207.1218459511669892 ) ) ;
#66586=DIRECTION ( 'NONE',  ( 0.8236474686107847498, 0.5669078173018529121, 0.01484500364079605582 ) ) ;
#66597=CARTESIAN_POINT ( 'NONE',  ( 1.122033391945000069, 1516.972341476009888, 208.3659064338399673 ) ) ;
#66605=CARTESIAN_POINT ( 'NONE',  ( -15.13257544217990080, 1512.281672892730057, 221.8969035856549965 ) ) ;
#66616=EDGE_LOOP ( 'NONE', ( #65624, #63677, #107058, #2847, #46095, #20833, #70570, #110142, #14609, #95631 ) ) ;
#66631=CARTESIAN_POINT ( 'NONE',  ( 2.285487581364999965, 1517.001127920769704, 205.0775242521070254 ) ) ;
#66634=CARTESIAN_POINT ( 'NONE',  ( 14.72577158086200022, 1514.214451999800076, 194.1036973123569851 ) ) ;
#66639=CARTESIAN_POINT ( 'NONE',  ( -12.22498602940789958, 1512.125809830880144, 194.3608099058220091 ) ) ;
#66649=CARTESIAN_POINT ( 'NONE',  ( -7.962346614255001676, 1514.830240247470101, 203.0623562961069979 ) ) ;
#66658=FACE_OUTER_BOUND ( 'NONE', #15150, .T. ) ;
#66692=EDGE_CURVE ( 'NONE', #65245, #46100, #72070, .T. ) ;
#66714=CARTESIAN_POINT ( 'NONE',  ( 14.84895960065126275, 1511.957228877181251, 197.0446257365507563 ) ) ;
#66724=CARTESIAN_POINT ( 'NONE',  ( -1.135460355084999762, 1516.790374942449944, 205.8685445508469911 ) ) ;
#66734=CARTESIAN_POINT ( 'NONE',  ( -15.90990515426090113, 1514.921193439799936, 224.3246443988719818 ) ) ;
#66738=CARTESIAN_POINT ( 'NONE',  ( -3.251611363945000388, 1516.779243033999819, 211.4202154400570066 ) ) ;
#66752=EDGE_LOOP ( 'NONE', ( #236, #82196, #100471, #80676 ) ) ;
#66769=CARTESIAN_POINT ( 'NONE',  ( 2.290886266485000267, 1517.184383877180153, 201.7830921018669983 ) ) ;
#66770=CARTESIAN_POINT ( 'NONE',  ( -5.014195139944999546, 1517.120861839400050, 207.4163795216369977 ) ) ;
#66778=CARTESIAN_POINT ( 'NONE',  ( 9.638115859575000499, 1520.551704408390151, 214.4931927712770232 ) ) ;
#66787=CARTESIAN_POINT ( 'NONE',  ( 3.454748808194999743, 1516.609912606490070, 216.4448802441970088 ) ) ;
#66792=CARTESIAN_POINT ( 'NONE',  ( 0.01306000193830150063, 1516.939762005280045, 213.7404293621069939 ) ) ;
#66809=CARTESIAN_POINT ( 'NONE',  ( -4.623788007495000407, 1516.947419719950176, 205.6726967363569827 ) ) ;
#66824=FACE_OUTER_BOUND ( 'NONE', #91934, .T. ) ;
#66845=CARTESIAN_POINT ( 'NONE',  ( -7.465999380592456269, 1510.821818217233613, 215.2858853877662284 ) ) ;
#66850=CARTESIAN_POINT ( 'NONE',  ( -7.722579826676089887, 1517.051704428850144, 208.6871515679729896 ) ) ;
#66854=CARTESIAN_POINT ( 'NONE',  ( -0.7543882209519990889, 1516.727502608469877, 202.5709757879969857 ) ) ;
#66857=CARTESIAN_POINT ( 'NONE',  ( 15.26322408243500028, 1511.857118786289902, 196.9337341496670035 ) ) ;
#66868=ORIENTED_EDGE ( 'NONE', *, *, #805, .F. ) ;
#66870=LINE ( 'NONE', #65208, #99347 ) ;
#66877=B_SPLINE_SURFACE_WITH_KNOTS ( 'NONE', 5, 5, ( 
 ( #86686, #9980, #44150, #78285, #79403, #85563, #8860, #20563, #54764, #72660, #28442, #81041, #4354, #90538, #105151, #55315, #55871, #97833, #30642, #73203, #96757, #20029, #39598, #106250, #64829, #79950, #47456, #39024, #63722, #62638, #54223, #80507, #88896 ),
 ( #13817, #29535, #21111, #72131, #3266, #45817, #28999, #88349, #11639, #3823, #37395, #71596, #98937, #105716, #63187, #81580, #21662, #12739, #97293, #12181, #107347, #46372, #89447, #4883, #37952, #82139, #106787, #46922, #38483, #30078, #64270, #98392, #89992 ),
 ( #22212, #56408, #13267, #48002, #5440, #67024, #14373, #49116, #40141, #84885, #92199, #65373, #7094, #100042, #23871, #31736, #101131, #41251, #8179, #50749, #74325, #33377, #93294, #92745, #109562, #91647, #49667, #99477, #48565, #6545, #40695, #24426, #82702 ),
 ( #59175, #23331, #58612, #5991, #83248, #108454, #73770, #15471, #22758, #75424, #57522, #58066, #65920, #16020, #32831, #107893, #31186, #14922, #67573, #16556, #50221, #84347, #74867, #83799, #56964, #109013, #32298, #66481, #7638, #100589, #41793, #91093, #75952 ),
 ( #110103, #101677, #24966, #27753, #70348, #35046, #110650, #69226, #42911, #43466, #34500, #33937, #1461, #35598, #68677, #103337, #93832, #10399, #9848, #18780, #60836, #61390, #95509, #78715, #78152, #86553, #19335, #77612, #102781, #96063, #42346, #9301, #52978 ),
 ( #61946, #76501, #26640, #103909, #94963, #2031, #44569, #68135, #102246, #87679, #923, #36163, #17105, #87110, #104460, #18231, #25526, #59715, #17665, #26075, #27207, #53535, #85433, #378, #51296, #52426, #69789, #8731, #77068, #60267, #94386, #51866, #44017 ),
 ( #86004, #19895, #64145, #38352, #29397, #105021, #56273, #89866, #54098, #12058, #98263, #79278, #98815, #89317, #45136, #80376, #88226, #12613, #46794, #4221, #72007, #37821, #105583, #13135, #47319, #63599, #107219, #37272, #72531, #62505, #97166, #11518, #22077 ),
 ( #29951, #63064, #96624, #45693, #106661, #2587, #10964, #70904, #81446, #30507, #46246, #28314, #21532, #79832, #64697, #4754, #3138, #71466, #28870, #38897, #36711, #20437, #3691, #54645, #73080, #88776, #106123, #20988, #55747, #97717, #55193, #80923, #47869 ),
 ( #5871, #67450, #101549, #41675, #82006, #5311, #57400, #6421, #99349, #15890, #66899, #58485, #48991, #56828, #82580, #23200, #91527, #108324, #39469, #49540, #40013, #74193, #57940, #13682, #66352, #100470, #75834, #90403, #40566, #41115, #83123, #50089, #92613 ),
 ( #73641, #74737, #90963, #31057, #23753, #92072, #15345, #24842, #101006, #84217, #14805, #7515, #107771, #109984, #108875, #32166, #83665, #65238, #22624, #14250, #48440, #31607, #65785, #99905, #6962, #33261, #75294, #109439, #32718, #24305, #77492, #42230, #104339 ),
 ( #60145, #17542, #43886, #84762, #1908, #27092, #51744, #36046, #792, #25395, #52854, #85878, #69670, #18656, #50630, #59044, #94265, #93166, #86982, #16436, #8059, #69108, #9720, #44448, #10271, #9181, #76378, #43344, #59587, #34921, #51180, #110527, #18110 ),
 ( #103209, #68005, #95392, #35477, #61276, #26515, #93703, #85310, #102650, #25950, #76939, #33811, #52306, #8605, #42780, #60713, #102116, #94834, #86430, #78592, #16981, #78030, #1338, #103792, #70233, #250, #34377, #68550, #72952, #28738, #64017, #2467, #80798 ),
 ( #4637, #4104, #106542, #62943, #29831, #19201, #47197, #97054, #20318, #105449, #36584, #79159, #62369, #53403, #87554, #3014, #45014, #70781, #21404, #61818, #104894, #38228, #55063, #46115, #10842, #27632, #98129, #28183, #54524, #72412, #95941, #38776, #106007 ),
 ( #96495, #80246, #19774, #55614, #88658, #89738, #13011, #81323, #3564, #53976, #88109, #20868, #11398, #37138, #45567, #79708, #37686, #71335, #71891, #11935, #29283, #63479, #89190, #97597, #12483, #46665, #107645, #66770, #15745, #15210, #32033, #14116, #82990 ),
 ( #73509, #39336, #83527, #75160, #65656, #30928, #99218, #39888, #74055, #48307, #21947, #66222, #22496, #56697, #74607, #30377, #6282, #40430, #92475, #107088, #57272, #57812, #99773, #32593, #109307, #98687, #56140, #41547, #108184, #100869, #81878, #49401, #40980 ),
 ( #6821, #24160, #31475, #58350, #90276, #49946, #23062, #91399, #14677, #5180, #47743, #65106, #13557, #90833, #82448, #5745, #48864, #84084, #64567, #108742, #7382, #23630, #100341, #91936, #10137, #43748, #7926, #76795, #52159, #33127, #52709, #43204, #109850 ),
 ( #17404, #42096, #69528, #68420, #86292, #77899, #1206, #94133, #61135, #101974, #68974, #16303, #51051, #76244, #86844, #51600, #67314, #9032, #25260, #25814, #33671, #103075, #77354, #75703, #101411, #110391, #35340, #95249, #94691, #656, #93573, #85733, #24703 ),
 ( #67863, #103648, #58900, #93032, #112, #50507, #26946, #84629, #59463, #34787, #26376, #18512, #16848, #102522, #85183, #60012, #8469, #34234, #42642, #60571, #17964, #9576, #36435, #106802, #95796, #13832, #62227, #70086, #4898, #70632, #104750, #13281, #78452 ),
 ( #31204, #44308, #30092, #107362, #38499, #82156, #48018, #35903, #104199, #91112, #46937, #5455, #19063, #98952, #90554, #4370, #1765, #27484, #19631, #28037, #30657, #56980, #87407, #2325, #39614, #72676, #39038, #53268, #73784, #107909, #64842, #61673, #81056 ),
 ( #10700, #44872, #22225, #73218, #64286, #79023, #96353, #65388, #53832, #98407, #56424, #87971, #22775, #47472, #12756, #21678, #55885, #81594, #99492, #90005, #75439, #41266, #109033, #84364, #93309, #91662, #109576, #76514, #65937, #6560, #58080, #84901, #8193 ),
 ( #40711, #32846, #83264, #41810, #92759, #59730, #102260, #14937, #42359, #33957, #33391, #50237, #32315, #101146, #6006, #100061, #92213, #15485, #7654, #23348, #7112, #82716, #16570, #74883, #67038, #110663, #74341, #49132, #24986, #68152, #75967, #16037, #49683 ),
 ( #25540, #14388, #40158, #108468, #83812, #24439, #57538, #50766, #101693, #48581, #58628, #66498, #100604, #110119, #67587, #23886, #59190, #31752, #69806, #103924, #79291, #93850, #44030, #44585, #86569, #19350, #61961, #85447, #8744, #28327, #94978, #53549, #68690 ),
 ( #61403, #70921, #70362, #96075, #18245, #87697, #42928, #2601, #52441, #9862, #60853, #102795, #34512, #17679, #77085, #393, #69243, #26092, #60281, #10977, #17121, #94401, #36178, #10416, #1479, #51883, #51310, #45150, #86019, #78166, #104475, #9318, #105037 ),
 ( #35610, #43483, #27222, #77626, #36726, #95525, #27769, #938, #35061, #18797, #103352, #26653, #87126, #52993, #78731, #2046, #73656, #80936, #54110, #106675, #88788, #12629, #20450, #89878, #29965, #107787, #39485, #63077, #22090, #82021, #81461, #98276, #80389 ),
 ( #54659, #28882, #105599, #56289, #88239, #62518, #63613, #96641, #90417, #19910, #11531, #72544, #13148, #47883, #13697, #55204, #45706, #89332, #97177, #97729, #12069, #79844, #21550, #55762, #46261, #46806, #3153, #30523, #64158, #38910, #4234, #4767, #73093 ),
 ( #47333, #37286, #21000, #3704, #5325, #107232, #37834, #71477, #72019, #64714, #106136, #29413, #38368, #98831, #50646, #66366, #14265, #50105, #82594, #84776, #109997, #99921, #108339, #74211, #101567, #22639, #76391, #32182, #31072, #24857, #65253, #90977, #41129 ),
 ( #41688, #93182, #92630, #109453, #100485, #57415, #8073, #42243, #16449, #56844, #99365, #108889, #57953, #40029, #67464, #7531, #33273, #23766, #31623, #23215, #74752, #92086, #49005, #48456, #101021, #91541, #14818, #32732, #5884, #6978, #75310, #65799, #83140 ),
 ( #15361, #6435, #66912, #84230, #15904, #40580, #49554, #83679, #24318, #58501, #75847, #59058, #87573, #86998, #78609, #809, #1925, #102129, #19219, #34935, #69121, #77506, #85325, #51194, #34391, #25409, #59601, #85894, #16994, #8620, #104355, #33830, #42796 ),
 ( #266, #103808, #52324, #35493, #69688, #103225, #26534, #95409, #93718, #53422, #36062, #60731, #10860, #86448, #76956, #27651, #94852, #10287, #70248, #61837, #18127, #95957, #25964, #27107, #68567, #9199, #102665, #45033, #9738, #43904, #44464, #78045, #110542 ),
 ( #1354, #61292, #18674, #68021, #60160, #94281, #17558, #51760, #52870, #43361, #53994, #21423, #13027, #37707, #36602, #104912, #54542, #105469, #64034, #90294, #11416, #37160, #47214, #71908, #38246, #19792, #81341, #38794, #98148, #2485, #3583, #88127, #80815 ),
 ( #55633, #106561, #97615, #62388, #13574, #4654, #45585, #80266, #89756, #70800, #56158, #46683, #28201, #106024, #79726, #4121, #72429, #29848, #29299, #63497, #62960, #72969, #107106, #3033, #20885, #30396, #71354, #28756, #11953, #64586, #98705, #21964, #20337 ),
 ( #79178, #96513, #97071, #88675, #46137, #55083, #89208, #12504, #66787, #99238, #67335, #15765, #5764, #14137, #90850, #7402, #39355, #93052, #48883, #47760, #41567, #81895, #107663, #57829, #109327, #33147, #75723, #40448, #5200, #74625, #48327, #83010, #39906 ),
 ( #40998, #74076, #108760, #22513, #49965, #15230, #24182, #66241, #100887, #58370, #84103, #83546, #91955, #24723, #6302, #108205, #101433, #73529, #30949, #65125, #32051, #109868, #56716, #92496, #58920, #100360, #82466, #31493, #23083, #65674, #32611, #99792, #57292 ) ),
 .UNSPECIFIED., .F., .F., .F.,
 ( 6, 3, 3, 3, 3, 3, 3, 3, 3, 3, 6 ),
 ( 6, 3, 3, 3, 3, 3, 3, 3, 3, 3, 6 ),
 ( 0.000000000000000000, 1.936717162300000128, 3.873434324599999812, 4.841792905749999321, 5.810151486899999718, 7.746868649199999624, 9.683585811500000418, 10.65194439270000082, 11.62030297379999944, 13.55702013610000023, 15.49373729840000102 ),
 ( 0.000000000000000000, 1.936717162300000128, 3.873434324599999812, 4.841792905749999321, 5.810151486899999718, 7.746868649199999624, 9.683585811500000418, 10.65194439270000082, 11.62030297379999944, 13.55702013610000023, 15.49373729840000102 ),
 .UNSPECIFIED. ) ;
#66882=ORIENTED_EDGE ( 'NONE', *, *, #83756, .T. ) ;
#66885=VERTEX_POINT ( 'NONE', #84818 ) ;
#66890=CARTESIAN_POINT ( 'NONE',  ( -1.708747662384999977, 1517.213554313520035, 216.0740123525270064 ) ) ;
#66899=CARTESIAN_POINT ( 'NONE',  ( 2.865911516645000212, 1516.906233342200039, 205.6598507734169914 ) ) ;
#66901=CARTESIAN_POINT ( 'NONE',  ( -3.455495871984999745, 1516.939877939420057, 209.1351200182310208 ) ) ;
#66912=CARTESIAN_POINT ( 'NONE',  ( 6.946748518954999341, 1516.983995446890049, 214.1250666973070054 ) ) ;
#66916=CARTESIAN_POINT ( 'NONE',  ( 6.551871745751780551, 1508.551566289579796, 216.0836877189279903 ) ) ;
#66917=CARTESIAN_POINT ( 'NONE',  ( -3.447128498755000159, 1516.778853242349896, 210.2570310142770040 ) ) ;
#66937=CARTESIAN_POINT ( 'NONE',  ( -7.331183129075000693, 1516.882217593000178, 202.1801186797769674 ) ) ;
#66963=CARTESIAN_POINT ( 'NONE',  ( 5.303300839834999891, 1513.301704408390151, 219.3748942783669804 ) ) ;
#66980=CARTESIAN_POINT ( 'NONE',  ( 13.92686551478569967, 1517.051704405520013, 192.0624604828410043 ) ) ;
#67016=CARTESIAN_POINT ( 'NONE',  ( -4.028307778284999863, 1516.797038924770050, 212.3881954442970255 ) ) ;
#67024=CARTESIAN_POINT ( 'NONE',  ( 5.003220727074999985, 1516.983995446890049, 202.1750974131470286 ) ) ;
#67035=DIRECTION ( 'NONE',  ( -0.7071067811865474617, -5.176495448588656087E-16, 0.7071067811865474617 ) ) ;
#67038=CARTESIAN_POINT ( 'NONE',  ( -3.445407572115000150, 1516.764084769670262, 211.4198948937369948 ) ) ;
#67044=CARTESIAN_POINT ( 'NONE',  ( -1.137296688934999800, 1516.908147884120126, 207.4199954749970232 ) ) ;
#67059=CARTESIAN_POINT ( 'NONE',  ( -2.867803664234999772, 1516.994127245590107, 213.7465828294170080 ) ) ;
#67062=CARTESIAN_POINT ( 'NONE',  ( 7.331183090945000203, 1516.882217593000178, 216.0635732225570109 ) ) ;
#67101=DIRECTION ( 'NONE',  ( -1.000000000000000000, 0.000000000000000000, 0.000000000000000000 ) ) ;
#67109=CARTESIAN_POINT ( 'NONE',  ( 3.330134165755000097, 1515.051704408389924, 213.4516374609670208 ) ) ;
#67121=DIRECTION ( 'NONE',  ( -0.7384854939282339270, -4.299149317525499380E-13, 0.6742693640212139572 ) ) ;
#67134=CARTESIAN_POINT ( 'NONE',  ( -8.654780631634018562, 1511.434547101049930, 214.5059332195740183 ) ) ;
#67139=CARTESIAN_POINT ( 'NONE',  ( 4.618583391875000110, 1516.939762005280045, 209.1087859301640322 ) ) ;
#67148=CARTESIAN_POINT ( 'NONE',  ( -14.76103606440959837, 1512.125809830880144, 221.3468319615099915 ) ) ;
#67150=CARTESIAN_POINT ( 'NONE',  ( -8.652776130911478347, 1511.435001053830092, 214.5073691320910143 ) ) ;
#67172=CARTESIAN_POINT ( 'NONE',  ( 3.448206878685000198, 1516.904492006980036, 205.0794281543969646 ) ) ;
#67175=CARTESIAN_POINT ( 'NONE',  ( 14.90569722004390130, 1513.941944658620059, 194.3080451509249826 ) ) ;
#67230=ORIENTED_EDGE ( 'NONE', *, *, #49168, .T. ) ;
#67245=CARTESIAN_POINT ( 'NONE',  ( 15.90990255763500016, 1516.551704408390151, 198.1616908427670296 ) ) ;
#67257=ORIENTED_EDGE ( 'NONE', *, *, #35093, .F. ) ;
#67264=DIRECTION ( 'NONE',  ( 0.02616798426500960631, -0.9993150019883682011, -0.02616798426500960631 ) ) ;
#67265=CARTESIAN_POINT ( 'NONE',  ( 15.78436436265907794, 1512.151624459632103, 197.9925267198427150 ) ) ;
#67272=CARTESIAN_POINT ( 'NONE',  ( 3.446942071715000111, 1516.842852731759876, 205.8545543269370057 ) ) ;
#67283=CYLINDRICAL_SURFACE ( 'NONE', #77827, 0.4999999999999909517 ) ;
#67287=CARTESIAN_POINT ( 'NONE',  ( -7.321169269124999879, 1516.531533746980131, 210.8305669548069829 ) ) ;
#67308=CARTESIAN_POINT ( 'NONE',  ( 4.752602785698186949, 1516.784510156639953, 214.9408003802788301 ) ) ;
#67312=ORIENTED_EDGE ( 'NONE', *, *, #90442, .F. ) ;
#67313=CARTESIAN_POINT ( 'NONE',  ( -6.942973667334999988, 1516.833844030519913, 201.7931697622170191 ) ) ;
#67314=CARTESIAN_POINT ( 'NONE',  ( -1.906501101195560124E-08, 1517.020990152690047, 209.1218459511669892 ) ) ;
#67318=CARTESIAN_POINT ( 'NONE',  ( 4.963882991561403557, 1511.398734635483606, 217.6327391777064122 ) ) ;
#67328=CARTESIAN_POINT ( 'NONE',  ( -16.82650407848411334, 1517.015068014068447, 194.8356516383118731 ) ) ;
#67335=CARTESIAN_POINT ( 'NONE',  ( 2.873329360754999673, 1516.572193931679976, 216.4439510378570048 ) ) ;
#67338=CARTESIAN_POINT ( 'NONE',  ( 0.8595391288403605445, 1516.693423516305984, 216.8350443691653879 ) ) ;
#67339=CARTESIAN_POINT ( 'NONE',  ( -2.286446363765000100, 1517.042661899400173, 213.7475398352470108 ) ) ;
#67359=CARTESIAN_POINT ( 'NONE',  ( -7.724423432224999608, 1517.122088787240045, 205.6676733166769964 ) ) ;
#67407=CARTESIAN_POINT ( 'NONE',  ( -7.333070173014999860, 1516.955859323880077, 203.3428461583270064 ) ) ;
#67410=CARTESIAN_POINT ( 'NONE',  ( 16.76527320893499962, 1513.875858217490077, 195.2591379279669752 ) ) ;
#67435=CARTESIAN_POINT ( 'NONE',  ( 6.059489635994999013, 1514.830240247470101, 201.1594993559769762 ) ) ;
#67436=ORIENTED_EDGE ( 'NONE', *, *, #43456, .T. ) ;
#67444=CARTESIAN_POINT ( 'NONE',  ( 1.128757561074999805, 1516.608208975040043, 216.8328129478670121 ) ) ;
#67445=CARTESIAN_POINT ( 'NONE',  ( -8.652776130911478347, 1511.435001053830092, 214.5073691320910143 ) ) ;
#67450=CARTESIAN_POINT ( 'NONE',  ( 7.323034273964999841, 1516.609912606490070, 205.6670971239069843 ) ) ;
#67455=CARTESIAN_POINT ( 'NONE',  ( 7.587489894784999578, 1513.914017980350081, 215.5240844366570059 ) ) ;
#67464=CARTESIAN_POINT ( 'NONE',  ( 1.133516965105000107, 1516.713079096360161, 213.7319258036569920 ) ) ;
#67467=CARTESIAN_POINT ( 'NONE',  ( 7.443079126130860423, 1508.729257035799947, 215.2419638459840030 ) ) ;
#67468=CARTESIAN_POINT ( 'NONE',  ( 5.012938863775000087, 1517.051603658920158, 211.6026598552170128 ) ) ;
#67480=B_SPLINE_CURVE_WITH_KNOTS ( 'NONE', 5,
 ( #4188, #53086, #103450, #94499, #27869, #81411 ),
 .UNSPECIFIED., .F., .F.,
 ( 6, 6 ),
 ( 0.000000000000000000, 1.000000000000000000 ),
 .UNSPECIFIED. ) ;
#67482=CARTESIAN_POINT ( 'NONE',  ( 11.02428137103500028, 1512.359593911809952, 224.9978793913670074 ) ) ;
#67484=CARTESIAN_POINT ( 'NONE',  ( -4.616899872884999922, 1517.050041317280147, 216.8443827349270236 ) ) ;
#67489=CARTESIAN_POINT ( 'NONE',  ( -1.709358701255000001, 1516.542957540330008, 202.1882582765869927 ) ) ;
#67547=CARTESIAN_POINT ( 'NONE',  ( 7.509820308583667448, 1510.675349056233244, 203.1409315813798173 ) ) ;
#67559=ORIENTED_EDGE ( 'NONE', *, *, #103432, .T. ) ;
#67565=CARTESIAN_POINT ( 'NONE',  ( -5.551188713984379852, 1510.480349263560129, 201.5713426139130320 ) ) ;
#67566=CARTESIAN_POINT ( 'NONE',  ( 3.460101851884999746, 1516.812923327049930, 213.1504765548870068 ) ) ;
#67573=CARTESIAN_POINT ( 'NONE',  ( -1.130607502004999931, 1516.632821972880038, 202.5736453444569918 ) ) ;
#67587=CARTESIAN_POINT ( 'NONE',  ( 1.136547584984999970, 1516.839862955080207, 211.5998212856970042 ) ) ;
#67592=CARTESIAN_POINT ( 'NONE',  ( -4.625790014595000166, 1517.104192383289956, 208.0004623403669939 ) ) ;
#67607=CARTESIAN_POINT ( 'NONE',  ( -7.324914956285000223, 1516.685667699390024, 213.7393364370070117 ) ) ;
#67610=CARTESIAN_POINT ( 'NONE',  ( -4.033653302454999867, 1517.028034847769959, 215.6825881955670070 ) ) ;
#67630=ORIENTED_EDGE ( 'NONE', *, *, #49168, .F. ) ;
#67687=CARTESIAN_POINT ( 'NONE',  ( -8.490445737682099647, 1511.451733153379791, 214.5038762997880042 ) ) ;
#67692=CARTESIAN_POINT ( 'NONE',  ( 5.006259848694999626, 1516.939723362869927, 209.1089481433290018 ) ) ;
#67697=ORIENTED_EDGE ( 'NONE', *, *, #11192, .F. ) ;
#67725=CARTESIAN_POINT ( 'NONE',  ( -5.009478105444999940, 1516.886345593249871, 204.5093386581970094 ) ) ;
#67728=CARTESIAN_POINT ( 'NONE',  ( 15.06905040192160072, 1513.645442088320124, 194.5599833342589875 ) ) ;
#67733=CARTESIAN_POINT ( 'NONE',  ( -14.86941682237170070, 1514.013728164699842, 194.2615873074070123 ) ) ;
#67760=CARTESIAN_POINT ( 'NONE',  ( 14.44303130513500122, 1516.995662938509895, 192.4521789031669812 ) ) ;
#67770=CARTESIAN_POINT ( 'NONE',  ( 2.298048923505000118, 1516.764084769670262, 212.5672535042169784 ) ) ;
#67809=CARTESIAN_POINT ( 'NONE',  ( 1.569161254424999985, 1517.051704408389924, 201.3992656178269840 ) ) ;
#67816=CARTESIAN_POINT ( 'NONE',  ( 4.027697225915000345, 1516.766397346390022, 206.2431526829570032 ) ) ;
#67817=VECTOR ( 'NONE', #95135, 1000.000000000000227 ) ;
#67826=DIRECTION ( 'NONE',  ( -1.000000000000000000, 0.000000000000000000, 0.000000000000000000 ) ) ;
#67832=CARTESIAN_POINT ( 'NONE',  ( -6.933616859135000254, 1516.548716157039962, 211.4141532006069895 ) ) ;
#67862=CARTESIAN_POINT ( 'NONE',  ( -3.454748846324999789, 1516.609912606490070, 201.7988116581369979 ) ) ;
#67863=CARTESIAN_POINT ( 'NONE',  ( 7.724874613184999461, 1517.139320148880188, 209.8621665372610039 ) ) ;
#67867=CARTESIAN_POINT ( 'NONE',  ( 2.942029629868560203, 1512.314860014990018, 217.0136234555809835 ) ) ;
#67889=CARTESIAN_POINT ( 'NONE',  ( 16.66966702893499885, 1516.995662938509895, 223.5648772753669959 ) ) ;
#67891=CARTESIAN_POINT ( 'NONE',  ( 2.490245914424999985, 1516.691389976299888, 213.7302634767470124 ) ) ;
#67899=PLANE ( 'NONE',  #75502 ) ;
#67909=CARTESIAN_POINT ( 'NONE',  ( -3.461360131404999763, 1516.874084700499907, 205.8683838714370040 ) ) ;
#67916=CARTESIAN_POINT ( 'NONE',  ( 7.012921545624998920, 1508.551704408389924, 214.6352815241970120 ) ) ;
#67926=B_SPLINE_SURFACE_WITH_KNOTS ( 'NONE', 5, 5, ( 
 ( #47600, #12880, #47059, #30226, #81726, #30783 ),
 ( #56557, #6687, #109706, #74472, #16707, #50909 ),
 ( #57120, #68286, #49263, #85040, #108600, #34094 ),
 ( #40288, #110247, #76652, #76107, #57675, #40844 ),
 ( #31888, #8330, #23483, #91790, #75017, #109167 ),
 ( #15066, #22912, #83389, #66074, #110802, #100199 ) ),
 .UNSPECIFIED., .F., .F., .F.,
 ( 6, 6 ),
 ( 6, 6 ),
 ( 4.250940516431640503, 7.082035122218359291 ),
 ( -9.670478362889549828E-06, 0.5000000000000000000 ),
 .UNSPECIFIED. ) ;
#67951=CARTESIAN_POINT ( 'NONE',  ( -5.513240571345160213, 1508.551563895499839, 216.2888651835419864 ) ) ;
#67959=DIRECTION ( 'NONE',  ( 1.643460219210440075E-32, 1.000000000000000000, -6.123233995736769734E-17 ) ) ;
#67961=CARTESIAN_POINT ( 'NONE',  ( 1.123101578415000024, 1517.157901477309906, 203.3331546065870157 ) ) ;
#67970=ORIENTED_EDGE ( 'NONE', *, *, #38482, .F. ) ;
#67988=CARTESIAN_POINT ( 'NONE',  ( 5.706397847405000334, 1514.325389163589989, 201.4706566950069941 ) ) ;
#67997=CARTESIAN_POINT ( 'NONE',  ( 2.873329360754999673, 1516.572193931679976, 216.4439510378570048 ) ) ;
#67998=CARTESIAN_POINT ( 'NONE',  ( -7.887508661103116658, 1512.146863357109623, 212.0793319856411756 ) ) ;
#68005=CARTESIAN_POINT ( 'NONE',  ( 7.321455873725000174, 1516.545806094630279, 206.6359999332069890 ) ) ;
#68011=CARTESIAN_POINT ( 'NONE',  ( 7.569982661595000550, 1513.743447518359972, 215.3638997164470084 ) ) ;
#68021=CARTESIAN_POINT ( 'NONE',  ( 6.556651371285000529, 1516.858146885269889, 215.6747433371770057 ) ) ;
#68024=CARTESIAN_POINT ( 'NONE',  ( -7.720322753056100495, 1516.965532036659852, 209.0131533299550028 ) ) ;
#68025=CARTESIAN_POINT ( 'NONE',  ( -4.608146819384999482, 1516.677239312369920, 211.4179708211670174 ) ) ;
#68044=CARTESIAN_POINT ( 'NONE',  ( -6.556651409415000131, 1516.858146885269889, 202.5689485651570010 ) ) ;
#68064=CARTESIAN_POINT ( 'NONE',  ( -4.115882557953129961, 1509.032029208890208, 213.4860371167349911 ) ) ;
#68066=AXIS2_PLACEMENT_3D ( 'NONE', #53478, #10908, #63544 ) ;
#68123=ORIENTED_EDGE ( 'NONE', *, *, #11208, .T. ) ;
#68128=CARTESIAN_POINT ( 'NONE',  ( -1.704794841465000044, 1517.096587378560116, 213.7484378375869767 ) ) ;
#68135=CARTESIAN_POINT ( 'NONE',  ( 4.031142351675000235, 1516.929569650079884, 204.1114229688670036 ) ) ;
#68143=CARTESIAN_POINT ( 'NONE',  ( -11.12931925038936498, 1512.151624459630966, 193.3374815694428435 ) ) ;
#68152=CARTESIAN_POINT ( 'NONE',  ( -6.546039433425000276, 1516.565291103010168, 211.4147861392469849 ) ) ;
#68156=CARTESIAN_POINT ( 'NONE',  ( 7.326072144144999854, 1516.714320817460020, 208.3685457967989976 ) ) ;
#68157=EDGE_CURVE ( 'NONE', #30294, #49664, #38848, .T. ) ;
#68158=VERTEX_POINT ( 'NONE', #109388 ) ;
#68162=ORIENTED_EDGE ( 'NONE', *, *, #52443, .T. ) ;
#68164=AXIS2_PLACEMENT_3D ( 'NONE', #56059, #47660, #81787 ) ;
#68172=DIRECTION ( 'NONE',  ( -0.000000000000000000, 0.02617694830742909803, 0.9996573249755689172 ) ) ;
#68173=CARTESIAN_POINT ( 'NONE',  ( -0.7365612166329978949, 1517.066898074209803, 213.7457380308570123 ) ) ;
#68176=CARTESIAN_POINT ( 'NONE',  ( 3.260378255074999565, 1516.582197289609894, 216.8321318079170226 ) ) ;
#68180=ORIENTED_EDGE ( 'NONE', *, *, #91161, .F. ) ;
#68250=CARTESIAN_POINT ( 'NONE',  ( -8.160415419918159330, 1511.384673127000042, 214.5167964041220046 ) ) ;
#68256=CARTESIAN_POINT ( 'NONE',  ( -1.715109485185000171, 1516.963431999339946, 208.3866188148990091 ) ) ;
#68266=CARTESIAN_POINT ( 'NONE',  ( -15.27803607861480018, 1512.526687531790003, 222.3611531480509882 ) ) ;
#68286=CARTESIAN_POINT ( 'NONE',  ( -4.119379060793310288, 1508.879004046169939, 204.7521175727229945 ) ) ;
#68288=CARTESIAN_POINT ( 'NONE',  ( -0.01328397755539850039, 1516.939580991450157, 205.8601936452070049 ) ) ;
#68294=VERTEX_POINT ( 'NONE', #75776 ) ;
#68328=AXIS2_PLACEMENT_3D ( 'NONE', #89784, #73561, #38822 ) ;
#68335=CARTESIAN_POINT ( 'NONE',  ( -5.772727946874999461, 1516.691414181030041, 212.5791125756269935 ) ) ;
#68376=CARTESIAN_POINT ( 'NONE',  ( 7.709032137684999952, 1516.534320418310244, 206.6366287381669906 ) ) ;
#68389=CARTESIAN_POINT ( 'NONE',  ( -6.546039433425000276, 1516.565291103010168, 211.4147861392469849 ) ) ;
#68414=CARTESIAN_POINT ( 'NONE',  ( 4.181771622075575401, 1516.718258641771627, 215.3525544691363507 ) ) ;
#68419=CARTESIAN_POINT ( 'NONE',  ( 4.615017327834999961, 1516.987478262539980, 202.5620478758069964 ) ) ;
#68420=CARTESIAN_POINT ( 'NONE',  ( 6.556850996575000146, 1516.939568781210028, 209.1101343261499892 ) ) ;
#68441=CARTESIAN_POINT ( 'NONE',  ( 0.9174002424232758912, 1516.679308524277985, 216.8346747550911573 ) ) ;
#68453=CARTESIAN_POINT ( 'NONE',  ( -16.57141203446500199, 1514.216506490359961, 223.4987549717669992 ) ) ;
#68459=CARTESIAN_POINT ( 'NONE',  ( 4.027051405805000428, 1516.733363207009916, 206.6306575737070261 ) ) ;
#68461=CARTESIAN_POINT ( 'NONE',  ( 7.509380762641779228, 1508.909942010254326, 214.6352815282469351 ) ) ;
#68482=CARTESIAN_POINT ( 'NONE',  ( -13.06907221071063319, 1513.473942842487531, 192.3324832216730442 ) ) ;
#68506=DIRECTION ( 'NONE',  ( -0.7071067811865493491, 0.000000000000000000, -0.7071067811865457964 ) ) ;
#68508=CARTESIAN_POINT ( 'NONE',  ( -0.01244697378919850002, 1516.939646076049939, 203.3402601539570185 ) ) ;
#68512=CARTESIAN_POINT ( 'NONE',  ( 8.568313680894998896, 1512.631076693560090, 221.2256935570670180 ) ) ;
#68514=DIRECTION ( 'NONE',  ( -1.000000000000000000, 0.000000000000000000, 0.000000000000000000 ) ) ;
#68532=CARTESIAN_POINT ( 'NONE',  ( -2.283570671295000132, 1516.909589401870107, 212.0033943946770023 ) ) ;
#68544=CARTESIAN_POINT ( 'NONE',  ( 2.485845998894999909, 1516.545806094630279, 216.4433018439569878 ) ) ;
#68545=CARTESIAN_POINT ( 'NONE',  ( -7.895935239610811784, 1512.041030487407625, 212.1227011107451688 ) ) ;
#68550=CARTESIAN_POINT ( 'NONE',  ( -5.012938901904998801, 1517.051603658920158, 206.6410320471169939 ) ) ;
#68557=CARTESIAN_POINT ( 'NONE',  ( 7.573276829334999682, 1513.355826799109764, 216.9658125846070220 ) ) ;
#68567=CARTESIAN_POINT ( 'NONE',  ( -3.451033427095000050, 1517.025653221279981, 214.9083735325669977 ) ) ;
#68570=CARTESIAN_POINT ( 'NONE',  ( 6.081400497050199583, 1508.610505975320166, 216.4418972163030048 ) ) ;
#68571=CARTESIAN_POINT ( 'NONE',  ( -6.933879441005000643, 1516.560253536979872, 211.6083207129769903 ) ) ;
#68578=CARTESIAN_POINT ( 'NONE',  ( -7.572192888655000509, 1511.308638870219966, 211.6864797536570109 ) ) ;
#68586=CARTESIAN_POINT ( 'NONE',  ( 1.706797785944999868, 1517.164987839469859, 203.3324512698969784 ) ) ;
#68609=CARTESIAN_POINT ( 'NONE',  ( -4.987081080971620395, 1508.551704408389924, 213.0804751642000099 ) ) ;
#68632=EDGE_CURVE ( 'NONE', #61609, #100009, #29775, .T. ) ;
#68646=VERTEX_POINT ( 'NONE', #52108 ) ;
#68656=DIRECTION ( 'NONE',  ( -1.000000000000000000, 0.000000000000000000, 0.000000000000000000 ) ) ;
#68670=CARTESIAN_POINT ( 'NONE',  ( -7.324914956285000223, 1516.685667699390024, 213.7393364370070117 ) ) ;
#68675=EDGE_CURVE ( 'NONE', #58764, #42643, #23421, .T. ) ;
#68677=CARTESIAN_POINT ( 'NONE',  ( 1.123101578415000024, 1517.157901477309906, 203.3331546065870157 ) ) ;
#68690=CARTESIAN_POINT ( 'NONE',  ( -7.709032175815000443, 1516.534320418310244, 211.6070631641669877 ) ) ;
#68696=CARTESIAN_POINT ( 'NONE',  ( -0.01012492377659850000, 1516.989863902050047, 207.9939175986969815 ) ) ;
#68704=ADVANCED_FACE ( 'NONE', ( #92981 ), #51953, .F. ) ;
#68712=CARTESIAN_POINT ( 'NONE',  ( 0.4403324358131759930, 1517.051704035390003, 201.6347831756999938 ) ) ;
#68714=CARTESIAN_POINT ( 'NONE',  ( 2.490245914424999985, 1516.691389976299888, 213.7302634767470124 ) ) ;
#68717=CARTESIAN_POINT ( 'NONE',  ( 3.454119916704999849, 1516.594591938570147, 216.8324563732270178 ) ) ;
#68732=ADVANCED_FACE ( 'NONE', ( #24647 ), #109796, .T. ) ;
#68769=EDGE_CURVE ( 'NONE', #61609, #30006, #6219, .T. ) ;
#68802=CARTESIAN_POINT ( 'NONE',  ( 4.042388501175000037, 1517.045004075700035, 209.8579434088520088 ) ) ;
#68819=CARTESIAN_POINT ( 'NONE',  ( -1.715109485185000171, 1516.963431999339946, 208.3866188148990091 ) ) ;
#68834=CARTESIAN_POINT ( 'NONE',  ( 4.028307740155000261, 1516.797038924770050, 205.8554964580370097 ) ) ;
#68882=ADVANCED_FACE ( 'NONE', ( #71703 ), #20668, .F. ) ;
#68889=CARTESIAN_POINT ( 'NONE',  ( 2.878693249144999466, 1516.766397346390022, 213.1495431961470217 ) ) ;
#68932=CARTESIAN_POINT ( 'NONE',  ( 3.252530615595000452, 1516.827328999679821, 206.2418890071470230 ) ) ;
#68939=VERTEX_POINT ( 'NONE', #31845 ) ;
#68940=CARTESIAN_POINT ( 'NONE',  ( -16.38124167859501412, 1514.407859703122313, 223.7133277291391664 ) ) ;
#68943=AXIS2_PLACEMENT_3D ( 'NONE', #37219, #88729, #71416 ) ;
#68945=CARTESIAN_POINT ( 'NONE',  ( 0.01319650876840149957, 1516.941178807709775, 211.4140629809269853 ) ) ;
#68953=ORIENTED_EDGE ( 'NONE', *, *, #80990, .T. ) ;
#68961=B_SPLINE_CURVE_WITH_KNOTS ( 'NONE', 5,
 ( #23273, #84295, #24374, #110052, #48511, #50167, #15418, #49609, #84828, #57470, #22703, #33326 ),
 .UNSPECIFIED., .F., .F.,
 ( 6, 3, 3, 6 ),
 ( -8.912489289840001661, -7.801458206499999548, -6.062162762929999893, -3.672001930560000460 ),
 .UNSPECIFIED. ) ;
#68973=CARTESIAN_POINT ( 'NONE',  ( 1.123101578415000024, 1517.157901477309906, 203.3331546065870157 ) ) ;
#68974=CARTESIAN_POINT ( 'NONE',  ( 2.873919002525000099, 1516.940252185109784, 209.1085733957019954 ) ) ;
#68975=ORIENTED_EDGE ( 'NONE', *, *, #65076, .F. ) ;
#68977=CARTESIAN_POINT ( 'NONE',  ( 3.215708743572380790, 1511.798530722473515, 217.0753755202089508 ) ) ;
#68997=CARTESIAN_POINT ( 'NONE',  ( -4.487249792034999629, 1509.038615934169911, 205.6342535031670025 ) ) ;
#69009=CARTESIAN_POINT ( 'NONE',  ( -15.09629036526500023, 1514.287526756679881, 224.4071695879669903 ) ) ;
#69014=CARTESIAN_POINT ( 'NONE',  ( -1.136547623115000016, 1516.839862955080207, 206.6438706166370025 ) ) ;
#69034=CARTESIAN_POINT ( 'NONE',  ( 5.726916880756410144, 1510.539524128566654, 216.6663165935511017 ) ) ;
#69067=CARTESIAN_POINT ( 'NONE',  ( -4.618749106614999711, 1516.729202374750002, 202.5720834851169911 ) ) ;
#69087=CARTESIAN_POINT ( 'NONE',  ( 2.942029629868560203, 1512.314860014990018, 217.0136234555809835 ) ) ;
#69088=CARTESIAN_POINT ( 'NONE',  ( 3.462620818104999998, 1516.938330505699923, 211.6001527901769919 ) ) ;
#69091=CARTESIAN_POINT ( 'NONE',  ( 7.382751547855000318, 1511.929989569679947, 202.5109750345870054 ) ) ;
#69092=ORIENTED_EDGE ( 'NONE', *, *, #17874, .F. ) ;
#69100=CARTESIAN_POINT ( 'NONE',  ( 1.708092266164999984, 1516.523379810429788, 216.8305916180169959 ) ) ;
#69108=CARTESIAN_POINT ( 'NONE',  ( -2.493073867885000183, 1516.826109302209943, 206.2575198447970024 ) ) ;
#69109=ORIENTED_EDGE ( 'NONE', *, *, #64845, .T. ) ;
#69112=ORIENTED_EDGE ( 'NONE', *, *, #102190, .T. ) ;
#69121=CARTESIAN_POINT ( 'NONE',  ( -2.287084308194999860, 1517.068517094990057, 214.1351209316169957 ) ) ;
#69127=CARTESIAN_POINT ( 'NONE',  ( 1.136547584984999970, 1516.839862955080207, 211.5998212856970042 ) ) ;
#69128=CARTESIAN_POINT ( 'NONE',  ( 15.01814799273499901, 1514.214451716350140, 223.8476172842669882 ) ) ;
#69143=CARTESIAN_POINT ( 'NONE',  ( -7.334328310795000583, 1517.005755693489846, 204.1179978101270081 ) ) ;
#69197=CARTESIAN_POINT ( 'NONE',  ( 7.477233242777599820, 1510.784366252118843, 202.9987894833095652 ) ) ;
#69218=CARTESIAN_POINT ( 'NONE',  ( 0.01322035751810150123, 1516.939819969850078, 213.1588969678170145 ) ) ;
#69226=CARTESIAN_POINT ( 'NONE',  ( 4.032397901875000024, 1516.981965530290154, 203.3362630185569913 ) ) ;
#69240=EDGE_CURVE ( 'NONE', #72815, #3729, #67480, .T. ) ;
#69243=CARTESIAN_POINT ( 'NONE',  ( 0.01327253640020150012, 1516.940252185109784, 211.9957649727570015 ) ) ;
#69248=CARTESIAN_POINT ( 'NONE',  ( 6.556850996575000146, 1516.939568781210028, 209.1101343261499892 ) ) ;
#69260=DIRECTION ( 'NONE',  ( -0.6768489701308448847, 0.6839977328998089190, 0.2720708970484284062 ) ) ;
#69263=CARTESIAN_POINT ( 'NONE',  ( 0.4354997668961430035, 1517.051704408389924, 201.4383102929800202 ) ) ;
#69265=CARTESIAN_POINT ( 'NONE',  ( -4.030514550714999977, 1516.901952101700090, 213.7446888144170032 ) ) ;
#69268=CARTESIAN_POINT ( 'NONE',  ( 6.942344691835000248, 1516.810037859429940, 216.8380980232070101 ) ) ;
#69271=CARTESIAN_POINT ( 'NONE',  ( 3.454172615424999648, 1517.122088787240045, 201.3974225380069925 ) ) ;
#69306=CARTESIAN_POINT ( 'NONE',  ( -1.902812991693870082, 1516.533218713809902, 201.4128426435650283 ) ) ;
#69333=ORIENTED_EDGE ( 'NONE', *, *, #65330, .F. ) ;
#69344=CARTESIAN_POINT ( 'NONE',  ( -8.555194285240508734, 1511.487508625139981, 214.6892046000639880 ) ) ;
#69352=CARTESIAN_POINT ( 'NONE',  ( 5.786847739675000213, 1517.104497701820037, 209.8595134730280165 ) ) ;
#69361=CARTESIAN_POINT ( 'NONE',  ( -15.30573755027229943, 1512.900351074050150, 222.8919101910120162 ) ) ;
#69371=CARTESIAN_POINT ( 'NONE',  ( 4.028611221114998919, 1516.744381837270112, 207.9874879615069858 ) ) ;
#69389=CARTESIAN_POINT ( 'NONE',  ( -1.135185082175000026, 1516.778853242349896, 205.6747174714770097 ) ) ;
#69392=CARTESIAN_POINT ( 'NONE',  ( -4.181771660003004598, 1516.718258641743432, 202.8911374329507282 ) ) ;
#69395=CARTESIAN_POINT ( 'NONE',  ( 4.487249753905000027, 1509.038615934169911, 212.6094383991670043 ) ) ;
#69399=CARTESIAN_POINT ( 'NONE',  ( 7.065869263262089639, 1517.051704406860154, 213.1971559965600136 ) ) ;
#69412=EDGE_LOOP ( 'NONE', ( #105079, #80582, #42745, #13875, #65088, #33262, #57108, #88744 ) ) ;
#69438=CARTESIAN_POINT ( 'NONE',  ( 6.559798056295000457, 1516.987478262539980, 213.7368632980669929 ) ) ;
#69477=CARTESIAN_POINT ( 'NONE',  ( -3.669386717783980068, 1517.051704642929963, 215.6629163041010031 ) ) ;
#69481=CARTESIAN_POINT ( 'NONE',  ( 1.118104729594999958, 1516.965971551240045, 206.8221779662269739 ) ) ;
#69496=CARTESIAN_POINT ( 'NONE',  ( 0.7574259850960020080, 1516.837969789639828, 212.3776558342370038 ) ) ;
#69508=ADVANCED_FACE ( 'NONE', ( #88563 ), #13882, .F. ) ;
#69526=EDGE_LOOP ( 'NONE', ( #82673, #27519, #76558, #93779 ) ) ;
#69527=CARTESIAN_POINT ( 'NONE',  ( -4.618749106614999711, 1516.729202374750002, 202.5720834851169911 ) ) ;
#69528=CARTESIAN_POINT ( 'NONE',  ( 6.944466742375000834, 1516.939530130779985, 209.1105810159089913 ) ) ;
#69549=CARTESIAN_POINT ( 'NONE',  ( -6.252266492314999979, 1511.741868877540128, 200.3335294429169835 ) ) ;
#69550=ORIENTED_EDGE ( 'NONE', *, *, #45218, .F. ) ;
#69567=CARTESIAN_POINT ( 'NONE',  ( -14.72577135216500110, 1514.214451716350140, 224.1399939629670257 ) ) ;
#69571=CARTESIAN_POINT ( 'NONE',  ( -6.563254928984999736, 1517.139039350860003, 206.6385234782069915 ) ) ;
#69589=CARTESIAN_POINT ( 'NONE',  ( -2.830985251735000485, 1512.320675624280057, 201.3411128641770063 ) ) ;
#69591=ORIENTED_EDGE ( 'NONE', *, *, #27476, .T. ) ;
#69613=CARTESIAN_POINT ( 'NONE',  ( -5.513199828441160300, 1509.038617475689989, 216.6345962050160097 ) ) ;
#69615=CARTESIAN_POINT ( 'NONE',  ( -9.638115897709079505, 1516.551188146539971, 203.7504991310609910 ) ) ;
#69622=CARTESIAN_POINT ( 'NONE',  ( -4.621267922064999922, 1516.830644417779922, 204.1223895416970038 ) ) ;
#69648=CARTESIAN_POINT ( 'NONE',  ( 0.01323701367210150005, 1516.939658295650133, 211.6080660720070341 ) ) ;
#69651=CARTESIAN_POINT ( 'NONE',  ( 7.163002496964999466, 1512.132770473880100, 202.2540665605069705 ) ) ;
#69657=CARTESIAN_POINT ( 'NONE',  ( -6.964055617815001042, 1512.881909847370025, 216.3028661151370216 ) ) ;
#69660=CARTESIAN_POINT ( 'NONE',  ( 5.779603100124999671, 1516.738222552470233, 216.8362174732170047 ) ) ;
#69670=CARTESIAN_POINT ( 'NONE',  ( 2.283570633165000086, 1516.909589401870107, 206.2402975076569760 ) ) ;
#69674=ORIENTED_EDGE ( 'NONE', *, *, #8299, .T. ) ;
#69675=CARTESIAN_POINT ( 'NONE',  ( -5.513203988984379578, 1508.884118749120262, 201.6131408764620119 ) ) ;
#69688=CARTESIAN_POINT ( 'NONE',  ( 5.782749401605000727, 1516.858301627840092, 214.8983370654769942 ) ) ;
#69690=CARTESIAN_POINT ( 'NONE',  ( 6.099947970667409791, 1511.445028088800200, 216.7805665003349986 ) ) ;
#69692=CARTESIAN_POINT ( 'NONE',  ( 3.462620818104999998, 1516.938330505699923, 211.6001527901769919 ) ) ;
#69700=DIRECTION ( 'NONE',  ( 0.02616798426500965835, -0.9993150019883683122, -0.02616798426500960631 ) ) ;
#69701=DIRECTION ( 'NONE',  ( 5.590778865670909642E-17, 1.000000000000000000, 0.000000000000000000 ) ) ;
#69709=CARTESIAN_POINT ( 'NONE',  ( 4.030514512585000375, 1516.901952101700090, 204.4990030879170320 ) ) ;
#69738=CARTESIAN_POINT ( 'NONE',  ( 7.887696381483615404, 1512.266332053796077, 206.1838970189314750 ) ) ;
#69746=CARTESIAN_POINT ( 'NONE',  ( 7.102869657934872905, 1516.552937176199521, 206.7109580197294463 ) ) ;
#69777=ORIENTED_EDGE ( 'NONE', *, *, #34575, .T. ) ;
#69784=CARTESIAN_POINT ( 'NONE',  ( 4.621897824414999967, 1516.858533673840157, 213.7337256555570093 ) ) ;
#69785=CARTESIAN_POINT ( 'NONE',  ( 3.167889818784999978, 1511.297452611750032, 216.7408386441069865 ) ) ;
#69789=CARTESIAN_POINT ( 'NONE',  ( -4.621267922064999922, 1516.830644417779922, 204.1223895416970038 ) ) ;
#69796=CARTESIAN_POINT ( 'NONE',  ( 2.485205649205000089, 1517.181921232829836, 201.3958557702769951 ) ) ;
#69806=CARTESIAN_POINT ( 'NONE',  ( -1.118353254094999860, 1516.977201124959947, 211.6155430111569729 ) ) ;
#69812=CARTESIAN_POINT ( 'NONE',  ( 2.286472886424999906, 1516.883361325900069, 208.3638615500849767 ) ) ;
#69827=CARTESIAN_POINT ( 'NONE',  ( 1.710004548794999968, 1516.557392317769882, 215.6678473207969944 ) ) ;
#69830=CARTESIAN_POINT ( 'NONE',  ( -0.7403206051589980019, 1517.139320148880188, 216.8467205834170102 ) ) ;
#69840=CIRCLE ( 'NONE', #12587, 6.500000000000000000 ) ;
#69864=CARTESIAN_POINT ( 'NONE',  ( -2.431784208376569723, 1516.533929790709863, 201.4128240233619920 ) ) ;
#69913=CARTESIAN_POINT ( 'NONE',  ( 4.044319887224999910, 1517.073005577650065, 210.2423896678870108 ) ) ;
#69930=CARTESIAN_POINT ( 'NONE',  ( 4.612671339784999880, 1516.783665406140017, 208.3654117178780041 ) ) ;
#69932=CARTESIAN_POINT ( 'NONE',  ( -7.460636202991704380, 1509.035273820330531, 215.1586052621513545 ) ) ;
#69935=VERTEX_POINT ( 'NONE', #52490 ) ;
#69945=CARTESIAN_POINT ( 'NONE',  ( 7.709681268295000223, 1516.559109716219837, 206.2491454149069909 ) ) ;
#69948=CARTESIAN_POINT ( 'NONE',  ( -4.327793213831197860, 1516.734711358231152, 202.9907106567216601 ) ) ;
#69966=CARTESIAN_POINT ( 'NONE',  ( 4.039897278065000208, 1516.787536375099990, 214.1203611275269907 ) ) ;
#69997=CARTESIAN_POINT ( 'NONE',  ( -7.323974644434999348, 1516.647924054489977, 213.1579656147470132 ) ) ;
#70013=DIRECTION ( 'NONE',  ( -0.2720708970484284062, 0.6839977328998089190, -0.6768489701308448847 ) ) ;
#70042=CARTESIAN_POINT ( 'NONE',  ( -8.680963252626170856, 1511.446089069276695, 214.5904756146348689 ) ) ;
#70045=CARTESIAN_POINT ( 'NONE',  ( -0.01319654689839849966, 1516.941178807709775, 206.8296289214069930 ) ) ;
#70054=CARTESIAN_POINT ( 'NONE',  ( 8.537822598675001373, 1517.051704408389924, 212.5465662711270056 ) ) ;
#70058=CARTESIAN_POINT ( 'NONE',  ( -7.322105105754999954, 1516.572193931679976, 211.9951753309869957 ) ) ;
#70085=CARTESIAN_POINT ( 'NONE',  ( 6.551643386774999023, 1516.807958722750072, 203.3403553877570005 ) ) ;
#70086=CARTESIAN_POINT ( 'NONE',  ( -5.000330033664999618, 1516.770163853809890, 209.8779366980180328 ) ) ;
#70089=VECTOR ( 'NONE', #49167, 1000.000000000000000 ) ;
#70099=DIRECTION ( 'NONE',  ( 0.02616798426500960631, -0.9993150019883682011, 0.02616798426500970345 ) ) ;
#70133=CARTESIAN_POINT ( 'NONE',  ( -2.493073867885000183, 1516.826109302209943, 206.2575198447970024 ) ) ;
#70151=CARTESIAN_POINT ( 'NONE',  ( -2.822464128215000034, 1512.205735116489905, 201.3478245270569857 ) ) ;
#70177=CARTESIAN_POINT ( 'NONE',  ( -6.725623931370599884, 1508.728101229370168, 216.3255547359810009 ) ) ;
#70189=CARTESIAN_POINT ( 'NONE',  ( -3.264778817514999876, 1516.727068157269969, 204.1245957781970048 ) ) ;
#70190=CARTESIAN_POINT ( 'NONE',  ( 15.62010807923499911, 1514.600163677630007, 193.7548396194670204 ) ) ;
#70213=CARTESIAN_POINT ( 'NONE',  ( -3.446329813785000251, 1516.812046502680005, 212.0014881234369852 ) ) ;
#70223=CARTESIAN_POINT ( 'NONE',  ( -8.473068926205000295, 1511.778199792620171, 215.2106786806170078 ) ) ;
#70233=CARTESIAN_POINT ( 'NONE',  ( -3.462620856235000044, 1516.938330505699923, 206.6435391121569864 ) ) ;
#70238=CARTESIAN_POINT ( 'NONE',  ( -7.260552783093170426, 1508.878902882709781, 202.3557464436360078 ) ) ;
#70248=CARTESIAN_POINT ( 'NONE',  ( -1.123101616545000070, 1517.157901477309906, 214.9105372957470195 ) ) ;
#70250=CARTESIAN_POINT ( 'NONE',  ( 5.586203231419629489, 1511.461696079649982, 217.8427964110400126 ) ) ;
#70252=CARTESIAN_POINT ( 'NONE',  ( -3.253141175365000137, 1516.858171774179937, 212.3894494859370070 ) ) ;
#70269=CARTESIAN_POINT ( 'NONE',  ( 5.775236792744999903, 1516.804776704140068, 204.1142572851869943 ) ) ;
#70297=CARTESIAN_POINT ( 'NONE',  ( 7.887474265800920037, 1512.146734774960350, 206.1643637411737302 ) ) ;
#70310=CARTESIAN_POINT ( 'NONE',  ( 6.554778533645000849, 1516.929962200689943, 201.4024535497269994 ) ) ;
#70314=CARTESIAN_POINT ( 'NONE',  ( 7.583791906034999641, 1511.751588929339960, 206.7961148284170179 ) ) ;
#70339=ORIENTED_EDGE ( 'NONE', *, *, #29001, .F. ) ;
#70342=CARTESIAN_POINT ( 'NONE',  ( 3.264778779384999829, 1516.727068157269969, 214.1190961241369735 ) ) ;
#70343=CARTESIAN_POINT ( 'NONE',  ( 4.820945208375000846, 1510.984078637139874, 216.7915721300269638 ) ) ;
#70348=CARTESIAN_POINT ( 'NONE',  ( 5.776491095245000373, 1516.858301627840092, 203.3390965304970166 ) ) ;
#70353=CARTESIAN_POINT ( 'NONE',  ( 5.779627054084999216, 1516.977993847330026, 201.4011957967969977 ) ) ;
#70362=CARTESIAN_POINT ( 'NONE',  ( 6.950214933285000285, 1517.129577905929864, 211.9934263588270085 ) ) ;
#70367=CARTESIAN_POINT ( 'NONE',  ( 5.006259848694999626, 1516.939723362869927, 209.1089481433290018 ) ) ;
#70373=ORIENTED_EDGE ( 'NONE', *, *, #87314, .T. ) ;
#70382=CARTESIAN_POINT ( 'NONE',  ( 7.719392382375000139, 1516.929962200689943, 215.6766245038770080 ) ) ;
#70406=CYLINDRICAL_SURFACE ( 'NONE', #78585, 0.9999999999999988898 ) ;
#70464=CARTESIAN_POINT ( 'NONE',  ( 2.297629621054999571, 1516.970035769810011, 209.8568691683980205 ) ) ;
#70481=CARTESIAN_POINT ( 'NONE',  ( -6.564578723344999922, 1517.199196846569976, 207.4137433428170141 ) ) ;
#70500=CARTESIAN_POINT ( 'NONE',  ( -5.788097265284999793, 1517.099836525840146, 206.6397780718770036 ) ) ;
#70519=CARTESIAN_POINT ( 'NONE',  ( -7.323974644434999348, 1516.647924054489977, 213.1579656147470132 ) ) ;
#70570=ORIENTED_EDGE ( 'NONE', *, *, #88439, .T. ) ;
#70588=CARTESIAN_POINT ( 'NONE',  ( -1.136547623115000016, 1516.839862955080207, 206.6438706166370025 ) ) ;
#70600=CARTESIAN_POINT ( 'NONE',  ( 3.268235720634999897, 1516.890356958860139, 211.9874346545169885 ) ) ;
#70610=CARTESIAN_POINT ( 'NONE',  ( 15.09731849065486387, 1514.821748426677459, 225.1372258183207862 ) ) ;
#70612=ORIENTED_EDGE ( 'NONE', *, *, #57263, .T. ) ;
#70617=ORIENTED_EDGE ( 'NONE', *, *, #34951, .F. ) ;
#70631=CARTESIAN_POINT ( 'NONE',  ( -4.036748876935000396, 1516.667393516340098, 202.1854475764570225 ) ) ;
#70632=CARTESIAN_POINT ( 'NONE',  ( -6.550870182235000172, 1516.727502608469877, 209.8762341530540141 ) ) ;
#70655=APPLICATION_CONTEXT ( 'automotive_design' ) ;
#70657=CARTESIAN_POINT ( 'NONE',  ( -7.213837406734999291, 1512.784460098840100, 202.2559763233970216 ) ) ;
#70673=CARTESIAN_POINT ( 'NONE',  ( 11.35635713053500062, 1512.376261820769969, 225.3263167562670048 ) ) ;
#70683=CARTESIAN_POINT ( 'NONE',  ( 7.709032137684999952, 1516.534320418310244, 206.6366287381669906 ) ) ;
#70702=CARTESIAN_POINT ( 'NONE',  ( -2.701540413345000058, 1511.422242621320265, 201.5466790130070081 ) ) ;
#70738=CARTESIAN_POINT ( 'NONE',  ( 6.936398355645000180, 1516.667393516340098, 205.0850970932970085 ) ) ;
#70755=EDGE_CURVE ( 'NONE', #98379, #42497, #93929, .T. ) ;
#70759=CARTESIAN_POINT ( 'NONE',  ( 5.011678838024999472, 1516.989560013210166, 212.3778133565769792 ) ) ;
#70771=CARTESIAN_POINT ( 'NONE',  ( -7.503873141484999287, 1512.035910181040208, 215.6868223634869821 ) ) ;
#70781=CARTESIAN_POINT ( 'NONE',  ( -0.7579844201469989606, 1516.883361325900069, 206.8353730456769881 ) ) ;
#70800=CARTESIAN_POINT ( 'NONE',  ( 3.261635932824999973, 1516.613881697390070, 216.0569793506570022 ) ) ;
#70804=CARTESIAN_POINT ( 'NONE',  ( 5.689538361743419870, 1510.689985724130111, 216.6800952772849769 ) ) ;
#70805=CARTESIAN_POINT ( 'NONE',  ( -3.487592467065000257, 1509.038615934169911, 213.6090957241370063 ) ) ;
#70806=CARTESIAN_POINT ( 'NONE',  ( -7.322105105754999954, 1516.572193931679976, 211.9951753309869957 ) ) ;
#70808=CARTESIAN_POINT ( 'NONE',  ( -14.44303134326499993, 1516.995662938509895, 225.7915129991669971 ) ) ;
#70824=CARTESIAN_POINT ( 'NONE',  ( -6.557909920764999789, 1516.908489800550115, 203.3441005368270282 ) ) ;
#70857=ORIENTED_EDGE ( 'NONE', *, *, #89633, .F. ) ;
#70865=CARTESIAN_POINT ( 'NONE',  ( 4.616899834755000320, 1517.050041317280147, 201.3993091674070115 ) ) ;
#70874=ORIENTED_EDGE ( 'NONE', *, *, #918, .F. ) ;
#70879=CARTESIAN_POINT ( 'NONE',  ( -7.853884020855000259, 1511.558654537720031, 212.4889000995470099 ) ) ;
#70897=CARTESIAN_POINT ( 'NONE',  ( 1.132949076425000090, 1516.693851263360102, 214.1195642086070166 ) ) ;
#70898=CARTESIAN_POINT ( 'NONE',  ( 5.160317800795000132, 1510.729589429620091, 216.6788758775169867 ) ) ;
#70899=ORIENTED_EDGE ( 'NONE', *, *, #90545, .T. ) ;
#70904=CARTESIAN_POINT ( 'NONE',  ( 4.029572640705000985, 1516.858649670339901, 205.0803734583570019 ) ) ;
#70908=CARTESIAN_POINT ( 'NONE',  ( -1.128757599205000073, 1516.608208975040043, 201.4108789544669946 ) ) ;
#70921=CARTESIAN_POINT ( 'NONE',  ( 7.337793712495000342, 1517.145312756229941, 211.9940546803969994 ) ) ;
#70927=CARTESIAN_POINT ( 'NONE',  ( 2.491655725414999800, 1516.977504706749869, 209.8569557413499922 ) ) ;
#70940=CARTESIAN_POINT ( 'NONE',  ( -0.7376675409259989546, 1517.104497701820037, 214.9086937099069985 ) ) ;
#70979=CARTESIAN_POINT ( 'NONE',  ( -15.20279846676549873, 1514.921193439789931, 193.2119408159660168 ) ) ;
#70980=CARTESIAN_POINT ( 'NONE',  ( -1.518801255529869998, 1516.566488792059999, 201.4119714359050022 ) ) ;
#71004=VERTEX_POINT ( 'NONE', #110477 ) ;
#71021=CARTESIAN_POINT ( 'NONE',  ( 7.339107202615000602, 1517.203017563489766, 210.2473558205170150 ) ) ;
#71036=CARTESIAN_POINT ( 'NONE',  ( 2.286472886424999906, 1516.883361325900069, 208.3638615500849767 ) ) ;
#71053=CARTESIAN_POINT ( 'NONE',  ( -1.716392779905000054, 1516.788317650260069, 206.2580580763669786 ) ) ;
#71071=CARTESIAN_POINT ( 'NONE',  ( 1.131796810615000037, 1516.659138130710289, 214.8948242487770131 ) ) ;
#71079=EDGE_CURVE ( 'NONE', #36663, #23166, #12965, .T. ) ;
#71091=VECTOR ( 'NONE', #93737, 1000.000000000000114 ) ;
#71096=VECTOR ( 'NONE', #50309, 1000.000000000000227 ) ;
#71120=AXIS2_PLACEMENT_3D ( 'NONE', #85791, #49456, #41031 ) ;
#71136=CARTESIAN_POINT ( 'NONE',  ( -6.729604382136518126, 1516.629170255225063, 212.4376854727360922 ) ) ;
#71140=CARTESIAN_POINT ( 'NONE',  ( 6.546302742015000398, 1516.577434278289957, 206.6347425125669872 ) ) ;
#71147=VERTEX_POINT ( 'NONE', #71284 ) ;
#71152=CARTESIAN_POINT ( 'NONE',  ( 0.01327253640020150012, 1516.940252185109784, 211.9957649727570015 ) ) ;
#71160=CARTESIAN_POINT ( 'NONE',  ( 12.01214636615307185, 1513.042027792501813, 225.7134143163021918 ) ) ;
#71162=ORIENTED_EDGE ( 'NONE', *, *, #108264, .T. ) ;
#71163=VERTEX_POINT ( 'NONE', #98080 ) ;
#71180=CARTESIAN_POINT ( 'NONE',  ( 3.449149195745000007, 1516.947419719950176, 204.4980579627370219 ) ) ;
#71183=CARTESIAN_POINT ( 'NONE',  ( 5.385523159618170297, 1511.435001054559962, 217.7746220610370074 ) ) ;
#71202=CARTESIAN_POINT ( 'NONE',  ( -8.027449309594999249, 1514.605246816799763, 202.6315394120669851 ) ) ;
#71218=CARTESIAN_POINT ( 'NONE',  ( 11.74940789013500009, 1512.456207068040158, 225.5877689890670013 ) ) ;
#71228=CARTESIAN_POINT ( 'NONE',  ( 6.933587655514999781, 1516.542957540330008, 207.4124872689769745 ) ) ;
#71237=B_SPLINE_CURVE_WITH_KNOTS ( 'NONE', 3,
 ( #3881, #79469, #55375, #10042, #105780, #35806, #63778, #61574, #36899, #54287 ),
 .UNSPECIFIED., .F., .F.,
 ( 4, 2, 2, 2, 4 ),
 ( 0.000000000000000000, 0.2500000000000000000, 0.5000000000000000000, 0.7500000000000000000, 1.000000000000000000 ),
 .UNSPECIFIED. ) ;
#71248=CARTESIAN_POINT ( 'NONE',  ( 5.980914351475993485, 1510.675349056919458, 216.6316662786656764 ) ) ;
#71284=CARTESIAN_POINT ( 'NONE',  ( 17.17760792425680094, 1517.051704368240053, 222.7507317666290305 ) ) ;
#71292=CARTESIAN_POINT ( 'NONE',  ( -7.721907926364999675, 1517.026025493960105, 204.1173703575669833 ) ) ;
#71312=CARTESIAN_POINT ( 'NONE',  ( 5.011367946795000528, 1516.974592746400049, 212.5716232859570027 ) ) ;
#71324=CARTESIAN_POINT ( 'NONE',  ( -7.777075051915000259, 1512.220794350760116, 215.6496765134470195 ) ) ;
#71325=CARTESIAN_POINT ( 'NONE',  ( 16.48452149413872547, 1514.266850628232305, 194.7220678386542261 ) ) ;
#71335=CARTESIAN_POINT ( 'NONE',  ( -0.7579263249019989601, 1516.927039499179955, 207.4176752179770347 ) ) ;
#71354=CARTESIAN_POINT ( 'NONE',  ( -4.615644842514999624, 1517.009964551830080, 216.0692237534070159 ) ) ;
#71357=CARTESIAN_POINT ( 'NONE',  ( 6.265221788440870299, 1511.198033794599951, 216.5696572527920125 ) ) ;
#71360=CARTESIAN_POINT ( 'NONE',  ( -2.283570671295000132, 1516.909589401870107, 212.0033943946770023 ) ) ;
#71379=CARTESIAN_POINT ( 'NONE',  ( -3.458526536014999930, 1516.742629295279812, 204.1242721449069961 ) ) ;
#71414=VERTEX_POINT ( 'NONE', #64923 ) ;
#71416=DIRECTION ( 'NONE',  ( -0.4025563316115431389, 0.03449475076686812219, -0.9147450530333514074 ) ) ;
#71419=CARTESIAN_POINT ( 'NONE',  ( -12.56945278516500153, 1512.044075975079977, 193.8624433630670012 ) ) ;
#71423=CARTESIAN_POINT ( 'NONE',  ( -3.260378293205000055, 1516.582197289609894, 201.4115600944169842 ) ) ;
#71450=VERTEX_POINT ( 'NONE', #98495 ) ;
#71458=AXIS2_PLACEMENT_3D ( 'NONE', #99795, #4123, #66244 ) ;
#71460=CARTESIAN_POINT ( 'NONE',  ( -2.869693497065000098, 1517.070197312179971, 214.9093229647470196 ) ) ;
#71461=CARTESIAN_POINT ( 'NONE',  ( 2.392017048025000037, 1512.336926113599930, 216.7209653789669801 ) ) ;
#71466=CARTESIAN_POINT ( 'NONE',  ( -0.7568987378019988999, 1516.805675336850072, 205.0906771642370074 ) ) ;
#71468=FACE_OUTER_BOUND ( 'NONE', #100509, .T. ) ;
#71477=CARTESIAN_POINT ( 'NONE',  ( 4.041472473744999405, 1516.858649670339901, 213.1514186109370144 ) ) ;
#71478=AXIS2_PLACEMENT_3D ( 'NONE', #51067, #96927, #11810 ) ;
#71483=CARTESIAN_POINT ( 'NONE',  ( 4.618583391875000110, 1516.939762005280045, 209.1087859301640322 ) ) ;
#71491=FACE_OUTER_BOUND ( 'NONE', #51288, .T. ) ;
#71500=CARTESIAN_POINT ( 'NONE',  ( -7.714371541114999786, 1516.738222552470233, 214.9014490703569891 ) ) ;
#71501=CARTESIAN_POINT ( 'NONE',  ( -7.709253412061816135, 1516.542698385629819, 211.7357737058638918 ) ) ;
#71505=CARTESIAN_POINT ( 'NONE',  ( -0.01010286742719850028, 1516.939452820819952, 201.4022050290969901 ) ) ;
#71511=CARTESIAN_POINT ( 'NONE',  ( 8.769368648193829330, 1511.501844456730169, 203.3371675829959884 ) ) ;
#71526=DIRECTION ( 'NONE',  ( 0.000000000000000000, -6.123233995736799316E-17, -1.000000000000000000 ) ) ;
#71560=DIRECTION ( 'NONE',  ( 0.000000000000000000, -1.000000000000000000, 6.123233995736769734E-17 ) ) ;
#71586=CARTESIAN_POINT ( 'NONE',  ( -2.282301616165000269, 1516.836638729160086, 210.8392784184970026 ) ) ;
#71588=EDGE_CURVE ( 'NONE', #21389, #71450, #93148, .T. ) ;
#71595=ADVANCED_FACE ( 'NONE', ( #33241 ), #8039, .F. ) ;
#71596=CARTESIAN_POINT ( 'NONE',  ( 2.484577657225000014, 1517.170512887980067, 201.7834339727070017 ) ) ;
#71601=CARTESIAN_POINT ( 'NONE',  ( 2.879318417774999972, 1516.995911393979895, 209.8571825100049750 ) ) ;
#71613=CARTESIAN_POINT ( 'NONE',  ( -5.614653854145000622, 1512.903985260039917, 216.7358144361969892 ) ) ;
#71618=CARTESIAN_POINT ( 'NONE',  ( 6.546039395294999785, 1516.565291103010168, 206.8289057630870218 ) ) ;
#71621=CARTESIAN_POINT ( 'NONE',  ( -2.282008387128519278, 1516.544479074504125, 201.9748403303481439 ) ) ;
#71635=CARTESIAN_POINT ( 'NONE',  ( -1.124289693584999972, 1517.184063036290127, 215.6857614941170027 ) ) ;
#71636=CARTESIAN_POINT ( 'NONE',  ( -6.500000019064997581, 1516.051704408390151, 209.1218459511669892 ) ) ;
#71687=AXIS2_PLACEMENT_3D ( 'NONE', #76734, #25758, #25202 ) ;
#71703=FACE_OUTER_BOUND ( 'NONE', #54264, .T. ) ;
#71709=CARTESIAN_POINT ( 'NONE',  ( -5.788097265284999793, 1517.099836525840146, 206.6397780718770036 ) ) ;
#71729=CARTESIAN_POINT ( 'NONE',  ( 14.63129139947360891, 1514.438069594173157, 225.4795426202890383 ) ) ;
#71746=ORIENTED_EDGE ( 'NONE', *, *, #8584, .T. ) ;
#71747=CARTESIAN_POINT ( 'NONE',  ( -1.712644754285000070, 1516.636036526019780, 204.1262224792070015 ) ) ;
#71750=CARTESIAN_POINT ( 'NONE',  ( 5.551188674472009588, 1510.480349264700180, 216.6723492941099778 ) ) ;
#71758=LINE ( 'NONE', #54925, #15364 ) ;
#71768=CARTESIAN_POINT ( 'NONE',  ( -7.496083208854999569, 1513.333000339830051, 202.7317914838369859 ) ) ;
#71783=CARTESIAN_POINT ( 'NONE',  ( 15.28532361773500092, 1514.287526756679881, 224.2181362973670105 ) ) ;
#71791=CARTESIAN_POINT ( 'NONE',  ( 4.995623452895000760, 1516.636036526019780, 207.4092012159470073 ) ) ;
#71811=CARTESIAN_POINT ( 'NONE',  ( 6.150246115290385340, 1510.808998940108040, 216.5916852012511811 ) ) ;
#71822=COLOUR_RGB ( '', 0.72549020, 0.75294118, 0.79215686) ;
#71840=CARTESIAN_POINT ( 'NONE',  ( -5.614653854145000622, 1512.903985260039917, 201.5078774661370176 ) ) ;
#71850=CARTESIAN_POINT ( 'NONE',  ( -5.009478105444999940, 1516.886345593249871, 204.5093386581970094 ) ) ;
#71864=CARTESIAN_POINT ( 'NONE',  ( -5.371346839175000554, 1516.551704408390151, 218.7599618298069970 ) ) ;
#71871=CARTESIAN_POINT ( 'NONE',  ( 1.715704490974999885, 1516.757508073510053, 212.3732403323669757 ) ) ;
#71879=VERTEX_POINT ( 'NONE', #69087 ) ;
#71880=CARTESIAN_POINT ( 'NONE',  ( -6.557434894264999592, 1513.513616978030086, 216.5800176418070180 ) ) ;
#71891=CARTESIAN_POINT ( 'NONE',  ( -1.137296688934999800, 1516.908147884120126, 207.4199954749970232 ) ) ;
#71896=CARTESIAN_POINT ( 'NONE',  ( -7.012530104786800500, 1508.551704607450120, 203.1375064762430043 ) ) ;
#71900=CARTESIAN_POINT ( 'NONE',  ( 14.95092670185879946, 1512.169469372310004, 196.6644221003890038 ) ) ;
#71902=FACE_OUTER_BOUND ( 'NONE', #47120, .T. ) ;
#71908=CARTESIAN_POINT ( 'NONE',  ( -3.258474617075000079, 1517.083030555940013, 215.6838419306269827 ) ) ;
#71910=CARTESIAN_POINT ( 'NONE',  ( 5.718152469055599596, 1511.533951550999973, 217.5449680129780177 ) ) ;
#71912=CARTESIAN_POINT ( 'NONE',  ( 0.7576635334400020350, 1516.855632454399938, 211.9899581013969794 ) ) ;
#71918=DIRECTION ( 'NONE',  ( 0.9996573249755574819, -0.02617694830786557875, 0.000000000000000000 ) ) ;
#71932=CARTESIAN_POINT ( 'NONE',  ( -3.265407155974999753, 1516.754149861460064, 204.5121726906670006 ) ) ;
#71965=CARTESIAN_POINT ( 'NONE',  ( -13.59434826296499921, 1512.526319173689899, 193.1055684605670137 ) ) ;
#71976=ORIENTED_EDGE ( 'NONE', *, *, #13146, .F. ) ;
#71981=CARTESIAN_POINT ( 'NONE',  ( -8.072094066334999596, 1511.572472350439739, 212.7333085737770091 ) ) ;
#72000=CARTESIAN_POINT ( 'NONE',  ( 6.557909882634999299, 1516.908489800550115, 214.8995913655070069 ) ) ;
#72001=CARTESIAN_POINT ( 'NONE',  ( 5.139225450924999272, 1511.037966505499980, 216.8073032440570103 ) ) ;
#72007=CARTESIAN_POINT ( 'NONE',  ( -2.296124889065000119, 1516.677239312369920, 204.5136991508470032 ) ) ;
#72014=DIRECTION ( 'NONE',  ( 0.000000000000000000, -1.000000000000000000, 6.123233995736769734E-17 ) ) ;
#72019=CARTESIAN_POINT ( 'NONE',  ( 3.460101851884999746, 1516.812923327049930, 213.1504765548870068 ) ) ;
#72027=CARTESIAN_POINT ( 'NONE',  ( 3.460866170685000132, 1517.020847257979995, 209.8575449048190080 ) ) ;
#72033=EDGE_LOOP ( 'NONE', ( #69333, #105773, #28439, #51780 ) ) ;
#72041=CARTESIAN_POINT ( 'NONE',  ( 1.131796810615000037, 1516.659138130710289, 214.8948242487770131 ) ) ;
#72042=CARTESIAN_POINT ( 'NONE',  ( 4.329791490734999471, 1515.051704408389924, 212.4519801359869859 ) ) ;
#72046=CARTESIAN_POINT ( 'NONE',  ( 2.484577657225000014, 1517.170512887980067, 201.7834339727070017 ) ) ;
#72053=EDGE_CURVE ( 'NONE', #89980, #71879, #32194, .T. ) ;
#72070=LINE ( 'NONE', #46855, #45355 ) ;
#72084=CARTESIAN_POINT ( 'NONE',  ( 13.58541694415399981, 1512.759354980459875, 224.4342445094760023 ) ) ;
#72124=CARTESIAN_POINT ( 'NONE',  ( -7.708745685915000756, 1516.523379810429788, 210.8299382363969983 ) ) ;
#72131=CARTESIAN_POINT ( 'NONE',  ( 6.554151426245000245, 1516.906641539930206, 201.7900338461269882 ) ) ;
#72153=CARTESIAN_POINT ( 'NONE',  ( 2.476733476015000157, 1516.858326417339867, 206.6281461634669938 ) ) ;
#72158=LINE ( 'NONE', #99505, #15881 ) ;
#72159=EDGE_CURVE ( 'NONE', #14138, #71450, #19020, .T. ) ;
#72170=CARTESIAN_POINT ( 'NONE',  ( -2.482067898354999969, 1517.099836525840146, 214.9099431973869798 ) ) ;
#72172=CARTESIAN_POINT ( 'NONE',  ( 7.709937712299099744, 1516.568902917619880, 207.6216162931799829 ) ) ;
#72211=LINE ( 'NONE', #63803, #65516 ) ;
#72213=CARTESIAN_POINT ( 'NONE',  ( -3.915803421951532748, 1515.051704408389924, 213.4516362061156656 ) ) ;
#72224=CARTESIAN_POINT ( 'NONE',  ( -7.444963660044519926, 1508.731180391400130, 214.6350537475119893 ) ) ;
#72235=CARTESIAN_POINT ( 'NONE',  ( 3.251394362135000105, 1516.757508073510053, 207.4061414411269766 ) ) ;
#72246=CARTESIAN_POINT ( 'NONE',  ( -5.513435588854999736, 1508.551704408389924, 216.1347675159770176 ) ) ;
#72253=CARTESIAN_POINT ( 'NONE',  ( 15.20279842864010078, 1514.921193439799936, 225.0317510863630162 ) ) ;
#72268=CARTESIAN_POINT ( 'NONE',  ( 3.255967386345000047, 1516.989560013210166, 204.1101670940770134 ) ) ;
#72282=CARTESIAN_POINT ( 'NONE',  ( 6.252266454184999489, 1511.741868877540128, 217.9101624594169948 ) ) ;
#72284=VECTOR ( 'NONE', #104061, 1000.000000000000114 ) ;
#72290=CARTESIAN_POINT ( 'NONE',  ( -6.843878254575000319, 1512.371933174370042, 200.6190499138870109 ) ) ;
#72307=CARTESIAN_POINT ( 'NONE',  ( 13.32051254013499886, 1512.868709057579963, 225.8700958719669813 ) ) ;
#72314=CARTESIAN_POINT ( 'NONE',  ( -3.462948834675000143, 1516.956048353049937, 206.8373194734570006 ) ) ;
#72337=ORIENTED_EDGE ( 'NONE', *, *, #25305, .F. ) ;
#72370=CARTESIAN_POINT ( 'NONE',  ( 2.478306819944999795, 1516.938330505699923, 205.6592251139969960 ) ) ;
#72385=CARTESIAN_POINT ( 'NONE',  ( 5.013429356055000063, 1517.123342927159911, 210.2437967141769946 ) ) ;
#72400=CARTESIAN_POINT ( 'NONE',  ( 16.35769667426164986, 1514.438069564495208, 194.4905545724909075 ) ) ;
#72412=CARTESIAN_POINT ( 'NONE',  ( -6.563595907815000352, 1517.154223579619838, 206.8322214998769937 ) ) ;
#72413=EDGE_LOOP ( 'NONE', ( #92919, #79318, #18615, #22306 ) ) ;
#72429=CARTESIAN_POINT ( 'NONE',  ( 0.01126491619350150110, 1516.939530130779985, 216.0663127125970107 ) ) ;
#72430=LINE ( 'NONE', #55084, #87374 ) ;
#72434=CARTESIAN_POINT ( 'NONE',  ( -3.253462098795000035, 1516.874084700499907, 212.5832060635069922 ) ) ;
#72452=CARTESIAN_POINT ( 'NONE',  ( -4.621897862544999569, 1516.858533673840157, 204.5099662467769974 ) ) ;
#72475=CARTESIAN_POINT ( 'NONE',  ( 8.394745799167832701, 1511.398924905634203, 204.5081796389210638 ) ) ;
#72483=VECTOR ( 'NONE', #84618, 1000.000000000000114 ) ;
#72486=CARTESIAN_POINT ( 'NONE',  ( -14.32514194706499921, 1513.248517198770060, 192.8985536356669854 ) ) ;
#72487=LINE ( 'NONE', #37775, #51978 ) ;
#72489=CARTESIAN_POINT ( 'NONE',  ( 4.035536225084999984, 1517.086065052259983, 201.3983658527070020 ) ) ;
#72493=CARTESIAN_POINT ( 'NONE',  ( 7.683494238625000250, 1512.058324472099912, 206.4100757371070074 ) ) ;
#72501=CARTESIAN_POINT ( 'NONE',  ( -3.454119954913678292, 1516.594591940487589, 201.4112355775968126 ) ) ;
#72504=CARTESIAN_POINT ( 'NONE',  ( -7.549016801754999229, 1510.423579818969984, 213.5498276941069946 ) ) ;
#72518=ORIENTED_EDGE ( 'NONE', *, *, #20517, .T. ) ;
#72523=CARTESIAN_POINT ( 'NONE',  ( 0.01244693565920149993, 1516.939646076049939, 214.9034317483770167 ) ) ;
#72531=CARTESIAN_POINT ( 'NONE',  ( -5.784638357945000031, 1516.939574742129935, 204.5080835752170003 ) ) ;
#72544=CARTESIAN_POINT ( 'NONE',  ( 2.492130623175000448, 1516.778761582560037, 212.5675310476169955 ) ) ;
#72550=CARTESIAN_POINT ( 'NONE',  ( -7.709003326667110301, 1516.533218713809902, 211.0246589237959824 ) ) ;
#72551=CARTESIAN_POINT ( 'NONE',  ( 3.455495833855000143, 1516.939877939420057, 209.1085718841020196 ) ) ;
#72566=CARTESIAN_POINT ( 'NONE',  ( 1.130002494264999990, 1516.621991115350056, 216.0576472317669925 ) ) ;
#72571=CARTESIAN_POINT ( 'NONE',  ( -7.718134667564999774, 1516.881930554049859, 201.7919159189069944 ) ) ;
#72572=CARTESIAN_POINT ( 'NONE',  ( -16.23061969806499860, 1512.609537213029853, 220.4047961632670081 ) ) ;
#72607=CARTESIAN_POINT ( 'NONE',  ( 13.31081193891139947, 1512.571279492530039, 224.4121312145439902 ) ) ;
#72650=VERTEX_POINT ( 'NONE', #84214 ) ;
#72652=CARTESIAN_POINT ( 'NONE',  ( 0.01319650876840149957, 1516.941178807709775, 211.4140629809269853 ) ) ;
#72659=EDGE_CURVE ( 'NONE', #37652, #68294, #82745, .T. ) ;
#72660=CARTESIAN_POINT ( 'NONE',  ( 3.260357128764999946, 1517.133889586189980, 201.3971135232069969 ) ) ;
#72676=CARTESIAN_POINT ( 'NONE',  ( -4.028611259245000298, 1516.744381837270112, 210.2562039408269925 ) ) ;
#72683=CARTESIAN_POINT ( 'NONE',  ( 7.685457273825000435, 1511.037966505489976, 203.9826204811770083 ) ) ;
#72685=CARTESIAN_POINT ( 'NONE',  ( 4.027051405805000428, 1516.733363207009916, 206.6306575737070261 ) ) ;
#72701=CARTESIAN_POINT ( 'NONE',  ( 2.488360629304999794, 1516.616791731099966, 214.8929950451170043 ) ) ;
#72703=CARTESIAN_POINT ( 'NONE',  ( 7.709266964192710070, 1516.543288080860066, 207.3768922116219926 ) ) ;
#72732=CARTESIAN_POINT ( 'NONE',  ( -4.678155188338201320, 1508.611350403811230, 212.6094318194185746 ) ) ;
#72735=EDGE_CURVE ( 'NONE', #110691, #56739, #21939, .T. ) ;
#72741=ORIENTED_EDGE ( 'NONE', *, *, #59405, .T. ) ;
#72744=CARTESIAN_POINT ( 'NONE',  ( 3.487584963630629087, 1508.551704408609794, 213.9544627601069351 ) ) ;
#72767=CARTESIAN_POINT ( 'NONE',  ( -8.641402442529509287, 1511.681013979509999, 215.1708878290160101 ) ) ;
#72772=CARTESIAN_POINT ( 'NONE',  ( -3.463767296015000330, 1517.014196759610059, 207.4190915607570105 ) ) ;
#72792=ORIENTED_EDGE ( 'NONE', *, *, #98337, .T. ) ;
#72802=CARTESIAN_POINT ( 'NONE',  ( 4.833437623558549667, 1508.551704408389924, 205.2117058254140147 ) ) ;
#72811=CARTESIAN_POINT ( 'NONE',  ( -2.875850132345000087, 1516.647618671360078, 203.3500485059169876 ) ) ;
#72815=VERTEX_POINT ( 'NONE', #9024 ) ;
#72832=CARTESIAN_POINT ( 'NONE',  ( -6.681558948264999742, 1511.816633140270142, 201.8377905138470112 ) ) ;
#72846=CARTESIAN_POINT ( 'NONE',  ( 13.56546623563500020, 1512.571022561229938, 224.6914189826670167 ) ) ;
#72847=CARTESIAN_POINT ( 'NONE',  ( -15.90990259576500065, 1516.814170398969964, 224.3246417466669982 ) ) ;
#72853=CARTESIAN_POINT ( 'NONE',  ( 3.445407533985000104, 1516.764084769670262, 206.8237970085970119 ) ) ;
#72899=CARTESIAN_POINT ( 'NONE',  ( -3.699374228837535306, 1511.553914496345442, 201.0215753219823114 ) ) ;
#72902=CARTESIAN_POINT ( 'NONE',  ( -8.359890808884999913, 1517.051704408389924, 205.8920033474969955 ) ) ;
#72908=CARTESIAN_POINT ( 'NONE',  ( 2.284526458645000258, 1516.956048353049937, 205.6588971355569981 ) ) ;
#72924=CARTESIAN_POINT ( 'NONE',  ( -6.550870182235000172, 1516.727502608469877, 209.8762341530540141 ) ) ;
#72936=CARTESIAN_POINT ( 'NONE',  ( -5.818574493064999409, 1514.487275757750012, 216.8147464187570108 ) ) ;
#72946=( BOUNDED_CURVE ( )  B_SPLINE_CURVE ( 3, ( #101901, #49881, #33057, #67245 ),
 .UNSPECIFIED., .F., .F. ) 
 B_SPLINE_CURVE_WITH_KNOTS ( ( 4, 4 ),
 ( 4.712545043314881887, 6.283338161952983114 ),
 .UNSPECIFIED. ) 
 CURVE ( )  GEOMETRIC_REPRESENTATION_ITEM ( )  RATIONAL_B_SPLINE_CURVE ( ( 1.000000000000000000, 0.8047386102935668584, 0.8047386102935668584, 1.000000000000000000 ) ) 
 REPRESENTATION_ITEM ( '' )  );
#72952=CARTESIAN_POINT ( 'NONE',  ( -5.788097265284999793, 1517.099836525840146, 206.6397780718770036 ) ) ;
#72956=VERTEX_POINT ( 'NONE', #2184 ) ;
#72962=CARTESIAN_POINT ( 'NONE',  ( -5.469699274806250067, 1510.954290761809943, 201.4579565197620070 ) ) ;
#72969=CARTESIAN_POINT ( 'NONE',  ( -2.483949978725000118, 1517.156142772249950, 216.0726795003369887 ) ) ;
#72973=CARTESIAN_POINT ( 'NONE',  ( 7.335900995594999863, 1517.068717944079935, 213.1567545299469657 ) ) ;
#72992=CARTESIAN_POINT ( 'NONE',  ( 2.285487581364999965, 1517.001127920769704, 205.0775242521070254 ) ) ;
#73020=CARTESIAN_POINT ( 'NONE',  ( 8.147597079235938011, 1511.509056589849934, 205.2719880346207901 ) ) ;
#73022=B_SPLINE_CURVE_WITH_KNOTS ( 'NONE', 5,
 ( #6355, #5818, #40503, #107159, #13625, #29890 ),
 .UNSPECIFIED., .F., .F.,
 ( 6, 6 ),
 ( 0.000000000000000000, 1.000000000000000000 ),
 .UNSPECIFIED. ) ;
#73025=EDGE_CURVE ( 'NONE', #21931, #48402, #36299, .T. ) ;
#73026=ORIENTED_EDGE ( 'NONE', *, *, #50103, .F. ) ;
#73027=DIRECTION ( 'NONE',  ( 0.000000000000000000, 1.000000000000000000, -6.123233995736769734E-17 ) ) ;
#73028=CARTESIAN_POINT ( 'NONE',  ( -7.509820346537817493, 1510.675349056949244, 215.1027603218261106 ) ) ;
#73031=CARTESIAN_POINT ( 'NONE',  ( -12.85600966886500096, 1512.300546902530186, 193.9285717199670103 ) ) ;
#73034=CARTESIAN_POINT ( 'NONE',  ( -3.454748846324999789, 1516.609912606490070, 201.7988116581369979 ) ) ;
#73060=CARTESIAN_POINT ( 'NONE',  ( 3.415238410854999795, 1511.775527460079957, 212.5370843810869985 ) ) ;
#73071=CARTESIAN_POINT ( 'NONE',  ( -3.451033427095000050, 1517.025653221279981, 214.9083735325669977 ) ) ;
#73080=CARTESIAN_POINT ( 'NONE',  ( -3.460101890015000237, 1516.812923327049930, 205.0932153474469715 ) ) ;
#73093=CARTESIAN_POINT ( 'NONE',  ( -7.710610441124999603, 1516.594591938570147, 212.5759658869370128 ) ) ;
#73098=CARTESIAN_POINT ( 'NONE',  ( -7.709376407373089712, 1516.547466091170008, 210.8176141999059894 ) ) ;
#73099=CARTESIAN_POINT ( 'NONE',  ( -6.935801299664999142, 1516.621991115350056, 210.2518484644969874 ) ) ;
#73103=ORIENTED_EDGE ( 'NONE', *, *, #103453, .T. ) ;
#73108=CARTESIAN_POINT ( 'NONE',  ( 7.548380872364999661, 1510.399296111369949, 204.3167683741870064 ) ) ;
#73111=CARTESIAN_POINT ( 'NONE',  ( 4.036748838804999906, 1516.667393516340098, 216.0582443258770127 ) ) ;
#73116=CARTESIAN_POINT ( 'NONE',  ( 6.553524377605000062, 1516.882690742909972, 202.1776141839370098 ) ) ;
#73122=CARTESIAN_POINT ( 'NONE',  ( 7.558249307053370281, 1510.689985724130111, 203.4323075703590007 ) ) ;
#73133=ORIENTED_EDGE ( 'NONE', *, *, #27478, .F. ) ;
#73143=DIRECTION ( 'NONE',  ( 0.000000000000000000, -6.123233995736759873E-17, -1.000000000000000000 ) ) ;
#73153=CARTESIAN_POINT ( 'NONE',  ( 14.28356506509309831, 1513.356256558030054, 224.3145391780770126 ) ) ;
#73165=AXIS2_PLACEMENT_3D ( 'NONE', #38612, #10680, #62203 ) ;
#73193=CARTESIAN_POINT ( 'NONE',  ( -4.026614517785000125, 1516.699825673279975, 210.8361802174170236 ) ) ;
#73195=CARTESIAN_POINT ( 'NONE',  ( 2.298369469825000344, 1516.779243033999819, 212.3734572960470075 ) ) ;
#73203=CARTESIAN_POINT ( 'NONE',  ( -1.708092304294999808, 1516.523379810429788, 201.4131002843170108 ) ) ;
#73211=ORIENTED_EDGE ( 'NONE', *, *, #103630, .F. ) ;
#73218=CARTESIAN_POINT ( 'NONE',  ( 6.564578685215000320, 1517.199196846569976, 210.8299485595169926 ) ) ;
#73225=CARTESIAN_POINT ( 'NONE',  ( -3.463767296015000330, 1517.014196759610059, 207.4190915607570105 ) ) ;
#73243=CARTESIAN_POINT ( 'NONE',  ( 3.263521904354999670, 1516.676340709600026, 214.8942497445370066 ) ) ;
#73245=CARTESIAN_POINT ( 'NONE',  ( 7.709178328070479758, 1516.539903203899939, 206.5651024190640044 ) ) ;
#73266=CYLINDRICAL_SURFACE ( 'NONE', #99181, 0.9999999999999982236 ) ;
#73268=CARTESIAN_POINT ( 'NONE',  ( -10.96015512746500065, 1514.690994518219895, 193.2119433744669834 ) ) ;
#73270=CARTESIAN_POINT ( 'NONE',  ( -3.558864061465000006, 1511.483345606789953, 201.2317265620570197 ) ) ;
#73279=AXIS2_PLACEMENT_3D ( 'NONE', #22474, #32567, #93006 ) ;
#73290=DIRECTION ( 'NONE',  ( 0.000000000000000000, 6.123233995736769734E-17, 1.000000000000000000 ) ) ;
#73312=CARTESIAN_POINT ( 'NONE',  ( -7.536818064318620003, 1511.326458810320219, 215.2928205442640035 ) ) ;
#73316=CARTESIAN_POINT ( 'NONE',  ( 4.610079833424999940, 1516.713079096360161, 207.9883289669969884 ) ) ;
#73329=CARTESIAN_POINT ( 'NONE',  ( -15.25688968024340042, 1512.464953430870082, 222.2583362424209952 ) ) ;
#73346=CARTESIAN_POINT ( 'NONE',  ( 4.119399112420410347, 1508.879003890470131, 204.7521254745670092 ) ) ;
#73355=CARTESIAN_POINT ( 'NONE',  ( 7.712490952985000980, 1516.666407245520077, 204.5049844236870058 ) ) ;
#73364=CARTESIAN_POINT ( 'NONE',  ( 4.987078422726499483, 1508.551704408389924, 205.6342535031670025 ) ) ;
#73389=ORIENTED_EDGE ( 'NONE', *, *, #8584, .F. ) ;
#73433=B_SPLINE_CURVE_WITH_KNOTS ( 'NONE', 3,
 ( #79083, #11319, #34843, #104263, #61735, #53900, #69034, #95859, #53327, #105371, #62291, #44936, #2390, #88035, #79631, #2935, #71248, #55528, #97515, #39251, #80717, #71811, #11859, #12397, #29210, #37609, #4026, #12940, #105931 ),
 .UNSPECIFIED., .F., .F.,
 ( 4, 2, 2, 1, 1, 2, 2, 2, 2, 2, 2, 2, 1, 2, 2, 4 ),
 ( 0.000000000000000000, 0.1250000000000399958, 0.1875000000000586753, 0.2187500000000699718, 0.2343749999999852340, 0.2421874999998512579, 0.2499999999997172817, 0.3750000000002788880, 0.4375000000005585532, 0.5000000000008382184, 0.6250000000009311441, 0.6875000000011701751, 0.7187500000011074475, 0.7343750000010753620, 0.7500000000010433876, 1.000000000000000000 ),
 .UNSPECIFIED. ) ;
#73458=CARTESIAN_POINT ( 'NONE',  ( -4.613769899311276568, 1511.398921086024302, 200.7270633290623607 ) ) ;
#73465=CARTESIAN_POINT ( 'NONE',  ( -4.042417815834999928, 1516.904492006980036, 205.6736390534169914 ) ) ;
#73470=EDGE_LOOP ( 'NONE', ( #65357, #58883, #29915, #23063 ) ) ;
#73479=CARTESIAN_POINT ( 'NONE',  ( -0.7352271553329990939, 1516.963431999339946, 210.8369554172870153 ) ) ;
#73494=CARTESIAN_POINT ( 'NONE',  ( 16.25286368722670716, 1514.564622118244188, 194.3294294352374436 ) ) ;
#73502=DIRECTION ( 'NONE',  ( 0.02616798426433289068, 0.9993150019884036173, 0.02616798426433289068 ) ) ;
#73508=CARTESIAN_POINT ( 'NONE',  ( 3.487592428934999766, 1509.038615934169911, 204.6345961781970004 ) ) ;
#73509=CARTESIAN_POINT ( 'NONE',  ( 7.710966977635000497, 1516.608208975040043, 207.9930883710269711 ) ) ;
#73517=FACE_OUTER_BOUND ( 'NONE', #77229, .T. ) ;
#73524=CARTESIAN_POINT ( 'NONE',  ( -6.187521092793239141, 1510.844697583444713, 201.6626558324045391 ) ) ;
#73529=CARTESIAN_POINT ( 'NONE',  ( -0.7403206051589980019, 1517.139320148880188, 216.8467205834170102 ) ) ;
#73533=CARTESIAN_POINT ( 'NONE',  ( -3.254401441735000233, 1516.919782530640077, 213.1645757730269963 ) ) ;
#73545=EDGE_CURVE ( 'NONE', #89306, #29708, #9282, .T. ) ;
#73553=CARTESIAN_POINT ( 'NONE',  ( -7.334957394705000411, 1517.030858226499959, 204.5055736355369902 ) ) ;
#73561=DIRECTION ( 'NONE',  ( 0.000000000000000000, -1.000000000000000000, 6.123233995736769734E-17 ) ) ;
#73584=CARTESIAN_POINT ( 'NONE',  ( 8.517158571662550415, 1511.399506464603064, 204.1391972876773480 ) ) ;
#73591=CARTESIAN_POINT ( 'NONE',  ( -7.540791941105130292, 1510.557600718731237, 214.8905100802431036 ) ) ;
#73595=CARTESIAN_POINT ( 'NONE',  ( -13.86270804226499997, 1513.875858217480072, 192.3565727231670053 ) ) ;
#73598=CARTESIAN_POINT ( 'NONE',  ( -0.7533001734329990429, 1516.714320817460020, 201.7957737879569891 ) ) ;
#73601=CARTESIAN_POINT ( 'NONE',  ( 15.31485518243500010, 1513.484013041540038, 194.5539220954669872 ) ) ;
#73606=CARTESIAN_POINT ( 'NONE',  ( 4.987078429774149946, 1508.551704408389924, 205.1632116869930087 ) ) ;
#73614=CARTESIAN_POINT ( 'NONE',  ( -7.588802720235000798, 1511.942942747529969, 211.3806715220270007 ) ) ;
#73633=CARTESIAN_POINT ( 'NONE',  ( -6.940473372275000052, 1516.833525648419936, 215.6778681647369922 ) ) ;
#73641=CARTESIAN_POINT ( 'NONE',  ( 7.710285837685000310, 1516.582197289609894, 205.8614676770269796 ) ) ;
#73643=CARTESIAN_POINT ( 'NONE',  ( -4.037051035714999792, 1516.939819969850078, 209.1350663277499962 ) ) ;
#73656=CARTESIAN_POINT ( 'NONE',  ( 0.01328393942530149870, 1516.939580991450157, 212.3834982571270018 ) ) ;
#73661=CARTESIAN_POINT ( 'NONE',  ( -7.709060745858529629, 1516.535411464270055, 210.9785344462470107 ) ) ;
#73662=CARTESIAN_POINT ( 'NONE',  ( -2.865636847234999784, 1516.815173273089840, 210.2578502442970318 ) ) ;
#73665=CARTESIAN_POINT ( 'NONE',  ( -5.513435705061030312, 1509.038615938849944, 201.6090957135359929 ) ) ;
#73670=AXIS2_PLACEMENT_3D ( 'NONE', #93730, #1365, #69701 ) ;
#73678=DIRECTION ( 'NONE',  ( -1.000000000000000000, 0.000000000000000000, 0.000000000000000000 ) ) ;
#73679=CARTESIAN_POINT ( 'NONE',  ( -2.483949978725000118, 1517.156142772249950, 216.0726795003369887 ) ) ;
#73684=CARTESIAN_POINT ( 'NONE',  ( -2.291047527245000381, 1516.524310051880093, 201.4130759250869858 ) ) ;
#73714=FACE_OUTER_BOUND ( 'NONE', #54233, .T. ) ;
#73722=CARTESIAN_POINT ( 'NONE',  ( 12.45742383169469925, 1512.169469372300000, 224.0727726720780026 ) ) ;
#73726=CARTESIAN_POINT ( 'NONE',  ( 6.238899643214079305, 1516.716532632738563, 204.9585377404597466 ) ) ;
#73760=CARTESIAN_POINT ( 'NONE',  ( -1.118104767724999782, 1516.965971551240045, 211.4215139361070044 ) ) ;
#73763=CARTESIAN_POINT ( 'NONE',  ( 4.623787969365000805, 1516.947419719950176, 212.5709951659769956 ) ) ;
#73770=CARTESIAN_POINT ( 'NONE',  ( 4.615017327834999961, 1516.987478262539980, 202.5620478758069964 ) ) ;
#73780=CARTESIAN_POINT ( 'NONE',  ( 8.133565924525001378, 1515.203649598490074, 214.8418076220970079 ) ) ;
#73784=CARTESIAN_POINT ( 'NONE',  ( -5.772978316675000166, 1516.659138130710289, 210.2536427808470023 ) ) ;
#73790=CARTESIAN_POINT ( 'NONE',  ( 4.997718238375000510, 1516.693851263360102, 207.9888968556769839 ) ) ;
#73808=CARTESIAN_POINT ( 'NONE',  ( 1.129386202275000084, 1516.613712827999962, 216.4452363774470030 ) ) ;
#73810=CARTESIAN_POINT ( 'NONE',  ( 7.709283117220651071, 1516.543904940109996, 207.3844237024999870 ) ) ;
#73859=CARTESIAN_POINT ( 'NONE',  ( 15.95461386393500369, 1514.857962383129916, 193.9637614619669819 ) ) ;
#73862=ORIENTED_EDGE ( 'NONE', *, *, #56227, .F. ) ;
#73870=CARTESIAN_POINT ( 'NONE',  ( -7.708815826551380646, 1516.526058373149908, 211.4663580544020078 ) ) ;
#73875=CARTESIAN_POINT ( 'NONE',  ( -6.563915562015000482, 1517.184063036290127, 207.9975562766469750 ) ) ;
#73904=CARTESIAN_POINT ( 'NONE',  ( 4.556910988561660325, 1508.729442836390035, 205.2988677068620120 ) ) ;
#73911=CARTESIAN_POINT ( 'NONE',  ( -7.334957394705000411, 1517.030858226499959, 204.5055736355369902 ) ) ;
#73914=CARTESIAN_POINT ( 'NONE',  ( 14.72576938353500076, 1512.123542805230272, 196.9321265835669976 ) ) ;
#73994=FACE_OUTER_BOUND ( 'NONE', #40363, .T. ) ;
#74002=CARTESIAN_POINT ( 'NONE',  ( -4.551369695278060235, 1511.401872466681198, 200.7475796568508599 ) ) ;
#74010=CARTESIAN_POINT ( 'NONE',  ( -5.786527600464999033, 1517.025653221279981, 205.6708125431369751 ) ) ;
#74024=EDGE_CURVE ( 'NONE', #37961, #29868, #84449, .T. ) ;
#74025=CARTESIAN_POINT ( 'NONE',  ( 6.951517132375000685, 1517.194816588360027, 210.2467400204669730 ) ) ;
#74054=CARTESIAN_POINT ( 'NONE',  ( 4.615644804385000022, 1517.009964551830080, 202.1744681489270192 ) ) ;
#74055=CARTESIAN_POINT ( 'NONE',  ( 3.447128460625000113, 1516.778853242349896, 207.9866608880570027 ) ) ;
#74058=B_SPLINE_CURVE_WITH_KNOTS ( 'NONE', 3,
 ( #6461, #15931, #74239, #23791, #74780, #24346, #84261, #50134, #82622, #92114 ),
 .UNSPECIFIED., .F., .F.,
 ( 4, 2, 2, 2, 4 ),
 ( 0.000000000000000000, 0.2500000000000000000, 0.5000000000000000000, 0.7500000000000000000, 1.000000000000000000 ),
 .UNSPECIFIED. ) ;
#74071=PLANE ( 'NONE',  #85725 ) ;
#74076=CARTESIAN_POINT ( 'NONE',  ( 7.329925222404999552, 1516.833976295079992, 216.8387248732070134 ) ) ;
#74082=CARTESIAN_POINT ( 'NONE',  ( -7.322709724964999722, 1516.596789218710001, 212.3828531017969965 ) ) ;
#74100=CARTESIAN_POINT ( 'NONE',  ( -5.011678876155000850, 1516.989560013210166, 205.8658785457569991 ) ) ;
#74131=CARTESIAN_POINT ( 'NONE',  ( 8.374229031442469662, 1511.401878032981131, 204.5705829445117274 ) ) ;
#74145=EDGE_CURVE ( 'NONE', #90411, #97290, #66441, .T. ) ;
#74147=CARTESIAN_POINT ( 'NONE',  ( -7.331183129075000693, 1516.882217593000178, 202.1801186797769674 ) ) ;
#74150=CARTESIAN_POINT ( 'NONE',  ( 16.20447078603499946, 1512.376261820769969, 197.7654888015669883 ) ) ;
#74160=EDGE_LOOP ( 'NONE', ( #41335, #60432, #55341, #50192 ) ) ;
#74164=CARTESIAN_POINT ( 'NONE',  ( -7.774021443175000101, 1512.205735116489905, 211.9443100603170080 ) ) ;
#74171=CARTESIAN_POINT ( 'NONE',  ( 7.722580314274999580, 1517.051704408389924, 209.1218459511669892 ) ) ;
#74184=CARTESIAN_POINT ( 'NONE',  ( 7.718134629434999283, 1516.881930554049859, 216.4517759834270123 ) ) ;
#74193=CARTESIAN_POINT ( 'NONE',  ( -2.492130661305000050, 1516.778761582560037, 205.6761608547170113 ) ) ;
#74195=CARTESIAN_POINT ( 'NONE',  ( -7.337297350114999617, 1517.135701590510052, 208.3821536943570152 ) ) ;
#74198=CARTESIAN_POINT ( 'NONE',  ( 6.462730625455000322, 1512.074228085019968, 217.6482617061570011 ) ) ;
#74204=AXIS2_PLACEMENT_3D ( 'NONE', #54786, #13842, #48590 ) ;
#74211=CARTESIAN_POINT ( 'NONE',  ( -3.254401441735000233, 1516.919782530640077, 213.1645757730269963 ) ) ;
#74216=CARTESIAN_POINT ( 'NONE',  ( -7.709125739314820258, 1516.537893464249919, 211.6437737813369893 ) ) ;
#74217=CARTESIAN_POINT ( 'NONE',  ( 5.013429356055000063, 1517.123342927159911, 210.2437967141769946 ) ) ;
#74231=CARTESIAN_POINT ( 'NONE',  ( -4.616272334694999202, 1517.030858226499959, 216.4568033268070053 ) ) ;
#74236=CARTESIAN_POINT ( 'NONE',  ( -0.01073133209419849937, 1516.939491476980038, 201.7897819926569980 ) ) ;
#74237=CARTESIAN_POINT ( 'NONE',  ( -15.26322412056499900, 1511.857118786289902, 221.3099577525670156 ) ) ;
#74238=ORIENTED_EDGE ( 'NONE', *, *, #70755, .T. ) ;
#74239=CARTESIAN_POINT ( 'NONE',  ( 6.036759309035796939, 1509.035273820309612, 216.5824821311529433 ) ) ;
#74240=AXIS2_PLACEMENT_3D ( 'NONE', #77756, #78299, #1612 ) ;
#74270=VERTEX_POINT ( 'NONE', #42190 ) ;
#74273=CARTESIAN_POINT ( 'NONE',  ( 12.82673415024670049, 1512.305164330090065, 224.2762155789449992 ) ) ;
#74311=ORIENTED_EDGE ( 'NONE', *, *, #98337, .F. ) ;
#74313=CARTESIAN_POINT ( 'NONE',  ( 6.562635822504999439, 1517.111322026010157, 211.9927976380170094 ) ) ;
#74317=CARTESIAN_POINT ( 'NONE',  ( -3.253141175365000137, 1516.858171774179937, 212.3894494859370070 ) ) ;
#74325=CARTESIAN_POINT ( 'NONE',  ( -2.292307268505000106, 1516.548716157039962, 202.1882291110970300 ) ) ;
#74341=CARTESIAN_POINT ( 'NONE',  ( -4.608146819384999482, 1516.677239312369920, 211.4179708211670174 ) ) ;
#74346=CARTESIAN_POINT ( 'NONE',  ( 7.564413961465000114, 1511.011611623900080, 205.8421879128569856 ) ) ;
#74347=CARTESIAN_POINT ( 'NONE',  ( -2.881548462575000080, 1516.909589401870107, 206.8382752989369919 ) ) ;
#74365=CARTESIAN_POINT ( 'NONE',  ( -2.290886304614999869, 1517.184383877180153, 216.4605998004670084 ) ) ;
#74405=ORIENTED_EDGE ( 'NONE', *, *, #66692, .F. ) ;
#74423=B_SPLINE_CURVE_WITH_KNOTS ( 'NONE', 3,
 ( #20933, #69738, #103856, #70297, #61889, #65726, #32109, #14191, #89806, #100411, #4700, #30999, #99289, #23139, #89259, #64635, #47264, #66295, #21474, #12554, #56770, #14748, #90907, #83064, #73020, #22016, #80866, #99846, #38295, #22565, #46732, #55684, #13077, #74131, #47813, #4165, #90344, #72475, #55139, #81948, #30451, #57343, #31548, #98756, #73584, #48378, #91467, #81386, #48935 ),
 .UNSPECIFIED., .F., .F.,
 ( 4, 2, 1, 2, 2, 2, 1, 1, 2, 2, 2, 2, 1, 1, 1, 2, 2, 2, 2, 1, 1, 1, 2, 2, 2, 1, 1, 2, 2, 4 ),
 ( 0.000000000000000000, 0.06250000000038768988, 0.09375000000058156258, 0.1093750000005562634, 0.1250000000005309642, 0.1875000000006294132, 0.2187500000006786516, 0.2343750000007824574, 0.2421875000008341661, 0.2500000000008858470, 0.3750000000014287460, 0.4375000000016672219, 0.4687500000017752466, 0.4843750000018290369, 0.4921875000018212098, 0.4960937500018174906, 0.5000000000018137714, 0.6250000000016393553, 0.6875000000015790702, 0.7187500000015458745, 0.7343750000015293322, 0.7421875000015359936, 0.7460937500015292212, 0.7500000000015223378, 0.8125000000012090329, 0.8437500000010399459, 0.8593750000009554579, 0.8671875000009101608, 0.8750000000008649748, 1.000000000000000000 ),
 .UNSPECIFIED. ) ;
#74437=CARTESIAN_POINT ( 'NONE',  ( 2.863787855735000054, 1516.788317650260069, 207.4054531903269947 ) ) ;
#74461=ORIENTED_EDGE ( 'NONE', *, *, #74024, .F. ) ;
#74465=CARTESIAN_POINT ( 'NONE',  ( 4.333389510011039114, 1508.551704407329908, 204.4537291618960069 ) ) ;
#74472=CARTESIAN_POINT ( 'NONE',  ( -3.861651061951890007, 1508.610718263850003, 204.4420517364369800 ) ) ;
#74474=CARTESIAN_POINT ( 'NONE',  ( 1.120543697654999837, 1517.073005577650065, 205.0775260448770041 ) ) ;
#74483=CARTESIAN_POINT ( 'NONE',  ( -13.40617548155469940, 1512.633419863009976, 193.8191794496820251 ) ) ;
#74494=CARTESIAN_POINT ( 'NONE',  ( -7.668984248404999704, 1514.216129015420165, 202.9976746052270187 ) ) ;
#74558=CARTESIAN_POINT ( 'NONE',  ( -3.215705694400522674, 1511.798535855272576, 201.1683149189278197 ) ) ;
#74563=CARTESIAN_POINT ( 'NONE',  ( -3.266349512195000138, 1516.797038924770050, 205.0935381919470046 ) ) ;
#74577=CARTESIAN_POINT ( 'NONE',  ( 0.01012488564660149991, 1516.989863902050047, 210.2497743036369968 ) ) ;
#74606=CARTESIAN_POINT ( 'NONE',  ( 6.554151426245000245, 1516.906641539930206, 201.7900338461269882 ) ) ;
#74607=CARTESIAN_POINT ( 'NONE',  ( 1.119592181715000079, 1516.958737650239982, 207.9859471464170326 ) ) ;
#74608=VERTEX_POINT ( 'NONE', #102901 ) ;
#74613=CARTESIAN_POINT ( 'NONE',  ( -8.612924558394999153, 1512.851027864960088, 211.3708094598169964 ) ) ;
#74617=CARTESIAN_POINT ( 'NONE',  ( -5.495614756258980549, 1510.802068165409992, 201.5298705880650232 ) ) ;
#74625=CARTESIAN_POINT ( 'NONE',  ( -6.554151464375000735, 1516.906641539930206, 216.4536580562070185 ) ) ;
#74629=CARTESIAN_POINT ( 'NONE',  ( 0.4614184642274221093, 1516.800601748523150, 216.8378509299481038 ) ) ;
#74630=CARTESIAN_POINT ( 'NONE',  ( 0.01327404799950150129, 1516.939877939420057, 212.5773418040870126 ) ) ;
#74633=CARTESIAN_POINT ( 'NONE',  ( 4.679794176543860651, 1508.610718243669908, 212.9835092646939927 ) ) ;
#74648=ORIENTED_EDGE ( 'NONE', *, *, #21983, .F. ) ;
#74649=CARTESIAN_POINT ( 'NONE',  ( -7.337153806245000354, 1517.119374999550018, 205.8621166342670108 ) ) ;
#74696=CARTESIAN_POINT ( 'NONE',  ( 3.452289182574999948, 1517.069378699710114, 202.5601595088670024 ) ) ;
#74700=CARTESIAN_POINT ( 'NONE',  ( 14.97406870653500022, 1513.863307887919973, 194.3519930166669951 ) ) ;
#74731=CARTESIAN_POINT ( 'NONE',  ( -3.452289220704999551, 1517.069378699710114, 215.6835323934670328 ) ) ;
#74737=CARTESIAN_POINT ( 'NONE',  ( 7.322709686834999232, 1516.596789218710001, 205.8608388005369818 ) ) ;
#74739=CARTESIAN_POINT ( 'NONE',  ( 6.944466742375000834, 1516.939530130779985, 209.1105810159089913 ) ) ;
#74742=CARTESIAN_POINT ( 'NONE',  ( 6.564976393265000709, 1512.035910181050212, 216.6257190735869926 ) ) ;
#74752=CARTESIAN_POINT ( 'NONE',  ( -2.286446363765000100, 1517.042661899400173, 213.7475398352470108 ) ) ;
#74757=CARTESIAN_POINT ( 'NONE',  ( -7.715720925248570339, 1516.789754148820066, 209.6216723975360026 ) ) ;
#74758=CARTESIAN_POINT ( 'NONE',  ( -5.772978316675000166, 1516.659138130710289, 210.2536427808470023 ) ) ;
#74772=CARTESIAN_POINT ( 'NONE',  ( -2.291514335905000088, 1517.194972660189933, 216.8481778957070105 ) ) ;
#74776=VECTOR ( 'NONE', #80041, 1000.000000000000114 ) ;
#74778=CARTESIAN_POINT ( 'NONE',  ( 7.326795523374999952, 1516.760434454289907, 203.3416138547669902 ) ) ;
#74779=CARTESIAN_POINT ( 'NONE',  ( -15.36767547136500056, 1514.414736986979960, 224.4986524488670057 ) ) ;
#74780=CARTESIAN_POINT ( 'NONE',  ( 6.742044461270444877, 1509.032357807656808, 216.2339689528981239 ) ) ;
#74800=CARTESIAN_POINT ( 'NONE',  ( -4.678149183724549687, 1508.611352722540005, 212.6094318194529933 ) ) ;
#74844=B_SPLINE_CURVE_WITH_KNOTS ( 'NONE', 3,
 ( #109017, #15473, #41794, #926, #43469, #35049 ),
 .UNSPECIFIED., .F., .F.,
 ( 4, 2, 4 ),
 ( 1.353581492229530087E-06, 0.01184126496313610104, 0.02355708206288909673 ),
 .UNSPECIFIED. ) ;
#74857=CARTESIAN_POINT ( 'NONE',  ( 1.716392741775000008, 1516.788317650260069, 211.9856338259669997 ) ) ;
#74861=CARTESIAN_POINT ( 'NONE',  ( -4.609996619675000851, 1516.769879638719885, 212.5810025483170023 ) ) ;
#74867=CARTESIAN_POINT ( 'NONE',  ( -2.874588960795000148, 1516.606339319019980, 202.5748942495170013 ) ) ;
#74883=CARTESIAN_POINT ( 'NONE',  ( -3.251611363945000388, 1516.779243033999819, 211.4202154400570066 ) ) ;
#74888=CARTESIAN_POINT ( 'NONE',  ( 2.864043418315000089, 1516.811292230880099, 206.8228319013669818 ) ) ;
#74909=CARTESIAN_POINT ( 'NONE',  ( -6.941100315875000426, 1516.858069504249897, 216.0654486236869900 ) ) ;
#74926=DIRECTION ( 'NONE',  ( 0.4999999999998399058, 0.7071067811867739472, 0.4999999999998399058 ) ) ;
#74928=ORIENTED_EDGE ( 'NONE', *, *, #92600, .T. ) ;
#74943=CARTESIAN_POINT ( 'NONE',  ( -5.181410188784999704, 1510.418062979269962, 201.5729736320070060 ) ) ;
#74977=CARTESIAN_POINT ( 'NONE',  ( -7.722580352405000070, 1517.051704408389924, 207.5526846776770071 ) ) ;
#74986=CARTESIAN_POINT ( 'NONE',  ( 3.261652286895000419, 1516.939580991450157, 209.1085619926769823 ) ) ;
#74990=VECTOR ( 'NONE', #35345, 1000.000000000000114 ) ;
#74995=CARTESIAN_POINT ( 'NONE',  ( -15.02944349056170026, 1512.205851781539877, 221.7001744404510077 ) ) ;
#75006=ORIENTED_EDGE ( 'NONE', *, *, #85135, .T. ) ;
#75017=CARTESIAN_POINT ( 'NONE',  ( -4.833437595822498878, 1508.551704408439946, 205.2116919714409846 ) ) ;
#75019=CARTESIAN_POINT ( 'NONE',  ( 4.997573787194999895, 1516.742629295279812, 205.6633194342169872 ) ) ;
#75022=CARTESIAN_POINT ( 'NONE',  ( 15.03014119857349939, 1513.722010160979835, 194.4919335047299853 ) ) ;
#75026=VECTOR ( 'NONE', #65334, 1000.000000000000114 ) ;
#75028=CARTESIAN_POINT ( 'NONE',  ( -14.28356510322089790, 1513.356256558030054, 193.9291527242570226 ) ) ;
#75038=B_SPLINE_CURVE_WITH_KNOTS ( 'NONE', 5,
 ( #96791, #19506, #53711, #45297, #69399, #61546, #34660, #52587, #95677 ),
 .UNSPECIFIED., .F., .F.,
 ( 6, 3, 6 ),
 ( 0.8631819232519999385, 2.053866005980000242, 3.194084093449060191 ),
 .UNSPECIFIED. ) ;
#75067=LINE ( 'NONE', #91841, #12744 ) ;
#75097=ORIENTED_EDGE ( 'NONE', *, *, #108527, .T. ) ;
#75112=CARTESIAN_POINT ( 'NONE',  ( -2.968355423891683387, 1512.111483631942974, 201.2327182046635983 ) ) ;
#75117=CARTESIAN_POINT ( 'NONE',  ( 7.322105067625000352, 1516.572193931679976, 206.2485165713470110 ) ) ;
#75126=CARTESIAN_POINT ( 'NONE',  ( -16.25736646461311707, 1514.559393050436938, 223.9077632415501000 ) ) ;
#75130=CARTESIAN_POINT ( 'NONE',  ( 1.136814033864999907, 1516.854133554269993, 211.4058994415870245 ) ) ;
#75150=CARTESIAN_POINT ( 'NONE',  ( -2.000000019065000245, 1517.051704408389924, 222.4523892994670007 ) ) ;
#75154=CARTESIAN_POINT ( 'NONE',  ( 6.541070334811199594, 1517.051704644130041, 212.7912326336579838 ) ) ;
#75159=CARTESIAN_POINT ( 'NONE',  ( -2.485217232065000115, 1516.534320418310244, 201.4128137944169907 ) ) ;
#75160=CARTESIAN_POINT ( 'NONE',  ( 6.548200587644999793, 1516.632821972880038, 207.9912384682270101 ) ) ;
#75182=CARTESIAN_POINT ( 'NONE',  ( 0.5608844116969206040, 1516.772451887518400, 216.8371137998956613 ) ) ;
#75183=CARTESIAN_POINT ( 'NONE',  ( -7.324914956285000223, 1516.685667699390024, 213.7393364370070117 ) ) ;
#75201=CARTESIAN_POINT ( 'NONE',  ( -7.724732447025000504, 1517.133889586189980, 205.8614888033369823 ) ) ;
#75223=CARTESIAN_POINT ( 'NONE',  ( -14.72258237740398101, 1514.508948671113103, 192.8217237370948851 ) ) ;
#75232=( BOUNDED_CURVE ( )  B_SPLINE_CURVE ( 3, ( #38567, #72213, #55399, #13905 ),
 .UNSPECIFIED., .F., .F. ) 
 B_SPLINE_CURVE_WITH_KNOTS ( ( 4, 4 ),
 ( 2.354951096460577986, 3.925058729076146058 ),
 .UNSPECIFIED. ) 
 CURVE ( )  GEOMETRIC_REPRESENTATION_ITEM ( )  RATIONAL_B_SPLINE_CURVE ( ( 1.000000000000000000, 0.8049001529475701133, 0.8049001529475701133, 1.000000000000000000 ) ) 
 REPRESENTATION_ITEM ( '' )  );
#75238=CARTESIAN_POINT ( 'NONE',  ( -5.371346839175000554, 1520.551704408390151, 218.7599618298069970 ) ) ;
#75240=CARTESIAN_POINT ( 'NONE',  ( -7.519244436443294433, 1510.642476678762705, 215.0516229487886335 ) ) ;
#75246=CARTESIAN_POINT ( 'NONE',  ( -6.541070373676360461, 1517.051704644259871, 205.4524592699869743 ) ) ;
#75250=CARTESIAN_POINT ( 'NONE',  ( 4.612507273904999039, 1516.886345593249871, 204.1123678647870179 ) ) ;
#75253=CARTESIAN_POINT ( 'NONE',  ( 16.57141199633499795, 1514.216506490359961, 194.7449369304669915 ) ) ;
#75283=CARTESIAN_POINT ( 'NONE',  ( 3.669386717837979983, 1517.051704638620095, 202.5807756278150009 ) ) ;
#75286=CARTESIAN_POINT ( 'NONE',  ( -2.870951705914999597, 1517.111322026010157, 215.6844817927369888 ) ) ;
#75287=CARTESIAN_POINT ( 'NONE',  ( -7.953531051250857686, 1511.798535855328510, 212.3375516263953386 ) ) ;
#75294=CARTESIAN_POINT ( 'NONE',  ( -4.624099329465000352, 1516.962555622980062, 205.8665050058069994 ) ) ;
#75296=CARTESIAN_POINT ( 'NONE',  ( -1.709766532154999963, 1516.959716008189844, 209.1345041580460133 ) ) ;
#75301=CARTESIAN_POINT ( 'NONE',  ( 6.160280177405000224, 1511.773927532309926, 217.7619188583669825 ) ) ;
#75310=CARTESIAN_POINT ( 'NONE',  ( -6.937338783705000012, 1516.706638732659940, 213.7399656364970042 ) ) ;
#75314=CARTESIAN_POINT ( 'NONE',  ( 7.507423012266849938, 1508.880864730590019, 215.2619739013699984 ) ) ;
#75315=CARTESIAN_POINT ( 'NONE',  ( 2.881325373965000214, 1517.003078582959688, 210.2407492406470055 ) ) ;
#75331=CARTESIAN_POINT ( 'NONE',  ( 2.291047489114999891, 1516.524310051880093, 216.8306159772470210 ) ) ;
#75336=CARTESIAN_POINT ( 'NONE',  ( 5.002593359325000044, 1516.960844870249957, 202.5626772953570196 ) ) ;
#75337=CARTESIAN_POINT ( 'NONE',  ( -15.64724543236500232, 1513.113451381389950, 223.4053766886669905 ) ) ;
#75382=LINE ( 'NONE', #13228, #85780 ) ;
#75411=CARTESIAN_POINT ( 'NONE',  ( 7.338411959395000572, 1517.170512887980067, 211.6064236274570192 ) ) ;
#75416=CARTESIAN_POINT ( 'NONE',  ( 2.879642153204999833, 1516.812046502680005, 212.5681757458869754 ) ) ;
#75424=CARTESIAN_POINT ( 'NONE',  ( 3.258474578945000033, 1517.083030555940013, 202.5598499717069956 ) ) ;
#75439=CARTESIAN_POINT ( 'NONE',  ( -2.282301616165000269, 1516.836638729160086, 210.8392784184970026 ) ) ;
#75445=CARTESIAN_POINT ( 'NONE',  ( 2.863787855735000054, 1516.788317650260069, 207.4054531903269947 ) ) ;
#75463=CARTESIAN_POINT ( 'NONE',  ( 5.784008635194999748, 1516.911981270829983, 214.1231845985469988 ) ) ;
#75465=DIRECTION ( 'NONE',  ( 0.000000000000000000, -1.000000000000000000, 2.084285079594309782E-16 ) ) ;
#75466=CARTESIAN_POINT ( 'NONE',  ( 5.780232077335000440, 1516.760434454289907, 216.4486414936069991 ) ) ;
#75482=LINE ( 'NONE', #7695, #42594 ) ;
#75493=DIRECTION ( 'NONE',  ( 0.000000000000000000, -1.000000000000000000, 6.123233995736769734E-17 ) ) ;
#75497=CARTESIAN_POINT ( 'NONE',  ( -15.20279581456499862, 1513.492015765619954, 193.2119433744669834 ) ) ;
#75502=AXIS2_PLACEMENT_3D ( 'NONE', #78487, #27523, #61708 ) ;
#75508=DIRECTION ( 'NONE',  ( -1.577721810442025012E-32, -1.000000000000000000, 6.123233995736769734E-17 ) ) ;
#75513=EDGE_CURVE ( 'NONE', #89621, #9383, #13681, .T. ) ;
#75533=CARTESIAN_POINT ( 'NONE',  ( -7.596320609278680358, 1510.929912129050081, 214.9254183270510055 ) ) ;
#75539=CARTESIAN_POINT ( 'NONE',  ( 2.868112131164999745, 1516.855632454399938, 208.3641823986619954 ) ) ;
#75576=CARTESIAN_POINT ( 'NONE',  ( 6.936398355645000180, 1516.667393516340098, 205.0850970932970085 ) ) ;
#75662=CARTESIAN_POINT ( 'NONE',  ( -5.012317106364999830, 1517.020727862619879, 206.2534121335969814 ) ) ;
#75675=CARTESIAN_POINT ( 'NONE',  ( 5.013274961385000061, 1517.068517094990057, 211.4089302402969963 ) ) ;
#75702=CARTESIAN_POINT ( 'NONE',  ( -3.261007169695000041, 1516.596789218710001, 201.7991362452670216 ) ) ;
#75703=CARTESIAN_POINT ( 'NONE',  ( -3.261652325025000021, 1516.939580991450157, 209.1351299096569960 ) ) ;
#75706=CARTESIAN_POINT ( 'NONE',  ( 2.937948913181351873, 1512.266332053888846, 217.0095423517265090 ) ) ;
#75723=CARTESIAN_POINT ( 'NONE',  ( -4.616272334694999202, 1517.030858226499959, 216.4568033268070053 ) ) ;
#75727=CARTESIAN_POINT ( 'NONE',  ( 4.621267883935000320, 1516.830644417779922, 214.1213023606370029 ) ) ;
#75745=CARTESIAN_POINT ( 'NONE',  ( -3.267291643295000103, 1516.842852731759876, 205.6749038603869906 ) ) ;
#75776=CARTESIAN_POINT ( 'NONE',  ( 5.649719750514999639, 1514.243099272629934, 201.4728115316369781 ) ) ;
#75781=CARTESIAN_POINT ( 'NONE',  ( -14.76985295356500139, 1513.863307887919973, 194.1477772255670118 ) ) ;
#75788=CARTESIAN_POINT ( 'NONE',  ( -4.037378294184999383, 1516.688761843659904, 202.5730239910470232 ) ) ;
#75791=CARTESIAN_POINT ( 'NONE',  ( 16.89844952793499999, 1513.192861445620110, 196.0568336347670026 ) ) ;
#75816=CARTESIAN_POINT ( 'NONE',  ( 8.664447096804998694, 1512.053281741910041, 202.5614213353869957 ) ) ;
#75825=CARTESIAN_POINT ( 'NONE',  ( -7.716878941104999612, 1516.833976295079992, 216.4517711926369827 ) ) ;
#75826=CARTESIAN_POINT ( 'NONE',  ( -7.894477417095063565, 1512.053565093132875, 212.1161737988796858 ) ) ;
#75832=EDGE_CURVE ( 'NONE', #5115, #89576, #58096, .T. ) ;
#75834=CARTESIAN_POINT ( 'NONE',  ( -4.623788007495000407, 1516.947419719950176, 205.6726967363569827 ) ) ;
#75840=CARTESIAN_POINT ( 'NONE',  ( 7.719525595194999923, 1513.939092156100060, 216.2221105575569879 ) ) ;
#75847=CARTESIAN_POINT ( 'NONE',  ( 2.877113070465000089, 1516.697242742309982, 214.1184881303969973 ) ) ;
#75850=CARTESIAN_POINT ( 'NONE',  ( 6.120119194504639815, 1508.729257029040127, 216.5649251008960050 ) ) ;
#75851=CARTESIAN_POINT ( 'NONE',  ( 6.563595869685000750, 1517.154223579619838, 211.4114704024570131 ) ) ;
#75865=CARTESIAN_POINT ( 'NONE',  ( -7.717505791104999346, 1516.857914730730045, 216.8393517232070167 ) ) ;
#75870=CARTESIAN_POINT ( 'NONE',  ( -3.455378015385000001, 1516.627618683580067, 202.1863880069169852 ) ) ;
#75875=CARTESIAN_POINT ( 'NONE',  ( 1.999999980934999977, 1517.051704408389924, 195.7913026028670060 ) ) ;
#75890=CARTESIAN_POINT ( 'NONE',  ( -4.556911026691660815, 1508.729442836390035, 212.9448241954719947 ) ) ;
#75907=CARTESIAN_POINT ( 'NONE',  ( 4.623921183531392920, 1516.955031447278543, 203.1162470316040185 ) ) ;
#75924=CARTESIAN_POINT ( 'NONE',  ( 7.535878249002015750, 1510.580107397280244, 203.3037915669708013 ) ) ;
#75940=ORIENTED_EDGE ( 'NONE', *, *, #65076, .T. ) ;
#75945=CARTESIAN_POINT ( 'NONE',  ( -1.119717754394999876, 1517.038650117239968, 212.5846815975970117 ) ) ;
#75952=CARTESIAN_POINT ( 'NONE',  ( -7.719392420504999741, 1516.929962200689943, 202.5670673984569703 ) ) ;
#75967=CARTESIAN_POINT ( 'NONE',  ( -6.933616859135000254, 1516.548716157039962, 211.4141532006069895 ) ) ;
#75972=CARTESIAN_POINT ( 'NONE',  ( -5.786847777804999815, 1517.104497701820037, 208.3841784293060186 ) ) ;
#75988=CARTESIAN_POINT ( 'NONE',  ( -3.449149233875000053, 1516.947419719950176, 213.7456339395970133 ) ) ;
#75991=CARTESIAN_POINT ( 'NONE',  ( 7.330554133425000174, 1516.857992118400034, 216.4511490482170188 ) ) ;
#76010=ORIENTED_EDGE ( 'NONE', *, *, #27478, .T. ) ;
#76070=VECTOR ( 'NONE', #93164, 1000.000000000000000 ) ;
#76077=CARTESIAN_POINT ( 'NONE',  ( 2.480427254505000345, 1516.872851364150165, 208.3639601402670110 ) ) ;
#76096=CARTESIAN_POINT ( 'NONE',  ( -7.260305637304787396, 1509.032998980356524, 215.6421396095613545 ) ) ;
#76107=CARTESIAN_POINT ( 'NONE',  ( -4.534001460666400085, 1508.610336687640029, 204.8848403547060002 ) ) ;
#76109=CARTESIAN_POINT ( 'NONE',  ( -1.714334285315000095, 1516.699825673279975, 205.0952314524469955 ) ) ;
#76112=CARTESIAN_POINT ( 'NONE',  ( 15.29028524431559966, 1512.571279492550048, 195.8110339931610042 ) ) ;
#76128=ORIENTED_EDGE ( 'NONE', *, *, #100780, .T. ) ;
#76138=EDGE_CURVE ( 'NONE', #48402, #51877, #60768, .T. ) ;
#76155=CARTESIAN_POINT ( 'NONE',  ( 1.134357970594999987, 1516.744381837270112, 213.1504571913470159 ) ) ;
#76193=CARTESIAN_POINT ( 'NONE',  ( 3.034964868304999897, 1517.051704408389924, 200.9398869892670234 ) ) ;
#76201=CARTESIAN_POINT ( 'NONE',  ( -5.011678876155000850, 1516.989560013210166, 205.8658785457569991 ) ) ;
#76211=CARTESIAN_POINT ( 'NONE',  ( -16.57651866747404057, 1513.029502680755968, 221.0948183014304789 ) ) ;
#76215=CARTESIAN_POINT ( 'NONE',  ( -2.282622950494999969, 1516.861367446839949, 211.4218295478370067 ) ) ;
#76238=CARTESIAN_POINT ( 'NONE',  ( -0.4403324739431219714, 1517.051704035390003, 216.6089087266339845 ) ) ;
#76243=CARTESIAN_POINT ( 'NONE',  ( 1.709384572955000126, 1517.224900789629828, 201.7820965968870155 ) ) ;
#76244=CARTESIAN_POINT ( 'NONE',  ( 1.709766494024999917, 1516.959716008189844, 209.1091877442879934 ) ) ;
#76247=CARTESIAN_POINT ( 'NONE',  ( 3.385873918483515155, 1511.683950138257387, 217.1255238520139415 ) ) ;
#76268=CARTESIAN_POINT ( 'NONE',  ( 1.712644716155000024, 1516.636036526019780, 214.1174694231270053 ) ) ;
#76271=CARTESIAN_POINT ( 'NONE',  ( 4.556911006048280477, 1508.729442775010057, 212.9448352109289999 ) ) ;
#76287=CARTESIAN_POINT ( 'NONE',  ( -5.786527600464999033, 1517.025653221279981, 205.6708125431369751 ) ) ;
#76310=CARTESIAN_POINT ( 'NONE',  ( -14.78979538456069243, 1514.562512395940075, 192.8671644546608661 ) ) ;
#76332=CARTESIAN_POINT ( 'NONE',  ( -7.592573335200579976, 1517.051705360449887, 204.6351128173299969 ) ) ;
#76335=CARTESIAN_POINT ( 'NONE',  ( 6.939219482805000005, 1516.783701990830195, 203.3409846960470020 ) ) ;
#76338=CARTESIAN_POINT ( 'NONE',  ( 15.73511540573499801, 1514.703592237370003, 193.7861023190669982 ) ) ;
#76363=CARTESIAN_POINT ( 'NONE',  ( 7.922128340844998284, 1512.637906871309724, 202.2771797188770222 ) ) ;
#76367=VERTEX_POINT ( 'NONE', #81024 ) ;
#76372=CARTESIAN_POINT ( 'NONE',  ( -1.126138146715000010, 1517.208444099459939, 216.8485306577670144 ) ) ;
#76373=CARTESIAN_POINT ( 'NONE',  ( -7.889127765447542906, 1512.111483631436613, 212.0902013560271655 ) ) ;
#76378=CARTESIAN_POINT ( 'NONE',  ( -4.624736897314999595, 1516.994127245590107, 206.2540423059970180 ) ) ;
#76383=CARTESIAN_POINT ( 'NONE',  ( 7.636446028244999518, 1514.050458741990042, 215.1082210740069911 ) ) ;
#76391=CARTESIAN_POINT ( 'NONE',  ( -4.610938249504999753, 1516.815231249920089, 213.1623732742069990 ) ) ;
#76394=CARTESIAN_POINT ( 'NONE',  ( 7.512716704728560124, 1509.034509440879901, 215.2632436668019977 ) ) ;
#76395=CARTESIAN_POINT ( 'NONE',  ( -2.282622950494999969, 1516.861367446839949, 211.4218295478370067 ) ) ;
#76414=CARTESIAN_POINT ( 'NONE',  ( 2.870951667784999994, 1517.111322026010157, 202.5592101095969895 ) ) ;
#76434=CARTESIAN_POINT ( 'NONE',  ( -4.492644285160710460, 1508.880967439349888, 212.9248381652639921 ) ) ;
#76491=ORIENTED_EDGE ( 'NONE', *, *, #63978, .F. ) ;
#76494=CARTESIAN_POINT ( 'NONE',  ( 6.946748518954999341, 1516.983995446890049, 214.1250666973070054 ) ) ;
#76495=CARTESIAN_POINT ( 'NONE',  ( 5.121512540634999944, 1511.279956263560052, 217.0557608965669658 ) ) ;
#76501=CARTESIAN_POINT ( 'NONE',  ( 7.325541787135000149, 1516.710692850270107, 204.1167749238070144 ) ) ;
#76506=CARTESIAN_POINT ( 'NONE',  ( -10.96015512746500065, 1512.830284628050094, 193.2119433744669834 ) ) ;
#76514=CARTESIAN_POINT ( 'NONE',  ( -4.995623491025000362, 1516.636036526019780, 210.8344906863870278 ) ) ;
#76519=CARTESIAN_POINT ( 'NONE',  ( 4.028611221114998919, 1516.744381837270112, 207.9874879615069858 ) ) ;
#76535=CARTESIAN_POINT ( 'NONE',  ( -1.121950782074999875, 1517.123342927159911, 214.1352753262870010 ) ) ;
#76538=CARTESIAN_POINT ( 'NONE',  ( -3.453544863754999472, 1517.106845464700200, 216.4586906126469898 ) ) ;
#76558=ORIENTED_EDGE ( 'NONE', *, *, #47228, .F. ) ;
#76583=ORIENTED_EDGE ( 'NONE', *, *, #91241, .F. ) ;
#76621=CARTESIAN_POINT ( 'NONE',  ( 7.326072144144999854, 1516.714320817460020, 208.3685457967989976 ) ) ;
#76652=CARTESIAN_POINT ( 'NONE',  ( -4.426491236972309729, 1508.728286123109910, 204.9619822988670137 ) ) ;
#76654=CARTESIAN_POINT ( 'NONE',  ( -6.949265684145000677, 1517.089216728169959, 205.6689289091970068 ) ) ;
#76703=CARTESIAN_POINT ( 'NONE',  ( -4.610938249504999753, 1516.815231249920089, 213.1623732742069990 ) ) ;
#76734=CARTESIAN_POINT ( 'NONE',  ( 15.20279577643499991, 1514.921193718960012, 194.6261569368670337 ) ) ;
#76750=CARTESIAN_POINT ( 'NONE',  ( -6.562635860634999929, 1517.111322026010157, 206.2508942643169974 ) ) ;
#76751=AXIS2_PLACEMENT_3D ( 'NONE', #51474, #18396, #103518 ) ;
#76765=CARTESIAN_POINT ( 'NONE',  ( 3.269184908365000197, 1516.940296199220029, 211.4060453336370244 ) ) ;
#76794=CARTESIAN_POINT ( 'NONE',  ( 7.326795523374999952, 1516.760434454289907, 203.3416138547669902 ) ) ;
#76795=CARTESIAN_POINT ( 'NONE',  ( -5.011551406145000165, 1517.080322339569875, 208.3849417611969841 ) ) ;
#76822=CARTESIAN_POINT ( 'NONE',  ( 1.931477262906880821, 1516.530173527225770, 216.8307695177551295 ) ) ;
#76843=VERTEX_POINT ( 'NONE', #28001 ) ;
#76844=CARTESIAN_POINT ( 'NONE',  ( -6.562635860634999929, 1517.111322026010157, 206.2508942643169974 ) ) ;
#76847=CARTESIAN_POINT ( 'NONE',  ( 7.141639577908946102, 1508.551704408428805, 214.6352815282469635 ) ) ;
#76866=CARTESIAN_POINT ( 'NONE',  ( -7.464251903891183204, 1516.685766403216121, 209.9631294702575701 ) ) ;
#76897=EDGE_CURVE ( 'NONE', #103079, #72815, #88343, .T. ) ;
#76898=CARTESIAN_POINT ( 'NONE',  ( 7.714371502985000184, 1516.738222552470233, 203.3422428319769892 ) ) ;
#76901=FACE_OUTER_BOUND ( 'NONE', #95116, .T. ) ;
#76924=CARTESIAN_POINT ( 'NONE',  ( 8.061256550655000908, 1512.677556571450168, 202.2106555494169982 ) ) ;
#76937=FACE_OUTER_BOUND ( 'NONE', #26380, .T. ) ;
#76939=CARTESIAN_POINT ( 'NONE',  ( 2.864326087304999824, 1516.826109302209943, 206.6287721023469999 ) ) ;
#76944=EDGE_CURVE ( 'NONE', #20905, #14138, #21956, .T. ) ;
#76947=CARTESIAN_POINT ( 'NONE',  ( 6.946514176795000495, 1512.024017243149956, 216.2067250139469934 ) ) ;
#76954=ADVANCED_FACE ( 'NONE', ( #102242 ), #63495, .T. ) ;
#76956=CARTESIAN_POINT ( 'NONE',  ( 1.131796810615000037, 1516.659138130710289, 214.8948242487770131 ) ) ;
#76960=CARTESIAN_POINT ( 'NONE',  ( 5.513200264406510342, 1508.884117426920056, 216.6305509554049991 ) ) ;
#76961=CARTESIAN_POINT ( 'NONE',  ( -6.546039433425000276, 1516.565291103010168, 211.4147861392469849 ) ) ;
#76979=ORIENTED_EDGE ( 'NONE', *, *, #21887, .T. ) ;
#76980=CARTESIAN_POINT ( 'NONE',  ( 2.869693458934999608, 1517.070197312179971, 203.3343689375869872 ) ) ;
#76998=ORIENTED_EDGE ( 'NONE', *, *, #51201, .F. ) ;
#77011=CARTESIAN_POINT ( 'NONE',  ( -8.325276424809809228, 1512.905891558365056, 216.5259404424210743 ) ) ;
#77029=CARTESIAN_POINT ( 'NONE',  ( -7.512750246095000861, 1509.038615934159907, 203.6084103740969908 ) ) ;
#77039=CARTESIAN_POINT ( 'NONE',  ( 7.407689794035296593, 1511.025938460391671, 202.7787461935695035 ) ) ;
#77061=CARTESIAN_POINT ( 'NONE',  ( 7.722536764694999611, 1517.050041317280147, 213.7387458049869906 ) ) ;
#77068=CARTESIAN_POINT ( 'NONE',  ( -5.784008673325000238, 1516.911981270829983, 204.1205073037870079 ) ) ;
#77071=EDGE_CURVE ( 'NONE', #78702, #46347, #7309, .T. ) ;
#77072=CARTESIAN_POINT ( 'NONE',  ( -2.182463115098289386, 1517.051704408389696, 216.8444262845050616 ) ) ;
#77084=VECTOR ( 'NONE', #103399, 1000.000000000000114 ) ;
#77085=CARTESIAN_POINT ( 'NONE',  ( 1.136004274065000041, 1516.815173273089840, 211.9874827793370287 ) ) ;
#77090=CARTESIAN_POINT ( 'NONE',  ( 2.284053471355000031, 1516.854133554269993, 207.9850318982369970 ) ) ;
#77106=CARTESIAN_POINT ( 'NONE',  ( 0.01306000193830150063, 1516.939762005280045, 213.7404293621069939 ) ) ;
#77115=AXIS2_PLACEMENT_3D ( 'NONE', #2749, #27923, #44183 ) ;
#77130=CARTESIAN_POINT ( 'NONE',  ( 7.112123000905755887, 1509.032357807246399, 202.3798014945801640 ) ) ;
#77184=CARTESIAN_POINT ( 'NONE',  ( -7.591975382166549657, 1510.802068165409992, 214.6174606883600120 ) ) ;
#77190=CARTESIAN_POINT ( 'NONE',  ( 4.625789976465000564, 1517.104192383289956, 210.2432295619669844 ) ) ;
#77199=CARTESIAN_POINT ( 'NONE',  ( -15.16689671995240118, 1513.426431440490205, 223.4767850746570161 ) ) ;
#77209=CARTESIAN_POINT ( 'NONE',  ( -5.775165567126295585, 1509.036904579127395, 216.6345513647860344 ) ) ;
#77224=CARTESIAN_POINT ( 'NONE',  ( 6.546951682585000043, 1516.606339319019980, 206.2472570094369928 ) ) ;
#77225=ORIENTED_EDGE ( 'NONE', *, *, #79903, .T. ) ;
#77229=EDGE_LOOP ( 'NONE', ( #54490, #68123, #54802, #55214 ) ) ;
#77273=CARTESIAN_POINT ( 'NONE',  ( -1.120543735785000106, 1517.073005577650065, 213.1661658574570026 ) ) ;
#77314=CARTESIAN_POINT ( 'NONE',  ( -4.043366258305000294, 1516.951766529250108, 206.2549880390970145 ) ) ;
#77322=CARTESIAN_POINT ( 'NONE',  ( -16.60142423921517718, 1513.050501378448644, 221.1601934794027784 ) ) ;
#77326=CARTESIAN_POINT ( 'NONE',  ( -1.118353254094999860, 1516.977201124959947, 211.6155430111569729 ) ) ;
#77348=CARTESIAN_POINT ( 'NONE',  ( 7.167019213074620865, 1508.551563895499839, 203.6086053948930044 ) ) ;
#77353=CARTESIAN_POINT ( 'NONE',  ( 4.613762356885000138, 1516.939574742129935, 203.3372076122869885 ) ) ;
#77354=CARTESIAN_POINT ( 'NONE',  ( -2.873919040654999701, 1516.940252185109784, 209.1351185066319829 ) ) ;
#77355=ORIENTED_EDGE ( 'NONE', *, *, #106261, .F. ) ;
#77357=CARTESIAN_POINT ( 'NONE',  ( 3.605887597328768290, 1511.586661999378066, 217.1930125735252943 ) ) ;
#77390=CARTESIAN_POINT ( 'NONE',  ( -15.69395960576500038, 1511.900571936589813, 221.5073600987669806 ) ) ;
#77391=CARTESIAN_POINT ( 'NONE',  ( 3.424720300894999792, 1517.051704408389924, 200.5840233334270124 ) ) ;
#77396=CARTESIAN_POINT ( 'NONE',  ( -7.725990199955000470, 1517.181921232829836, 206.6366402828969910 ) ) ;
#77409=CARTESIAN_POINT ( 'NONE',  ( -2.689982596155000127, 1512.192993275409890, 201.4357459275669839 ) ) ;
#77447=CARTESIAN_POINT ( 'NONE',  ( 5.000083827734999709, 1516.858456333729919, 204.1129977322069919 ) ) ;
#77466=EDGE_CURVE ( 'NONE', #49508, #21931, #87228, .T. ) ;
#77471=CARTESIAN_POINT ( 'NONE',  ( 5.012317068235000228, 1517.020727862619879, 211.9902797687369969 ) ) ;
#77475=CARTESIAN_POINT ( 'NONE',  ( 7.503873103355000573, 1512.035910181040208, 202.5568695388469962 ) ) ;
#77485=CARTESIAN_POINT ( 'NONE',  ( -6.554151464375000735, 1516.906641539930206, 216.4536580562070185 ) ) ;
#77486=CARTESIAN_POINT ( 'NONE',  ( -8.302057905577099106, 1511.419855272942868, 213.4520019170473688 ) ) ;
#77490=DIRECTION ( 'NONE',  ( 0.000000000000000000, -6.123233995736769734E-17, -1.000000000000000000 ) ) ;
#77492=CARTESIAN_POINT ( 'NONE',  ( -6.949574985774999547, 1517.102359858469754, 205.8627441332170065 ) ) ;
#77498=CARTESIAN_POINT ( 'NONE',  ( 8.118882928225001905, 1514.642928591849795, 215.6564664142569825 ) ) ;
#77500=ORIENTED_EDGE ( 'NONE', *, *, #29200, .T. ) ;
#77506=CARTESIAN_POINT ( 'NONE',  ( -2.480813923114999930, 1517.051603658920158, 214.1347848340070072 ) ) ;
#77512=CARTESIAN_POINT ( 'NONE',  ( -2.864326125434999870, 1516.826109302209943, 211.6149197999869784 ) ) ;
#77530=CARTESIAN_POINT ( 'NONE',  ( -7.721907926364999675, 1517.026025493960105, 204.1173703575669833 ) ) ;
#77571=CARTESIAN_POINT ( 'NONE',  ( 7.075014806132906564, 1516.558166122959847, 206.6310126780043674 ) ) ;
#77587=CARTESIAN_POINT ( 'NONE',  ( 7.519244400428443775, 1510.642476670986071, 203.1920689657892751 ) ) ;
#77607=CARTESIAN_POINT ( 'NONE',  ( 2.877744946244999991, 1516.723920667490120, 213.7309102736070088 ) ) ;
#77612=CARTESIAN_POINT ( 'NONE',  ( -5.007588685045000432, 1516.804776704140068, 203.3466091393569855 ) ) ;
#77626=CARTESIAN_POINT ( 'NONE',  ( 6.561995960394999550, 1517.083030555940013, 212.3803205491769859 ) ) ;
#77631=CARTESIAN_POINT ( 'NONE',  ( -7.724874651314999952, 1517.139320148880188, 208.3815253650730028 ) ) ;
#77646=CARTESIAN_POINT ( 'NONE',  ( 4.621267883935000320, 1516.830644417779922, 214.1213023606370029 ) ) ;
#77649=CARTESIAN_POINT ( 'NONE',  ( -2.872208748294999836, 1517.145312756229941, 216.4596396827270155 ) ) ;
#77654=ORIENTED_EDGE ( 'NONE', *, *, #84206, .F. ) ;
#77678=CARTESIAN_POINT ( 'NONE',  ( -7.550503362009299835, 1510.480349264700180, 214.6730346447039892 ) ) ;
#77684=CARTESIAN_POINT ( 'NONE',  ( -1.146118350564959920, 1516.628317670959859, 201.4103523897319974 ) ) ;
#77725=CARTESIAN_POINT ( 'NONE',  ( -7.921235470229449405, 1511.346448533420016, 214.8276827278679662 ) ) ;
#77732=CARTESIAN_POINT ( 'NONE',  ( -0.7402208985179988820, 1516.992029636990083, 209.8751463226419958 ) ) ;
#77750=CARTESIAN_POINT ( 'NONE',  ( -6.951517170504999399, 1517.194816588360027, 207.9969518818670053 ) ) ;
#77756=CARTESIAN_POINT ( 'NONE',  ( -1.906499846882070084E-08, 1517.051704408389924, 209.1218459511669892 ) ) ;
#77765=CARTESIAN_POINT ( 'NONE',  ( 7.322709686834999232, 1516.596789218710001, 205.8608388005369818 ) ) ;
#77771=CARTESIAN_POINT ( 'NONE',  ( 4.490619199204468615, 1508.909942010298437, 212.6094383991669758 ) ) ;
#77814=CARTESIAN_POINT ( 'NONE',  ( 0.7572979362240020995, 1516.829948096479939, 212.5714934102470011 ) ) ;
#77827=AXIS2_PLACEMENT_3D ( 'NONE', #101375, #67826, #42608 ) ;
#77844=ORIENTED_EDGE ( 'NONE', *, *, #105503, .F. ) ;
#77849=ADVANCED_FACE ( 'NONE', ( #19212 ), #3576, .T. ) ;
#77857=CARTESIAN_POINT ( 'NONE',  ( -1.717084749545000122, 1516.819260244609950, 206.6456753351970121 ) ) ;
#77870=CARTESIAN_POINT ( 'NONE',  ( 5.787476994515000861, 1517.070197312179971, 211.9915394291670054 ) ) ;
#77892=CARTESIAN_POINT ( 'NONE',  ( 7.096077594474770933, 1508.610125823030103, 202.4734937754249984 ) ) ;
#77898=CARTESIAN_POINT ( 'NONE',  ( -0.7543882209519990889, 1516.727502608469877, 202.5709757879969857 ) ) ;
#77899=CARTESIAN_POINT ( 'NONE',  ( 5.006259848694999626, 1516.939723362869927, 209.1089481433290018 ) ) ;
#77934=CARTESIAN_POINT ( 'NONE',  ( -16.61115978156500006, 1513.007288725350008, 221.0814365924669858 ) ) ;
#77938=CARTESIAN_POINT ( 'NONE',  ( -5.012938901904998801, 1517.051603658920158, 206.6410320471169939 ) ) ;
#77956=CARTESIAN_POINT ( 'NONE',  ( -3.165841394545000131, 1511.802450769970164, 201.1846294787470129 ) ) ;
#77982=CARTESIAN_POINT ( 'NONE',  ( -3.034964906435000387, 1517.051704408389924, 217.3038049130670117 ) ) ;
#77989=CARTESIAN_POINT ( 'NONE',  ( 4.030514512585000375, 1516.901952101700090, 204.4990030879170320 ) ) ;
#78010=CARTESIAN_POINT ( 'NONE',  ( 0.01327253640020150012, 1516.940252185109784, 211.9957649727570015 ) ) ;
#78013=CARTESIAN_POINT ( 'NONE',  ( 7.084879043715000435, 1512.024017243130174, 202.1753317553169893 ) ) ;
#78018=EDGE_CURVE ( 'NONE', #56695, #78578, #62088, .T. ) ;
#78019=CARTESIAN_POINT ( 'NONE',  ( -8.297002917174999936, 1511.752511073100095, 215.1658660083070060 ) ) ;
#78021=CARTESIAN_POINT ( 'NONE',  ( -7.550503362009299835, 1510.480349264700180, 214.6730346447039892 ) ) ;
#78023=CARTESIAN_POINT ( 'NONE',  ( -3.453544863754999472, 1517.106845464700200, 216.4586906126469898 ) ) ;
#78030=CARTESIAN_POINT ( 'NONE',  ( -2.493699806765000027, 1516.858326417339867, 206.6451124560869914 ) ) ;
#78039=CARTESIAN_POINT ( 'NONE',  ( -6.150613017182610776, 1511.023286695659863, 201.6389880435640123 ) ) ;
#78045=CARTESIAN_POINT ( 'NONE',  ( -7.326795561505000443, 1516.760434454289907, 214.9020780475669881 ) ) ;
#78051=CARTESIAN_POINT ( 'NONE',  ( 3.269184908365000197, 1516.940296199220029, 211.4060453336370244 ) ) ;
#78071=CARTESIAN_POINT ( 'NONE',  ( 4.031142351675000235, 1516.929569650079884, 204.1114229688670036 ) ) ;
#78090=EDGE_CURVE ( 'NONE', #40123, #63057, #93043, .T. ) ;
#78123=CARTESIAN_POINT ( 'NONE',  ( 7.459190098609637332, 1510.844697587253677, 202.9343248737379781 ) ) ;
#78147=CARTESIAN_POINT ( 'NONE',  ( -3.254401441735000233, 1516.919782530640077, 213.1645757730269963 ) ) ;
#78148=CARTESIAN_POINT ( 'NONE',  ( 3.385713881024999594, 1511.191277613550028, 216.7448064569670123 ) ) ;
#78152=CARTESIAN_POINT ( 'NONE',  ( -3.457266643525000127, 1516.691414181030041, 203.3491180233569935 ) ) ;
#78155=CARTESIAN_POINT ( 'NONE',  ( -2.234923082067399758, 1512.341036938790012, 201.5226187867249905 ) ) ;
#78166=CARTESIAN_POINT ( 'NONE',  ( -6.546951720715000533, 1516.606339319019980, 211.9964348928969855 ) ) ;
#78168=VECTOR ( 'NONE', #52091, 1000.000000000000000 ) ;
#78169=CARTESIAN_POINT ( 'NONE',  ( 17.05938516367379876, 1517.051704408300111, 223.0487112149370148 ) ) ;
#78173=CARTESIAN_POINT ( 'NONE',  ( -0.7559395363919990674, 1516.972341476009888, 207.9998125401569951 ) ) ;
#78177=( BOUNDED_CURVE ( )  B_SPLINE_CURVE ( 3, ( #100093, #4925, #6034, #56449 ),
 .UNSPECIFIED., .F., .T. ) 
 B_SPLINE_CURVE_WITH_KNOTS ( ( 4, 4 ),
 ( 0.5395807524062695704, 1.539014399150256507 ),
 .UNSPECIFIED. ) 
 CURVE ( )  GEOMETRIC_REPRESENTATION_ITEM ( )  RATIONAL_B_SPLINE_CURVE ( ( 1.000000000000000000, 0.9184788592064836443, 0.9184788592064836443, 1.000000000000000000 ) ) 
 REPRESENTATION_ITEM ( '' )  );
#78190=CARTESIAN_POINT ( 'NONE',  ( 3.456007385174999946, 1516.647534046129977, 215.6697273451470096 ) ) ;
#78193=CARTESIAN_POINT ( 'NONE',  ( -2.291514335905000088, 1517.194972660189933, 216.8481778957070105 ) ) ;
#78200=EDGE_CURVE ( 'NONE', #8750, #107607, #27499, .T. ) ;
#78201=CARTESIAN_POINT ( 'NONE',  ( 7.558973819147550621, 1511.169205552290123, 203.0547742380890099 ) ) ;
#78230=CARTESIAN_POINT ( 'NONE',  ( -2.589417882402239801, 1516.541553964140121, 201.4126244432099782 ) ) ;
#78274=CARTESIAN_POINT ( 'NONE',  ( -5.775625115495000017, 1516.745833913490060, 209.8771724060850090 ) ) ;
#78276=CARTESIAN_POINT ( 'NONE',  ( -7.269615836804730336, 1508.603735221707211, 203.6084103740970193 ) ) ;
#78285=CARTESIAN_POINT ( 'NONE',  ( 6.554778533645000849, 1516.929962200689943, 201.4024535497269994 ) ) ;
#78292=CARTESIAN_POINT ( 'NONE',  ( 4.031168767865001001, 1516.805675336850072, 208.3649472324300120 ) ) ;
#78299=DIRECTION ( 'NONE',  ( 0.000000000000000000, -1.000000000000000000, 6.123233995736769734E-17 ) ) ;
#78310=CARTESIAN_POINT ( 'NONE',  ( -4.624099329465000352, 1516.962555622980062, 205.8665050058069994 ) ) ;
#78335=CARTESIAN_POINT ( 'NONE',  ( -5.774609660074999873, 1516.777260590120022, 213.7418541773069762 ) ) ;
#78342=ADVANCED_FACE ( 'NONE', ( #94992 ), #44043, .T. ) ;
#78366=CARTESIAN_POINT ( 'NONE',  ( -1.702754409475000008, 1517.014196759610059, 212.5856132281170119 ) ) ;
#78369=CARTESIAN_POINT ( 'NONE',  ( -8.181958980964999739, 1517.051704408389924, 206.0868810637969943 ) ) ;
#78404=CARTESIAN_POINT ( 'NONE',  ( -7.079928805590961716, 1516.557407140219766, 211.5970724783486219 ) ) ;
#78409=CARTESIAN_POINT ( 'NONE',  ( 3.251611325815000342, 1516.779243033999819, 206.8234764622770001 ) ) ;
#78418=VERTEX_POINT ( 'NONE', #54673 ) ;
#78420=CARTESIAN_POINT ( 'NONE',  ( 9.638115859579080791, 1516.551188146539971, 214.4931927712729873 ) ) ;
#78424=CARTESIAN_POINT ( 'NONE',  ( -3.252530653725000054, 1516.827328999679821, 212.0018028951869837 ) ) ;
#78446=CARTESIAN_POINT ( 'NONE',  ( 7.320051246071350270, 1508.610505975320166, 203.0404454350509695 ) ) ;
#78451=CARTESIAN_POINT ( 'NONE',  ( -2.487103457664999961, 1516.577434278289957, 202.5755431900869894 ) ) ;
#78452=CARTESIAN_POINT ( 'NONE',  ( -7.713648872314999849, 1516.710624944440042, 209.8745175203999906 ) ) ;
#78455=ADVANCED_FACE ( 'NONE', ( #71491 ), #61973, .F. ) ;
#78487=CARTESIAN_POINT ( 'NONE',  ( -7.821732098484999618, 1516.863303996349941, 201.3872288444869980 ) ) ;
#78488=CARTESIAN_POINT ( 'NONE',  ( 11.28295019303499913, 1512.609537213029853, 225.3524656301670177 ) ) ;
#78492=CARTESIAN_POINT ( 'NONE',  ( -15.78856002036499717, 1512.525301340740043, 222.7193983515670084 ) ) ;
#78496=CARTESIAN_POINT ( 'NONE',  ( -0.01327257453019850021, 1516.940252185109784, 206.2479269295770052 ) ) ;
#78525=CARTESIAN_POINT ( 'NONE',  ( -15.93623144086499899, 1516.904916668740043, 193.9453790007669909 ) ) ;
#78540=CARTESIAN_POINT ( 'NONE',  ( -6.961841786822310141, 1508.551566289579796, 215.6737177159799899 ) ) ;
#78548=CARTESIAN_POINT ( 'NONE',  ( 1.705466410464999916, 1517.120861839400050, 204.1076508302870138 ) ) ;
#78571=CARTESIAN_POINT ( 'NONE',  ( 0.7574259850960020080, 1516.837969789639828, 212.3776558342370038 ) ) ;
#78574=CARTESIAN_POINT ( 'NONE',  ( 6.124171326874999544, 1514.216129015430170, 201.4528617218270199 ) ) ;
#78578=VERTEX_POINT ( 'NONE', #46820 ) ;
#78585=AXIS2_PLACEMENT_3D ( 'NONE', #104525, #3201, #2645 ) ;
#78592=CARTESIAN_POINT ( 'NONE',  ( -1.717084749545000122, 1516.819260244609950, 206.6456753351970121 ) ) ;
#78597=CARTESIAN_POINT ( 'NONE',  ( -6.827666136118519802, 1508.551704606160001, 202.6664247900299927 ) ) ;
#78609=CARTESIAN_POINT ( 'NONE',  ( 1.132949076425000090, 1516.693851263360102, 214.1195642086070166 ) ) ;
#78611=CARTESIAN_POINT ( 'NONE',  ( 5.762402162469949296, 1511.083508941950186, 216.8055985269170094 ) ) ;
#78614=CARTESIAN_POINT ( 'NONE',  ( 3.461995158685000185, 1516.906233342200039, 211.9877574868770012 ) ) ;
#78623=CARTESIAN_POINT ( 'NONE',  ( -7.548380910495000151, 1510.399296111369949, 213.9269235281369959 ) ) ;
#78631=CARTESIAN_POINT ( 'NONE',  ( -7.333070173014999860, 1516.955859323880077, 203.3428461583270064 ) ) ;
#78665=EDGE_LOOP ( 'NONE', ( #58546, #99736, #26591, #62865 ) ) ;
#78674=CARTESIAN_POINT ( 'NONE',  ( 3.454172615424999648, 1517.122088787240045, 201.3974225380069925 ) ) ;
#78678=CARTESIAN_POINT ( 'NONE',  ( 7.599119408734999581, 1512.336926113599930, 206.7298288840769942 ) ) ;
#78696=SURFACE_STYLE_USAGE ( .BOTH. , #97695 ) ;
#78702=VERTEX_POINT ( 'NONE', #22654 ) ;
#78710=CARTESIAN_POINT ( 'NONE',  ( 7.334328272665000092, 1517.005755693489846, 214.1256940922069987 ) ) ;
#78711=CARTESIAN_POINT ( 'NONE',  ( 3.077691717124999560, 1511.730395268069969, 216.9250477754170277 ) ) ;
#78715=CARTESIAN_POINT ( 'NONE',  ( -3.263521942484999716, 1516.676340709600026, 203.3494421577970002 ) ) ;
#78720=CARTESIAN_POINT ( 'NONE',  ( -0.01010286742719850028, 1516.939452820819952, 201.4022050290969901 ) ) ;
#78731=CARTESIAN_POINT ( 'NONE',  ( 1.135460316954999938, 1516.790374942449944, 212.3751473514870156 ) ) ;
#78736=CARTESIAN_POINT ( 'NONE',  ( 7.337297311985000015, 1517.135701590510052, 209.8615382079770200 ) ) ;
#78752=CARTESIAN_POINT ( 'NONE',  ( -6.552897405075000847, 1516.858146885269889, 215.6784973415170157 ) ) ;
#78763=CARTESIAN_POINT ( 'NONE',  ( 7.920874050670489552, 1511.346048414110101, 203.4159230979989843 ) ) ;
#78775=LINE ( 'NONE', #104523, #40316 ) ;
#78782=B_SPLINE_CURVE_WITH_KNOTS ( 'NONE', 3,
 ( #5261, #6906, #99297, #91475, #39414, #15829, #65186, #50032, #14198, #73591, #41063, #32667, #38849, #31006, #75240, #4706, #73028, #22572, #13631, #57350, #98763, #22024, #66845, #58431, #109390, #48385, #56776, #92559, #82527 ),
 .UNSPECIFIED., .F., .F.,
 ( 4, 2, 2, 1, 1, 2, 2, 2, 2, 2, 2, 2, 1, 2, 2, 4 ),
 ( 0.000000000000000000, 0.1250000000005312417, 0.1875000000007969181, 0.2187500000009944268, 0.2343750000010931256, 0.2421875000011424472, 0.2500000000011917689, 0.3750000000012347345, 0.4375000000011303736, 0.5000000000010259571, 0.6250000000013459234, 0.6875000000015057955, 0.7187500000017689183, 0.7343750000019237945, 0.7500000000020786706, 1.000000000000000000 ),
 .UNSPECIFIED. ) ;
#78792=CARTESIAN_POINT ( 'NONE',  ( -2.100767134424469607, 1516.527474870850256, 201.4129930513860245 ) ) ;
#78806=B_SPLINE_CURVE_WITH_KNOTS ( 'NONE', 3,
 ( #14962, #46961, #39066, #73245, #5481, #97873, #56448, #4398, #21148, #40185, #55355, #81081, #64313, #47497, #89488, #90027, #38526, #13860, #63760, #98976, #57010, #12783, #31231, #72703, #73810, #23374, #30681, #55909, #72172, #48607, #106828, #22804, #4924, #30118, #98432, #107385, #22250, #21704, #99519, #13304, #65967, #106290, #91138, #57565, #48044, #49157, #31780, #90580, #14415, #82183, #83289, #6587, #60308, #23911, #50265, #84926, #8219, #92787, #84394, #86047, #26118 ),
 .UNSPECIFIED., .F., .F.,
 ( 4, 3, 3, 3, 3, 3, 3, 3, 3, 3, 3, 3, 3, 3, 3, 3, 3, 3, 3, 3, 4 ),
 ( 7.020647373213010134, 7.318242487455970391, 7.663999848964880179, 7.934526232592060246, 8.156304087536639713, 8.278825267203739457, 8.449185380093728881, 8.482857723717689424, 8.514868418927969529, 8.765148280566069872, 9.022911409362329493, 9.297145710536121044, 9.587002469640040658, 9.900769533069599504, 10.04480025696140011, 10.11612467641749902, 10.52133809873689962, 10.85847357495339871, 11.00458707344359865, 11.32809206207529940, 11.65159705070689888 ),
 .UNSPECIFIED. ) ;
#78808=B_SPLINE_CURVE_WITH_KNOTS ( 'NONE', 3,
 ( #107297, #3769, #63676, #13215, #97787, #21063, #81527, #73722, #39547, #22707, #56905, #88849, #98342, #38975, #38431, #74273, #90489, #40091, #30025, #20514, #4829, #37903, #89400, #46869, #12688, #28950, #72607, #63139, #97240, #30591, #54722, #72084, #98889, #4304, #91038, #31134, #46326, #21615, #64218, #14325, #82654, #22157, #73153, #56357, #48515, #13764, #5946, #47948, #12134, #80997, #82088, #106737, #5390, #107845, #65319 ),
 .UNSPECIFIED., .F., .F.,
 ( 4, 3, 3, 3, 3, 3, 3, 3, 3, 3, 3, 3, 3, 3, 3, 3, 3, 3, 4 ),
 ( 9.902195898209999569, 10.17210527304969858, 10.45530577765890001, 10.70141353110000004, 11.00396970312500144, 11.32322756693239896, 11.52456852350000105, 11.84989040643209890, 12.16242387753359999, 12.38020728900000123, 12.74551463662050033, 13.12275145103740037, 13.53252099862019975, 13.95359103776459975, 14.40783883235129892, 14.91487510228819957, 15.44821056779149870, 15.94145638527190023, 16.40090783169999966 ),
 .UNSPECIFIED. ) ;
#78842=ORIENTED_EDGE ( 'NONE', *, *, #24948, .T. ) ;
#78846=CARTESIAN_POINT ( 'NONE',  ( 3.460866170685000132, 1517.020847257979995, 209.8575449048190080 ) ) ;
#78848=CARTESIAN_POINT ( 'NONE',  ( 7.012921650808690899, 1508.551704408389696, 202.7299073050613174 ) ) ;
#78860=DIRECTION ( 'NONE',  ( 0.4999999999998399614, 0.7071067811867740582, 0.4999999999998399614 ) ) ;
#78868=CARTESIAN_POINT ( 'NONE',  ( -3.462835665494999660, 1517.038650117239968, 208.0021282158369900 ) ) ;
#78885=CARTESIAN_POINT ( 'NONE',  ( -5.786527600464999033, 1517.025653221279981, 205.6708125431369751 ) ) ;
#78902=CARTESIAN_POINT ( 'NONE',  ( 2.877113070465000089, 1516.697242742309982, 214.1184881303969973 ) ) ;
#78925=LINE ( 'NONE', #61573, #99645 ) ;
#78967=ADVANCED_FACE ( 'NONE', ( #108073 ), #21290, .T. ) ;
#78976=CARTESIAN_POINT ( 'NONE',  ( -7.211758761846644106, 1516.538242702012212, 211.1938241164952217 ) ) ;
#78981=CARTESIAN_POINT ( 'NONE',  ( -4.625693903144999730, 1517.042661899400173, 206.8353996064669786 ) ) ;
#78983=( GEOMETRIC_REPRESENTATION_CONTEXT ( 3 ) GLOBAL_UNCERTAINTY_ASSIGNED_CONTEXT ( ( #97207 ) ) GLOBAL_UNIT_ASSIGNED_CONTEXT ( ( #106100, #88755, #36690 ) ) REPRESENTATION_CONTEXT ( 'NONE', 'WORKASPACE' ) );
#78990=CARTESIAN_POINT ( 'NONE',  ( 13.07344732962040013, 1516.551188146170034, 192.4513774157680075 ) ) ;
#78994=CARTESIAN_POINT ( 'NONE',  ( 5.011678838024999472, 1516.989560013210166, 212.3778133565769792 ) ) ;
#79000=FACE_OUTER_BOUND ( 'NONE', #56792, .T. ) ;
#79022=CARTESIAN_POINT ( 'NONE',  ( -2.292940207144999576, 1516.565291103010168, 202.5758065368070220 ) ) ;
#79023=CARTESIAN_POINT ( 'NONE',  ( 5.014195101815000832, 1517.120861839400050, 210.8273123806970091 ) ) ;
#79044=CARTESIAN_POINT ( 'NONE',  ( -7.855404022624998817, 1514.254015528259970, 202.3343151538169877 ) ) ;
#79047=VECTOR ( 'NONE', #80827, 1000.000000000000114 ) ;
#79058=CARTESIAN_POINT ( 'NONE',  ( 12.18811178233499959, 1511.857118786289902, 224.3850700526670039 ) ) ;
#79066=CARTESIAN_POINT ( 'NONE',  ( -4.624736897314999595, 1516.994127245590107, 206.2540423059970180 ) ) ;
#79083=CARTESIAN_POINT ( 'NONE',  ( 5.551188674472009588, 1510.480349264700180, 216.6723492941099778 ) ) ;
#79116=CARTESIAN_POINT ( 'NONE',  ( -7.334957394705000411, 1517.030858226499959, 204.5055736355369902 ) ) ;
#79137=CARTESIAN_POINT ( 'NONE',  ( -2.284199401535000007, 1516.940296199220029, 212.3910308785969789 ) ) ;
#79159=CARTESIAN_POINT ( 'NONE',  ( 2.476450664134999702, 1516.843453247299749, 206.8221896160070230 ) ) ;
#79165=CARTESIAN_POINT ( 'NONE',  ( -6.769697780263440379, 1509.032013233849966, 201.8557327794140122 ) ) ;
#79169=CARTESIAN_POINT ( 'NONE',  ( 15.18091657867779887, 1512.335564144490036, 196.2297506243189957 ) ) ;
#79178=CARTESIAN_POINT ( 'NONE',  ( 7.718134629434999283, 1516.881930554049859, 216.4517759834270123 ) ) ;
#79180=CARTESIAN_POINT ( 'NONE',  ( 5.554947007364200218, 1511.433089852210060, 217.3313357707569935 ) ) ;
#79182=CARTESIAN_POINT ( 'NONE',  ( 1.135460316954999938, 1516.790374942449944, 212.3751473514870156 ) ) ;
#79199=CARTESIAN_POINT ( 'NONE',  ( 2.480813884984999884, 1517.051603658920158, 204.1089070683270279 ) ) ;
#79213=ORIENTED_EDGE ( 'NONE', *, *, #50102, .T. ) ;
#79239=CARTESIAN_POINT ( 'NONE',  ( 5.778999773775000293, 1516.955859323880077, 201.7887757972170277 ) ) ;
#79242=FACE_OUTER_BOUND ( 'NONE', #79959, .T. ) ;
#79253=CARTESIAN_POINT ( 'NONE',  ( -7.669726197924999767, 1510.984078637139874, 213.9427911786070240 ) ) ;
#79271=CARTESIAN_POINT ( 'NONE',  ( -7.714371541114999786, 1516.738222552470233, 214.9014490703569891 ) ) ;
#79272=CARTESIAN_POINT ( 'NONE',  ( 2.325731103684999912, 1511.751588929339960, 216.7056378762670192 ) ) ;
#79278=CARTESIAN_POINT ( 'NONE',  ( 2.480187016714999970, 1517.025470194390209, 204.4964864072570094 ) ) ;
#79283=CARTESIAN_POINT ( 'NONE',  ( -11.75640701318574699, 1511.791180387471059, 193.9413991097462997 ) ) ;
#79286=DIRECTION ( 'NONE',  ( -1.000000000000000000, 0.000000000000000000, 0.000000000000000000 ) ) ;
#79291=CARTESIAN_POINT ( 'NONE',  ( -2.282915221395000138, 1516.876240617270014, 211.6158662526670184 ) ) ;
#79296=CARTESIAN_POINT ( 'NONE',  ( -4.618583430005000601, 1516.939762005280045, 209.1349059721700030 ) ) ;
#79305=( BOUNDED_CURVE ( )  B_SPLINE_CURVE ( 3, ( #103916, #33947, #86011, #102788 ),
 .UNSPECIFIED., .F., .T. ) 
 B_SPLINE_CURVE_WITH_KNOTS ( ( 4, 4 ),
 ( 4.424142070271249949, 5.579787944462250238 ),
 .UNSPECIFIED. ) 
 CURVE ( )  GEOMETRIC_REPRESENTATION_ITEM ( )  RATIONAL_B_SPLINE_CURVE ( ( 1.000000000000000000, 0.8917691662044565648, 0.8917691662044565648, 1.000000000000000000 ) ) 
 REPRESENTATION_ITEM ( '' )  );
#79311=CARTESIAN_POINT ( 'NONE',  ( -7.328049318385000177, 1516.809497469189864, 215.6772390872569929 ) ) ;
#79318=ORIENTED_EDGE ( 'NONE', *, *, #76138, .T. ) ;
#79342=CARTESIAN_POINT ( 'NONE',  ( -7.703229051499217661, 1511.126521620429685, 214.5635182500827511 ) ) ;
#79348=CARTESIAN_POINT ( 'NONE',  ( -2.152805114430509814, 1516.527314490149820, 201.4129972511030076 ) ) ;
#79378=LINE ( 'NONE', #3246, #21215 ) ;
#79393=CARTESIAN_POINT ( 'NONE',  ( 0.007128837152181529378, 1517.006509894990131, 209.8686634857439799 ) ) ;
#79398=LINE ( 'NONE', #96754, #80502 ) ;
#79403=CARTESIAN_POINT ( 'NONE',  ( 5.779627054084999216, 1516.977993847330026, 201.4011957967969977 ) ) ;
#79408=ORIENTED_EDGE ( 'NONE', *, *, #81624, .T. ) ;
#79410=CARTESIAN_POINT ( 'NONE',  ( -7.339107240745000205, 1517.203017563489766, 207.9963360818169917 ) ) ;
#79428=CARTESIAN_POINT ( 'NONE',  ( 4.995725969715000048, 1516.651306816259876, 206.8263604310569690 ) ) ;
#79445=CARTESIAN_POINT ( 'NONE',  ( 7.331812085974999782, 1516.906641539930206, 215.6759973964769870 ) ) ;
#79452=CARTESIAN_POINT ( 'NONE',  ( 4.486733114842439640, 1517.051705360449887, 201.5292726349509849 ) ) ;
#79469=CARTESIAN_POINT ( 'NONE',  ( -5.775166187770511605, 1509.036904563493863, 201.6091405521827937 ) ) ;
#79490=EDGE_LOOP ( 'NONE', ( #107258, #83856, #76128, #107766 ) ) ;
#79516=CARTESIAN_POINT ( 'NONE',  ( -6.287493054558040306, 1516.709230591747882, 213.2274840498923254 ) ) ;
#79519=DIRECTION ( 'NONE',  ( -0.8236474686107856380, -0.5669078173018518019, -0.01484500364079635246 ) ) ;
#79520=CARTESIAN_POINT ( 'NONE',  ( -7.726331963605000297, 1517.194972660189933, 206.8303316343270239 ) ) ;
#79533=CARTESIAN_POINT ( 'NONE',  ( 7.337793712495000342, 1517.145312756229941, 211.9940546803969994 ) ) ;
#79542=CARTESIAN_POINT ( 'NONE',  ( 14.79241649771974743, 1514.564622118912894, 225.3747096568645816 ) ) ;
#79546=VECTOR ( 'NONE', #18957, 1000.000000000000227 ) ;
#79558=CARTESIAN_POINT ( 'NONE',  ( 6.140127931138819939, 1508.880864730590019, 201.6144229198349933 ) ) ;
#79564=CARTESIAN_POINT ( 'NONE',  ( 4.030514512585000375, 1516.901952101700090, 204.4990030879170320 ) ) ;
#79586=CARTESIAN_POINT ( 'NONE',  ( -6.809551170575000256, 1512.240414293130016, 201.8588037525169909 ) ) ;
#79612=CARTESIAN_POINT ( 'NONE',  ( -2.494020320564999782, 1516.876240617270014, 206.8389307488369866 ) ) ;
#79631=CARTESIAN_POINT ( 'NONE',  ( 5.929777003983391914, 1510.642476694421475, 216.6410903641369146 ) ) ;
#79648=FACE_OUTER_BOUND ( 'NONE', #53964, .T. ) ;
#79650=AXIS2_PLACEMENT_3D ( 'NONE', #62155, #86773, #35827 ) ;
#79667=CARTESIAN_POINT ( 'NONE',  ( -3.265407155974999753, 1516.754149861460064, 204.5121726906670006 ) ) ;
#79686=CARTESIAN_POINT ( 'NONE',  ( -3.253141175365000137, 1516.858171774179937, 212.3894494859370070 ) ) ;
#79708=CARTESIAN_POINT ( 'NONE',  ( 0.7352271172030020452, 1516.963431999339946, 207.4067364850470199 ) ) ;
#79714=CARTESIAN_POINT ( 'NONE',  ( -7.512715662404939820, 1509.034509512849809, 202.9804584623499863 ) ) ;
#79720=CARTESIAN_POINT ( 'NONE',  ( -6.375350519788010040, 1511.068351247050032, 201.7267438082049864 ) ) ;
#79725=CARTESIAN_POINT ( 'NONE',  ( 3.330134165755000097, 1515.051704408389924, 204.7920544413669859 ) ) ;
#79726=CARTESIAN_POINT ( 'NONE',  ( 1.130002494264999990, 1516.621991115350056, 216.0576472317669925 ) ) ;
#79728=CARTESIAN_POINT ( 'NONE',  ( 6.044713202946720543, 1511.753217516670247, 217.4189031040939994 ) ) ;
#79730=CARTESIAN_POINT ( 'NONE',  ( 2.298369469825000344, 1516.779243033999819, 212.3734572960470075 ) ) ;
#79749=CARTESIAN_POINT ( 'NONE',  ( 7.713117802984999827, 1516.690345681169902, 204.1174038931170003 ) ) ;
#79789=CARTESIAN_POINT ( 'NONE',  ( -11.02428140916500077, 1512.359593911809952, 193.2458125109669993 ) ) ;
#79806=CARTESIAN_POINT ( 'NONE',  ( -8.170896261794998949, 1511.354819475749991, 213.9493513980370096 ) ) ;
#79825=CARTESIAN_POINT ( 'NONE',  ( 5.782749401605000727, 1516.858301627840092, 214.8983370654769942 ) ) ;
#79826=CARTESIAN_POINT ( 'NONE',  ( 2.892503378805000303, 1511.980236064749988, 216.8996406803269963 ) ) ;
#79832=CARTESIAN_POINT ( 'NONE',  ( 1.703779605225000049, 1517.057265928030120, 205.0766634521770015 ) ) ;
#79844=CARTESIAN_POINT ( 'NONE',  ( -2.478306858074999841, 1516.938330505699923, 212.5844667883370107 ) ) ;
#79849=CARTESIAN_POINT ( 'NONE',  ( 4.042388501175000037, 1517.045004075700035, 209.8579434088520088 ) ) ;
#79863=CARTESIAN_POINT ( 'NONE',  ( -1.708102627415000185, 1517.199196846569976, 215.6864246554469844 ) ) ;
#79868=CARTESIAN_POINT ( 'NONE',  ( 1.710012720495000194, 1517.232977404109988, 201.3945188173769907 ) ) ;
#79872=ADVANCED_FACE ( 'NONE', ( #61400 ), #27219, .F. ) ;
#79874=FACE_OUTER_BOUND ( 'NONE', #10488, .T. ) ;
#79902=CARTESIAN_POINT ( 'NONE',  ( 0.008257837813740559821, 1516.936920898230028, 201.4022722931759972 ) ) ;
#79903=EDGE_CURVE ( 'NONE', #78702, #38027, #95521, .T. ) ;
#79925=ORIENTED_EDGE ( 'NONE', *, *, #39098, .T. ) ;
#79942=CARTESIAN_POINT ( 'NONE',  ( 6.952166382295000169, 1517.213554313520035, 210.8305935944869987 ) ) ;
#79950=CARTESIAN_POINT ( 'NONE',  ( -4.035490750684999739, 1516.630499592039996, 201.4102952541169884 ) ) ;
#79955=CARTESIAN_POINT ( 'NONE',  ( 2.491655725414999800, 1516.977504706749869, 209.8569557413499922 ) ) ;
#79959=EDGE_LOOP ( 'NONE', ( #106685, #63854, #34200, #49564 ) ) ;
#79971=CARTESIAN_POINT ( 'NONE',  ( -1.136547623115000016, 1516.839862955080207, 206.6438706166370025 ) ) ;
#79988=CARTESIAN_POINT ( 'NONE',  ( 1.711311228545000063, 1516.591755933730155, 214.8926661113670207 ) ) ;
#79995=CARTESIAN_POINT ( 'NONE',  ( 4.380123746805410612, 1517.051697240460271, 201.6648244196679798 ) ) ;
#80027=LINE ( 'NONE', #88429, #54990 ) ;
#80041=DIRECTION ( 'NONE',  ( -0.4999999999998399058, 0.7071067811867739472, -0.4999999999998399058 ) ) ;
#80055=CARTESIAN_POINT ( 'NONE',  ( 4.608417506514999928, 1516.691389976299888, 206.6316000176769876 ) ) ;
#80081=ORIENTED_EDGE ( 'NONE', *, *, #11251, .T. ) ;
#80096=CARTESIAN_POINT ( 'NONE',  ( -2.294209667535000108, 1516.603620185149794, 203.3509623682169831 ) ) ;
#80109=CARTESIAN_POINT ( 'NONE',  ( 5.556349309971470696, 1511.457792576160728, 217.8325609232749969 ) ) ;
#80117=CARTESIAN_POINT ( 'NONE',  ( -7.170545816755000246, 1512.974587999889991, 202.0495477424069861 ) ) ;
#80122=DIRECTION ( 'NONE',  ( 0.7071067811865475727, -1.473812113707079404E-16, -0.7071067811865475727 ) ) ;
#80132=EDGE_CURVE ( 'NONE', #13404, #100009, #94182, .T. ) ;
#80133=CARTESIAN_POINT ( 'NONE',  ( 13.59755238133500121, 1512.525301340730039, 224.9104059524669879 ) ) ;
#80142=CARTESIAN_POINT ( 'NONE',  ( 5.770820141135000192, 1516.591755933730155, 207.4105347035570048 ) ) ;
#80199=CARTESIAN_POINT ( 'NONE',  ( 5.690155709095000347, 1515.224164712790071, 200.9877428003970010 ) ) ;
#80201=CARTESIAN_POINT ( 'NONE',  ( 1.121950743945000051, 1517.123342927159911, 204.1084165760470057 ) ) ;
#80224=CARTESIAN_POINT ( 'NONE',  ( -7.322105105754999954, 1516.572193931679976, 211.9951753309869957 ) ) ;
#80232=ADVANCED_FACE ( 'NONE', ( #56190 ), #13605, .F. ) ;
#80233=CARTESIAN_POINT ( 'NONE',  ( -5.924854902405000345, 1514.639648807489948, 216.8926256227769898 ) ) ;
#80234=CARTESIAN_POINT ( 'NONE',  ( 16.09179317404203502, 1514.742486280438925, 194.1160285898321831 ) ) ;
#80246=CARTESIAN_POINT ( 'NONE',  ( 7.321169230994999388, 1516.531533746980131, 207.4131249475269954 ) ) ;
#80256=CARTESIAN_POINT ( 'NONE',  ( 14.92433369415259925, 1512.160613316490071, 196.7006824897309798 ) ) ;
#80266=CARTESIAN_POINT ( 'NONE',  ( 4.036748838804999906, 1516.667393516340098, 216.0582443258770127 ) ) ;
#80270=CARTESIAN_POINT ( 'NONE',  ( 5.384056454772290223, 1511.434805660039956, 217.7741241935190146 ) ) ;
#80273=CARTESIAN_POINT ( 'NONE',  ( 2.299014030735000436, 1516.811292230880099, 211.9858893885470081 ) ) ;
#80290=CARTESIAN_POINT ( 'NONE',  ( -5.010423001364999962, 1516.929569650079884, 205.0907035804270038 ) ) ;
#80300=DIRECTION ( 'NONE',  ( 0.01484500363295476050, 0.5669078173070210003, -0.8236474686073690377 ) ) ;
#80323=CIRCLE ( 'NONE', #14122, 1.000000000039237946 ) ;
#80329=CARTESIAN_POINT ( 'NONE',  ( -14.66019555306499988, 1513.841826332629807, 192.8214360263669960 ) ) ;
#80333=CARTESIAN_POINT ( 'NONE',  ( -3.454119954834999895, 1516.594591938570147, 201.4112355291069889 ) ) ;
#80337=CARTESIAN_POINT ( 'NONE',  ( 7.625190025545000694, 1512.177707669779920, 206.5800331731570054 ) ) ;
#80341=CARTESIAN_POINT ( 'NONE',  ( -17.05938549526129577, 1517.051704405600049, 195.1949804090679947 ) ) ;
#80347=CARTESIAN_POINT ( 'NONE',  ( -8.558300775104999758, 1511.397837225850026, 214.2288200170269761 ) ) ;
#80354=( LENGTH_UNIT ( ) NAMED_UNIT ( * ) SI_UNIT ( .MILLI., .METRE. ) );
#80369=CARTESIAN_POINT ( 'NONE',  ( 2.874588922665000545, 1516.606339319019980, 215.6687976528169770 ) ) ;
#80370=CARTESIAN_POINT ( 'NONE',  ( 3.432975284724999909, 1511.645462744430006, 217.1388420280169953 ) ) ;
#80376=CARTESIAN_POINT ( 'NONE',  ( 0.7365611785030020675, 1517.066898074209803, 204.4979538714769944 ) ) ;
#80389=CARTESIAN_POINT ( 'NONE',  ( -7.710285875814999912, 1516.582197289609894, 212.3822242253069987 ) ) ;
#80396=CARTESIAN_POINT ( 'NONE',  ( 6.562094069294999166, 1517.122674412569950, 209.8604508749069737 ) ) ;
#80407=CYLINDRICAL_SURFACE ( 'NONE', #83099, 2.000000000000007550 ) ;
#80411=CARTESIAN_POINT ( 'NONE',  ( -4.613762395014999740, 1516.939574742129935, 214.9064842900469898 ) ) ;
#80415=ORIENTED_EDGE ( 'NONE', *, *, #27617, .F. ) ;
#80416=CARTESIAN_POINT ( 'NONE',  ( 0.7391219670640019057, 1517.130100026000036, 202.1721425974470208 ) ) ;
#80422=CARTESIAN_POINT ( 'NONE',  ( 8.639302646193000257, 1511.681069547209972, 203.0735539262880138 ) ) ;
#80439=DIRECTION ( 'NONE',  ( 1.000000000000000000, 0.000000000000000000, 0.000000000000000000 ) ) ;
#80451=CARTESIAN_POINT ( 'NONE',  ( -0.2489082263676290208, 1516.862251239930174, 201.4042270512659911 ) ) ;
#80498=CARTESIAN_POINT ( 'NONE',  ( -0.7352271553329990939, 1516.963431999339946, 210.8369554172870153 ) ) ;
#80502=VECTOR ( 'NONE', #20559, 1000.000000000000000 ) ;
#80507=CARTESIAN_POINT ( 'NONE',  ( -7.329925260535000042, 1516.833976295079992, 201.4049670291269933 ) ) ;
#80528=CARTESIAN_POINT ( 'NONE',  ( -0.7576635715699989726, 1516.855632454399938, 206.2537338009369989 ) ) ;
#80545=CARTESIAN_POINT ( 'NONE',  ( 2.292940169014999974, 1516.565291103010168, 215.6678853655270132 ) ) ;
#80582=ORIENTED_EDGE ( 'NONE', *, *, #97548, .F. ) ;
#80588=CARTESIAN_POINT ( 'NONE',  ( -7.613267233414999779, 1512.877204813269827, 211.3708094598169964 ) ) ;
#80596=LINE ( 'NONE', #73859, #74776 ) ;
#80601=CARTESIAN_POINT ( 'NONE',  ( -7.096077632602200147, 1508.610125823030103, 215.7701981269059957 ) ) ;
#80614=CARTESIAN_POINT ( 'NONE',  ( -2.882326017515000061, 1516.969638403840008, 207.4201161117570109 ) ) ;
#80619=CARTESIAN_POINT ( 'NONE',  ( 10.96015508933500016, 1516.551704408390151, 225.0317485278669949 ) ) ;
#80635=CARTESIAN_POINT ( 'NONE',  ( 12.43458519346858715, 1513.190421807558096, 225.8467871284239834 ) ) ;
#80652=CARTESIAN_POINT ( 'NONE',  ( 2.867803626105000170, 1516.994127245590107, 204.4971090729170271 ) ) ;
#80666=CARTESIAN_POINT ( 'NONE',  ( 5.716900179066289667, 1511.491070485845285, 217.8701534166750946 ) ) ;
#80675=CARTESIAN_POINT ( 'NONE',  ( -7.469619929815000781, 1513.342361861110248, 201.3714591891869929 ) ) ;
#80676=ORIENTED_EDGE ( 'NONE', *, *, #34468, .F. ) ;
#80689=CARTESIAN_POINT ( 'NONE',  ( 13.19864377693500046, 1513.023086264660151, 225.9744572943669993 ) ) ;
#80698=CARTESIAN_POINT ( 'NONE',  ( 3.251394362135000105, 1516.757508073510053, 207.4061414411269766 ) ) ;
#80712=LINE ( 'NONE', #37604, #85500 ) ;
#80717=CARTESIAN_POINT ( 'NONE',  ( 6.123056445345035570, 1510.784366248568858, 216.5990792139033942 ) ) ;
#80755=CARTESIAN_POINT ( 'NONE',  ( -6.560742263465000335, 1517.028034847769959, 205.0881926677770082 ) ) ;
#80769=DIRECTION ( 'NONE',  ( -0.6742693640212139572, -4.521919481779818477E-17, -0.7384854939282339270 ) ) ;
#80786=CARTESIAN_POINT ( 'NONE',  ( 16.26362608049849712, 1514.552098279665415, 194.3450158896016831 ) ) ;
#80789=CIRCLE ( 'NONE', #68328, 7.500000000000000000 ) ;
#80794=( BOUNDED_CURVE ( )  B_SPLINE_CURVE ( 3, ( #82665, #108413, #5956, #66980 ),
 .UNSPECIFIED., .F., .F. ) 
 B_SPLINE_CURVE_WITH_KNOTS ( ( 4, 4 ),
 ( 0.9002477009694567212, 1.144704973640544798 ),
 .UNSPECIFIED. ) 
 CURVE ( )  GEOMETRIC_REPRESENTATION_ITEM ( )  RATIONAL_B_SPLINE_CURVE ( ( 1.000000000000000000, 0.9950262503666102987, 0.9950262503666102987, 1.000000000000000000 ) ) 
 REPRESENTATION_ITEM ( '' )  );
#80798=CARTESIAN_POINT ( 'NONE',  ( -7.725990199955000470, 1517.181921232829836, 206.6366402828969910 ) ) ;
#80807=CARTESIAN_POINT ( 'NONE',  ( 7.512750207965000371, 1509.038615934239942, 203.6084103740869864 ) ) ;
#80809=CARTESIAN_POINT ( 'NONE',  ( -5.730039698873020448, 1510.523965798400013, 201.5701372575169898 ) ) ;
#80815=CARTESIAN_POINT ( 'NONE',  ( -7.715625241105000143, 1516.786099423779888, 215.6766101314970001 ) ) ;
#80819=CARTESIAN_POINT ( 'NONE',  ( -5.771797464315000070, 1516.647618671360078, 211.9976960644470125 ) ) ;
#80827=DIRECTION ( 'NONE',  ( 0.9980967576408298347, 0.06164622075854649108, 0.001614265483442069724 ) ) ;
#80835=CARTESIAN_POINT ( 'NONE',  ( -2.877744984375000037, 1516.723920667490120, 204.5127816287269980 ) ) ;
#80866=CARTESIAN_POINT ( 'NONE',  ( 8.152186767047583160, 1511.505229895813500, 205.2575009507046957 ) ) ;
#80871=VERTEX_POINT ( 'NONE', #78369 ) ;
#80877=CARTESIAN_POINT ( 'NONE',  ( -11.95959066036500040, 1513.007288725360013, 192.5106861886669947 ) ) ;
#80881=CARTESIAN_POINT ( 'NONE',  ( 3.453544825624999870, 1517.106845464700200, 201.7850012896870169 ) ) ;
#80885=CARTESIAN_POINT ( 'NONE',  ( 7.629870545114999736, 1512.332007210709889, 206.5727344848370137 ) ) ;
#80887=EDGE_CURVE ( 'NONE', #88321, #72815, #100414, .T. ) ;
#80895=CARTESIAN_POINT ( 'NONE',  ( -7.563688229914999894, 1510.983859056260144, 212.0526840097969909 ) ) ;
#80907=DIRECTION ( 'NONE',  ( -0.4999999999998399614, -0.7071067811867740582, -0.4999999999998399614 ) ) ;
#80908=ORIENTED_EDGE ( 'NONE', *, *, #3502, .F. ) ;
#80916=CARTESIAN_POINT ( 'NONE',  ( 1.711311228545000063, 1516.591755933730155, 214.8926661113670207 ) ) ;
#80923=CARTESIAN_POINT ( 'NONE',  ( -7.335901033725000353, 1517.068717944079935, 205.0869373723870126 ) ) ;
#80930=CARTESIAN_POINT ( 'NONE',  ( -17.17760814124009983, 1517.051704413129983, 195.4929600000709797 ) ) ;
#80936=CARTESIAN_POINT ( 'NONE',  ( -0.7355686809059980291, 1517.012231669750008, 212.3888856620870058 ) ) ;
#80941=CARTESIAN_POINT ( 'NONE',  ( -7.712670236151770276, 1516.673252337400072, 210.0631823355520282 ) ) ;
#80942=CARTESIAN_POINT ( 'NONE',  ( 7.339107202615000602, 1517.203017563489766, 210.2473558205170150 ) ) ;
#80948=B_SPLINE_CURVE_WITH_KNOTS ( 'NONE', 3,
 ( #90424, #46811, #14269, #49009, #89883, #74216, #38917, #13702, #48460, #57419, #63619, #97735, #47890, #21006, #81467, #5330, #55209, #31627, #72550, #73661, #82026, #65260, #22096, #6440, #65805, #73098, #98836, #99371, #99925, #107237, #64720, #83145, #39490, #82598, #29971, #91545, #107793, #89338, #22643, #23219, #80941, #31077, #40585, #4239, #5888, #30528, #38374, #108345, #74757, #21557, #29419, #64163, #12634, #106680, #98281, #13153, #47338, #49558, #68024, #85897, #57957, #15909, #9203, #24860 ),
 .UNSPECIFIED., .F., .F.,
 ( 4, 3, 3, 3, 3, 3, 3, 3, 3, 3, 3, 3, 3, 3, 3, 3, 3, 3, 3, 3, 3, 4 ),
 ( -14.97205243065559976, -14.82652090134419964, -14.54016986210000084, -14.44422471178040013, -14.18616264305039998, -13.96389174838669867, -13.75628582469069983, -13.55954966579430021, -13.48778920245429980, -13.41168693589320071, -13.29682063962729899, -13.03955858623080033, -12.77367974343709989, -12.48589049144669971, -12.17406903241579919, -11.81735513509999969, -11.73764735024779959, -11.37242316392340058, -11.02427058926000036, -10.95328185380470032, -10.66065659679330047, -10.38572052090729869 ),
 .UNSPECIFIED. ) ;
#80953=CARTESIAN_POINT ( 'NONE',  ( 7.594039249315000184, 1512.142919181319940, 206.8921143228970152 ) ) ;
#80956=CARTESIAN_POINT ( 'NONE',  ( -1.709384611084999950, 1517.224900789629828, 216.4615953054470197 ) ) ;
#80960=CARTESIAN_POINT ( 'NONE',  ( -3.260378293205000055, 1516.582197289609894, 201.4115600944169842 ) ) ;
#80964=EDGE_CURVE ( 'NONE', #5353, #44905, #99004, .T. ) ;
#80990=EDGE_CURVE ( 'NONE', #66010, #89621, #102023, .T. ) ;
#80994=CARTESIAN_POINT ( 'NONE',  ( -0.08855571868401390656, 1516.909122020869972, 201.4030000720750024 ) ) ;
#80997=CARTESIAN_POINT ( 'NONE',  ( 14.75568479846049819, 1513.870294662269998, 224.0700459103859714 ) ) ;
#81024=CARTESIAN_POINT ( 'NONE',  ( 14.72577158086200022, 1514.214451999800076, 194.1036973123569851 ) ) ;
#81035=CARTESIAN_POINT ( 'NONE',  ( 2.300729626665000360, 1516.923170579120097, 210.8225527465970117 ) ) ;
#81041=CARTESIAN_POINT ( 'NONE',  ( 2.485205649205000089, 1517.181921232829836, 201.3958557702769951 ) ) ;
#81056=CARTESIAN_POINT ( 'NONE',  ( -7.710967015764999211, 1516.608208975040043, 210.2506035313070072 ) ) ;
#81061=CARTESIAN_POINT ( 'NONE',  ( 7.559673304084999934, 1510.830536680500245, 205.9482437802269885 ) ) ;
#81062=CARTESIAN_POINT ( 'NONE',  ( -4.043366258305000294, 1516.951766529250108, 206.2549880390970145 ) ) ;
#81079=CARTESIAN_POINT ( 'NONE',  ( 2.875850094215000041, 1516.647618671360078, 214.8936433964170192 ) ) ;
#81081=CARTESIAN_POINT ( 'NONE',  ( 7.708876326848260518, 1516.528370242520168, 207.0834033919979902 ) ) ;
#81111=CARTESIAN_POINT ( 'NONE',  ( -13.92686555291570194, 1517.051704405520013, 226.1812314194930025 ) ) ;
#81147=CYLINDRICAL_SURFACE ( 'NONE', #3667, 1.000000000000070166 ) ;
#81151=CARTESIAN_POINT ( 'NONE',  ( -0.7559395363919990674, 1516.972341476009888, 207.9998125401569951 ) ) ;
#81170=CARTESIAN_POINT ( 'NONE',  ( 10.96015508933500016, 1512.830284628050094, 225.0317485278669949 ) ) ;
#81177=CARTESIAN_POINT ( 'NONE',  ( 4.678149145594550085, 1508.611352722540005, 205.6342600828810134 ) ) ;
#81185=CARTESIAN_POINT ( 'NONE',  ( -2.877113108595000135, 1516.697242742309982, 204.1252037719370094 ) ) ;
#81186=ORIENTED_EDGE ( 'NONE', *, *, #45621, .T. ) ;
#81189=ORIENTED_EDGE ( 'NONE', *, *, #60296, .F. ) ;
#81194=CARTESIAN_POINT ( 'NONE',  ( -13.13649031037390102, 1512.464953430890091, 193.8649562899759928 ) ) ;
#81206=CARTESIAN_POINT ( 'NONE',  ( -6.013894009214999947, 1511.644799026709961, 201.1705823216470037 ) ) ;
#81222=CARTESIAN_POINT ( 'NONE',  ( 13.50445032983499871, 1512.655881406860090, 224.4988687930670039 ) ) ;
#81228=CARTESIAN_POINT ( 'NONE',  ( 1.118104729594999958, 1516.965971551240045, 206.8221779662269739 ) ) ;
#81282=CARTESIAN_POINT ( 'NONE',  ( -2.878693287274999957, 1516.766397346390022, 205.0941487061870134 ) ) ;
#81298=CARTESIAN_POINT ( 'NONE',  ( -1.119592219845000125, 1516.958737650239982, 210.2577447559170025 ) ) ;
#81311=CARTESIAN_POINT ( 'NONE',  ( -6.834484321545000185, 1513.760531203570054, 216.6429190012370043 ) ) ;
#81323=CARTESIAN_POINT ( 'NONE',  ( 4.026614479655000522, 1516.699825673279975, 207.4075116849170115 ) ) ;
#81334=CARTESIAN_POINT ( 'NONE',  ( -5.972112790866080267, 1511.562335007999991, 200.3290730311999823 ) ) ;
#81341=CARTESIAN_POINT ( 'NONE',  ( -4.615017365965000451, 1516.987478262539980, 215.6816440265270103 ) ) ;
#81345=CARTESIAN_POINT ( 'NONE',  ( -6.547881413045000265, 1516.647534046129977, 212.5778533554070293 ) ) ;
#81363=CARTESIAN_POINT ( 'NONE',  ( 7.711550677984999602, 1516.630499592039996, 205.0863552195469879 ) ) ;
#81386=CARTESIAN_POINT ( 'NONE',  ( 8.609269427741782721, 1511.418041552835120, 203.8636807336108063 ) ) ;
#81397=CARTESIAN_POINT ( 'NONE',  ( -12.49293100206499929, 1511.939906524110256, 193.6511072290670086 ) ) ;
#81400=CARTESIAN_POINT ( 'NONE',  ( -6.943602691585000208, 1516.858069504249897, 202.1807456543569685 ) ) ;
#81411=CARTESIAN_POINT ( 'NONE',  ( -3.487592467065000257, 1509.038615934169911, 213.6090957241370063 ) ) ;
#81425=FACE_OUTER_BOUND ( 'NONE', #94290, .T. ) ;
#81435=CARTESIAN_POINT ( 'NONE',  ( -0.7376675409259989546, 1517.104497701820037, 214.9086937099069985 ) ) ;
#81446=CARTESIAN_POINT ( 'NONE',  ( 3.448206878685000198, 1516.904492006980036, 205.0794281543969646 ) ) ;
#81461=CARTESIAN_POINT ( 'NONE',  ( -6.935133418554999096, 1516.613881697390070, 212.3834819030570031 ) ) ;
#81467=CARTESIAN_POINT ( 'NONE',  ( -7.708852918845599866, 1516.527474870850256, 211.2226130665349899 ) ) ;
#81468=CARTESIAN_POINT ( 'NONE',  ( -0.7374509209069979310, 1516.978425811520083, 210.2554991112269818 ) ) ;
#81480=CARTESIAN_POINT ( 'NONE',  ( 7.563688191785000292, 1510.983859056260144, 206.1910078925270113 ) ) ;
#81484=CARTESIAN_POINT ( 'NONE',  ( -2.290886304614999869, 1517.184383877180153, 216.4605998004670084 ) ) ;
#81489=CARTESIAN_POINT ( 'NONE',  ( -1.708092304294999808, 1516.523379810429788, 201.4131002843170108 ) ) ;
#81492=CARTESIAN_POINT ( 'NONE',  ( -15.87603345926501675, 1512.359593911809952, 220.1461273412669755 ) ) ;
#81523=CARTESIAN_POINT ( 'NONE',  ( -0.9413364034040100359, 1516.673252337410077, 201.4091757340799802 ) ) ;
#81527=CARTESIAN_POINT ( 'NONE',  ( 12.42116344234460001, 1512.160613316490071, 224.0461796643650132 ) ) ;
#81529=EDGE_LOOP ( 'NONE', ( #6903, #3106, #46429, #64970 ) ) ;
#81565=ORIENTED_EDGE ( 'NONE', *, *, #102982, .T. ) ;
#81569=CARTESIAN_POINT ( 'NONE',  ( 7.727327114725000001, 1517.232977404109988, 210.8318586907270173 ) ) ;
#81572=CARTESIAN_POINT ( 'NONE',  ( 4.042729802795000715, 1516.919782530640077, 212.3762473738369749 ) ) ;
#81580=CARTESIAN_POINT ( 'NONE',  ( 0.7396922377450010355, 1517.135701590510052, 201.7845486201169933 ) ) ;
#81594=CARTESIAN_POINT ( 'NONE',  ( -0.7352271553329990939, 1516.963431999339946, 210.8369554172870153 ) ) ;
#81600=CARTESIAN_POINT ( 'NONE',  ( 8.016996057795001462, 1511.645462744430006, 205.6888706473769730 ) ) ;
#81602=CARTESIAN_POINT ( 'NONE',  ( 4.608417506514999928, 1516.691389976299888, 206.6316000176769876 ) ) ;
#81618=LINE ( 'NONE', #5477, #31638 ) ;
#81619=CARTESIAN_POINT ( 'NONE',  ( 3.457266605394999637, 1516.691414181030041, 214.8945738789770132 ) ) ;
#81624=EDGE_CURVE ( 'NONE', #104774, #5353, #80596, .T. ) ;
#81637=ORIENTED_EDGE ( 'NONE', *, *, #20758, .F. ) ;
#81683=CARTESIAN_POINT ( 'NONE',  ( -7.482857926667088933, 1511.023286695659863, 215.2724589492860048 ) ) ;
#81689=CARTESIAN_POINT ( 'NONE',  ( 7.323390407215000231, 1516.613712827999962, 207.9924597298270044 ) ) ;
#81716=EDGE_CURVE ( 'NONE', #53542, #110638, #14057, .T. ) ;
#81718=CARTESIAN_POINT ( 'NONE',  ( 3.861663294462490015, 1508.610718243669908, 204.4420517555579977 ) ) ;
#81720=LINE ( 'NONE', #39172, #29488 ) ;
#81726=CARTESIAN_POINT ( 'NONE',  ( -3.487585001777260274, 1508.551704408610021, 204.2892321445339689 ) ) ;
#81728=CARTESIAN_POINT ( 'NONE',  ( -4.621267922064999922, 1516.830644417779922, 204.1223895416970038 ) ) ;
#81737=CARTESIAN_POINT ( 'NONE',  ( -14.69525445759580151, 1513.799047785590119, 194.1342753316129688 ) ) ;
#81760=( BOUNDED_CURVE ( )  B_SPLINE_CURVE ( 3, ( #72847, #106981, #56041, #30269 ),
 .UNSPECIFIED., .F., .T. ) 
 B_SPLINE_CURVE_WITH_KNOTS ( ( 4, 4 ),
 ( 1.570952385993269473, 3.141745504670674816 ),
 .UNSPECIFIED. ) 
 CURVE ( )  GEOMETRIC_REPRESENTATION_ITEM ( )  RATIONAL_B_SPLINE_CURVE ( ( 1.000000000000000000, 0.8047386102843028244, 0.8047386102843028244, 1.000000000000000000 ) ) 
 REPRESENTATION_ITEM ( '' )  );
#81767=CARTESIAN_POINT ( 'NONE',  ( 11.65415823093499981, 1512.679339245399888, 225.6053821474669974 ) ) ;
#81787=DIRECTION ( 'NONE',  ( 0.7071067811865490160, 0.000000000000000000, -0.7071067811865460184 ) ) ;
#81794=B_SPLINE_CURVE_WITH_KNOTS ( 'NONE', 3,
 ( #36439, #44313, #28596, #35343, #54379, #12331 ),
 .UNSPECIFIED., .F., .F.,
 ( 4, 2, 4 ),
 ( 0.000000000000000000, 0.5000000000000000000, 1.000000000000000000 ),
 .UNSPECIFIED. ) ;
#81816=CARTESIAN_POINT ( 'NONE',  ( 5.649719750514999639, 1514.216922324319739, 200.4731542066570000 ) ) ;
#81824=CARTESIAN_POINT ( 'NONE',  ( -3.605950197753253761, 1511.586636682142625, 201.0506624174682315 ) ) ;
#81832=CARTESIAN_POINT ( 'NONE',  ( -1.134358008724999811, 1516.744381837270112, 205.0932347109869909 ) ) ;
#81847=CARTESIAN_POINT ( 'NONE',  ( -4.031168805994999715, 1516.805675336850072, 209.8787446699039947 ) ) ;
#81861=ORIENTED_EDGE ( 'NONE', *, *, #48019, .T. ) ;
#81863=CARTESIAN_POINT ( 'NONE',  ( -6.059489674125000391, 1514.830240247470101, 217.0841925463570021 ) ) ;
#81864=CARTESIAN_POINT ( 'NONE',  ( 16.78391007505477361, 1513.564960623365778, 195.8729266718472672 ) ) ;
#81878=CARTESIAN_POINT ( 'NONE',  ( -6.951517170504999399, 1517.194816588360027, 207.9969518818670053 ) ) ;
#81888=CARTESIAN_POINT ( 'NONE',  ( -5.912728008667049728, 1510.598356033839991, 201.5879984038760142 ) ) ;
#81890=CARTESIAN_POINT ( 'NONE',  ( -5.929777071639043662, 1510.642476712295547, 201.6026015433274381 ) ) ;
#81895=CARTESIAN_POINT ( 'NONE',  ( -2.484577695354999616, 1517.170512887980067, 216.4602579296269766 ) ) ;
#81899=CARTESIAN_POINT ( 'NONE',  ( 7.336844642415000450, 1517.106845464700200, 212.5753907958570039 ) ) ;
#81919=CARTESIAN_POINT ( 'NONE',  ( -1.713317447804999949, 1516.660388280709867, 204.5138242629670060 ) ) ;
#81945=CARTESIAN_POINT ( 'NONE',  ( -4.075310406729379942, 1517.051704406860154, 216.1877156734769869 ) ) ;
#81948=CARTESIAN_POINT ( 'NONE',  ( 8.431940979592114971, 1511.395336166478046, 204.3955032846177460 ) ) ;
#81957=CARTESIAN_POINT ( 'NONE',  ( -10.96771875526499862, 1512.594959757389915, 193.2043797466670014 ) ) ;
#81960=CARTESIAN_POINT ( 'NONE',  ( 5.002593359325000044, 1516.960844870249957, 202.5626772953570196 ) ) ;
#81963=CARTESIAN_POINT ( 'NONE',  ( 16.22329229643499815, 1513.248517198770060, 194.7967040231669955 ) ) ;
#81968=VERTEX_POINT ( 'NONE', #90503 ) ;
#81985=CARTESIAN_POINT ( 'NONE',  ( 7.449529084515000399, 1511.198876514819858, 202.8590003749670245 ) ) ;
#81996=CARTESIAN_POINT ( 'NONE',  ( -5.002593397454999646, 1516.960844870249957, 215.6810146069769871 ) ) ;
#82006=CARTESIAN_POINT ( 'NONE',  ( 5.772727908745000747, 1516.691414181030041, 205.6645793267070133 ) ) ;
#82008=CARTESIAN_POINT ( 'NONE',  ( -4.623892098755000291, 1517.066898074209803, 208.3852847535989952 ) ) ;
#82012=CARTESIAN_POINT ( 'NONE',  ( 7.101217468594999360, 1512.693483295329997, 217.4300948872370043 ) ) ;
#82015=CARTESIAN_POINT ( 'NONE',  ( 5.513435558210308507, 1508.551704408385376, 216.2892291545065291 ) ) ;
#82021=CARTESIAN_POINT ( 'NONE',  ( -6.547556969464999987, 1516.633288330999903, 212.3841106205370011 ) ) ;
#82026=CARTESIAN_POINT ( 'NONE',  ( -7.709135228525060057, 1516.538255842549916, 210.9323641728119867 ) ) ;
#82027=CARTESIAN_POINT ( 'NONE',  ( -2.477975353594999763, 1516.839862955080207, 210.2583935552169976 ) ) ;
#82041=CARTESIAN_POINT ( 'NONE',  ( -3.259101837015000225, 1517.102359858469754, 216.0714209178769920 ) ) ;
#82046=CARTESIAN_POINT ( 'NONE',  ( -7.329925260535000042, 1516.833976295079992, 201.4049670291269933 ) ) ;
#82061=LINE ( 'NONE', #65295, #89461 ) ;
#82067=DIRECTION ( 'NONE',  ( 0.9996573249755689172, 0.02617694830742899742, -1.602875797806941134E-18 ) ) ;
#82079=AXIS2_PLACEMENT_3D ( 'NONE', #9647, #43822, #3495 ) ;
#82083=CARTESIAN_POINT ( 'NONE',  ( 0.1763907685423009852, 1516.984411380839902, 201.4010288749069844 ) ) ;
#82088=CARTESIAN_POINT ( 'NONE',  ( 14.81380078118680110, 1513.941944658630064, 224.0275431902680054 ) ) ;
#82093=CARTESIAN_POINT ( 'NONE',  ( 5.421019186268996037, 1516.848040087860227, 203.8236974790748945 ) ) ;
#82129=CARTESIAN_POINT ( 'NONE',  ( 1.136814033864999907, 1516.854133554269993, 211.4058994415870245 ) ) ;
#82131=CARTESIAN_POINT ( 'NONE',  ( 6.560742225334999844, 1517.028034847769959, 213.1554992345569701 ) ) ;
#82139=CARTESIAN_POINT ( 'NONE',  ( -4.036119682645000317, 1516.647924054489977, 201.7978713257969900 ) ) ;
#82156=CARTESIAN_POINT ( 'NONE',  ( 5.013429356055000063, 1517.123342927159911, 210.2437967141769946 ) ) ;
#82161=CARTESIAN_POINT ( 'NONE',  ( 8.245978508674999929, 1511.399604276809896, 204.0113757433670116 ) ) ;
#82162=CARTESIAN_POINT ( 'NONE',  ( 5.772978278544999675, 1516.659138130710289, 207.9900491214870044 ) ) ;
#82173=CARTESIAN_POINT ( 'NONE',  ( 6.372167600494999640, 1511.069621805459974, 216.5183910133270047 ) ) ;
#82181=CARTESIAN_POINT ( 'NONE',  ( 1.708720984574999768, 1516.531533746980131, 216.4430152012269843 ) ) ;
#82183=CARTESIAN_POINT ( 'NONE',  ( 7.717523752519699798, 1516.858602105719910, 208.8606392115019901 ) ) ;
#82184=LINE ( 'NONE', #30120, #62392 ) ;
#82196=ORIENTED_EDGE ( 'NONE', *, *, #63454, .T. ) ;
#82197=CARTESIAN_POINT ( 'NONE',  ( -5.513435911474870110, 1508.551704408389924, 202.1089243664339961 ) ) ;
#82218=EDGE_CURVE ( 'NONE', #23166, #51438, #37548, .T. ) ;
#82246=ADVANCED_FACE ( 'NONE', ( #79242 ), #40143, .T. ) ;
#82254=CARTESIAN_POINT ( 'NONE',  ( -8.642118163667179331, 1511.774552108250191, 215.2838205174969630 ) ) ;
#82260=CARTESIAN_POINT ( 'NONE',  ( 2.865636809105000182, 1516.815173273089840, 207.9858416580370033 ) ) ;
#82269=ORIENTED_EDGE ( 'NONE', *, *, #17844, .F. ) ;
#82290=CARTESIAN_POINT ( 'NONE',  ( 3.487584386345879750, 1508.551704408389924, 204.1347675156980017 ) ) ;
#82300=CARTESIAN_POINT ( 'NONE',  ( 2.478306819944999795, 1516.938330505699923, 205.6592251139969960 ) ) ;
#82309=CARTESIAN_POINT ( 'NONE',  ( -13.03156812829710098, 1512.406412988020065, 193.8931400537850038 ) ) ;
#82315=CYLINDRICAL_SURFACE ( 'NONE', #23134, 0.9999999999999985567 ) ;
#82398=CARTESIAN_POINT ( 'NONE',  ( -3.849878380766676766, 1511.509050022477140, 200.9742446617588314 ) ) ;
#82406=CARTESIAN_POINT ( 'NONE',  ( 4.609996581545000360, 1516.769879638719885, 205.6626893540170329 ) ) ;
#82422=CARTESIAN_POINT ( 'NONE',  ( -6.935801299664999142, 1516.621991115350056, 210.2518484644969874 ) ) ;
#82434=CARTESIAN_POINT ( 'NONE',  ( -6.648850802594999720, 1513.600111798349872, 216.5887361369370012 ) ) ;
#82435=CARTESIAN_POINT ( 'NONE',  ( 16.61266722949974195, 1514.059034352515937, 195.0269839839985480 ) ) ;
#82447=CARTESIAN_POINT ( 'NONE',  ( 2.872836622524999939, 1517.158319634930194, 201.3964737998670103 ) ) ;
#82448=CARTESIAN_POINT ( 'NONE',  ( 1.122033391945000069, 1516.972341476009888, 208.3659064338399673 ) ) ;
#82462=FACE_OUTER_BOUND ( 'NONE', #54066, .T. ) ;
#82466=CARTESIAN_POINT ( 'NONE',  ( -4.616899872884999922, 1517.050041317280147, 216.8443827349270236 ) ) ;
#82471=CARTESIAN_POINT ( 'NONE',  ( -2.865911554774999814, 1516.906233342200039, 212.5838411289170153 ) ) ;
#82474=CARTESIAN_POINT ( 'NONE',  ( 3.801724372608250135, 1509.034524880150002, 213.6092044083339943 ) ) ;
#82488=CARTESIAN_POINT ( 'NONE',  ( -1.134358008724999811, 1516.744381837270112, 205.0932347109869909 ) ) ;
#82490=( GEOMETRIC_REPRESENTATION_CONTEXT ( 3 ) GLOBAL_UNCERTAINTY_ASSIGNED_CONTEXT ( ( #102831 ) ) GLOBAL_UNIT_ASSIGNED_CONTEXT ( ( #80354, #29928, #98241 ) ) REPRESENTATION_CONTEXT ( 'NONE', 'WORKASPACE' ) );
#82527=CARTESIAN_POINT ( 'NONE',  ( -7.396545081224999763, 1511.069621805459974, 215.4940135707269917 ) ) ;
#82536=CARTESIAN_POINT ( 'NONE',  ( 7.328676169885000036, 1516.833844030519913, 202.1788723028969912 ) ) ;
#82539=CARTESIAN_POINT ( 'NONE',  ( 16.10875976033500123, 1511.961073825299991, 196.9868955663669965 ) ) ;
#82553=CARTESIAN_POINT ( 'NONE',  ( -7.893411120225001021, 1512.020737142380085, 212.1186310024369845 ) ) ;
#82564=CARTESIAN_POINT ( 'NONE',  ( 8.232567722344999339, 1512.371207877099778, 202.4629285007669921 ) ) ;
#82565=ORIENTED_EDGE ( 'NONE', *, *, #85786, .F. ) ;
#82573=CARTESIAN_POINT ( 'NONE',  ( -5.003220765204999587, 1516.983995446890049, 216.0685944891870065 ) ) ;
#82580=CARTESIAN_POINT ( 'NONE',  ( 1.119717716265000051, 1517.038650117239968, 205.6590103047369951 ) ) ;
#82582=CARTESIAN_POINT ( 'NONE',  ( -2.868112169295000236, 1516.855632454399938, 209.8795095036720113 ) ) ;
#82588=CARTESIAN_POINT ( 'NONE',  ( 5.513435558014999849, 1508.551704408389924, 216.1347675157070114 ) ) ;
#82594=CARTESIAN_POINT ( 'NONE',  ( -1.120543735785000106, 1517.073005577650065, 213.1661658574570026 ) ) ;
#82598=CARTESIAN_POINT ( 'NONE',  ( -7.710327657623590625, 1516.583792872650065, 210.5203955415310020 ) ) ;
#82599=CARTESIAN_POINT ( 'NONE',  ( 2.299667965875000331, 1516.965971551240045, 210.2399506998270056 ) ) ;
#82613=CARTESIAN_POINT ( 'NONE',  ( -2.872208748294999836, 1517.145312756229941, 216.4596396827270155 ) ) ;
#82618=CARTESIAN_POINT ( 'NONE',  ( 7.328676169885000036, 1516.833844030519913, 202.1788723028969912 ) ) ;
#82619=FACE_OUTER_BOUND ( 'NONE', #42993, .T. ) ;
#82622=CARTESIAN_POINT ( 'NONE',  ( 7.512705394560745376, 1509.036904579576458, 214.8970114893355117 ) ) ;
#82644=CARTESIAN_POINT ( 'NONE',  ( -8.311290134334250013, 1511.035127054690065, 215.8965699024140008 ) ) ;
#82645=CARTESIAN_POINT ( 'NONE',  ( -4.987078460856490203, 1508.551704408389924, 212.6094383991630252 ) ) ;
#82654=CARTESIAN_POINT ( 'NONE',  ( 14.15402810059180005, 1513.231391185909843, 224.3576605340919912 ) ) ;
#82665=CARTESIAN_POINT ( 'NONE',  ( 13.62888593203049936, 1517.051704413129983, 191.9442378289920157 ) ) ;
#82673=ORIENTED_EDGE ( 'NONE', *, *, #85806, .T. ) ;
#82674=ORIENTED_EDGE ( 'NONE', *, *, #82218, .T. ) ;
#82692=CARTESIAN_POINT ( 'NONE',  ( -4.608417544644999531, 1516.691389976299888, 211.6120918846570191 ) ) ;
#82695=CARTESIAN_POINT ( 'NONE',  ( -6.935133418554999096, 1516.613881697390070, 212.3834819030570031 ) ) ;
#82702=CARTESIAN_POINT ( 'NONE',  ( -7.718763544034999313, 1516.905946377369901, 202.1794916586869988 ) ) ;
#82716=CARTESIAN_POINT ( 'NONE',  ( -2.476450702264999748, 1516.843453247299749, 211.4215022863270121 ) ) ;
#82721=CARTESIAN_POINT ( 'NONE',  ( 7.550503323924999677, 1510.480349266450048, 203.5706572581269995 ) ) ;
#82722=CARTESIAN_POINT ( 'NONE',  ( 4.608021669135000664, 1516.660388280709867, 207.4085285224269910 ) ) ;
#82739=CARTESIAN_POINT ( 'NONE',  ( -1.125509888415000104, 1517.203017563489766, 216.4609531728469847 ) ) ;
#82745=( BOUNDED_CURVE ( )  B_SPLINE_CURVE ( 3, ( #102113, #25392, #6417, #23749 ),
 .UNSPECIFIED., .F., .F. ) 
 B_SPLINE_CURVE_WITH_KNOTS ( ( 4, 4 ),
 ( 1.282549416709988011, 2.438195290911524982 ),
 .UNSPECIFIED. ) 
 CURVE ( )  GEOMETRIC_REPRESENTATION_ITEM ( )  RATIONAL_B_SPLINE_CURVE ( ( 1.000000000000000000, 0.8917691662025382104, 0.8917691662025382104, 1.000000000000000000 ) ) 
 REPRESENTATION_ITEM ( '' )  );
#82768=CARTESIAN_POINT ( 'NONE',  ( -5.496430559424999807, 1510.805212328559946, 201.5628357695169939 ) ) ;
#82807=CARTESIAN_POINT ( 'NONE',  ( -1.717139122245000094, 1516.949031626070109, 208.0040058453670042 ) ) ;
#82819=CARTESIAN_POINT ( 'NONE',  ( 7.487063056100070391, 1517.051702153270071, 209.5621714086410066 ) ) ;
#82832=CARTESIAN_POINT ( 'NONE',  ( 4.679794195664990220, 1508.610718263850003, 205.2601949082799990 ) ) ;
#82842=CARTESIAN_POINT ( 'NONE',  ( -3.459156616214999591, 1516.769879638719885, 204.5118493505569859 ) ) ;
#82843=ORIENTED_EDGE ( 'NONE', *, *, #96197, .T. ) ;
#82846=CARTESIAN_POINT ( 'NONE',  ( 15.00007757067209901, 1512.191474810040063, 196.5897778920760288 ) ) ;
#82865=ORIENTED_EDGE ( 'NONE', *, *, #37742, .F. ) ;
#82942=CARTESIAN_POINT ( 'NONE',  ( 0.7360974386200019870, 1517.045004075700035, 205.0794574309270217 ) ) ;
#82957=CARTESIAN_POINT ( 'NONE',  ( 6.564578685215000320, 1517.199196846569976, 210.8299485595169926 ) ) ;
#82960=EDGE_CURVE ( 'NONE', #56695, #6679, #99198, .T. ) ;
#82989=CARTESIAN_POINT ( 'NONE',  ( -6.555393155154999540, 1516.809497469189864, 201.7937966518470034 ) ) ;
#82990=CARTESIAN_POINT ( 'NONE',  ( -7.727327152855000492, 1517.232977404109988, 207.4118332116069894 ) ) ;
#83001=CARTESIAN_POINT ( 'NONE',  ( -5.385694318444020467, 1511.434991102970116, 200.8007895389870043 ) ) ;
#83009=B_SPLINE_CURVE_WITH_KNOTS ( 'NONE', 3,
 ( #38964, #107286, #3758, #63128 ),
 .UNSPECIFIED., .F., .F.,
 ( 4, 4 ),
 ( 0.000000000000000000, 1.000000000000000000 ),
 .UNSPECIFIED. ) ;
#83010=CARTESIAN_POINT ( 'NONE',  ( -7.329303116114999739, 1516.857992118400034, 216.4524001036569985 ) ) ;
#83014=FACE_OUTER_BOUND ( 'NONE', #63712, .T. ) ;
#83015=CARTESIAN_POINT ( 'NONE',  ( 0.1364787244639666663, 1516.894040417452288, 216.8402977076042646 ) ) ;
#83016=CARTESIAN_POINT ( 'NONE',  ( 2.297085715815000206, 1516.718889242609976, 213.1486234561869821 ) ) ;
#83019=CARTESIAN_POINT ( 'NONE',  ( 4.534001422476420018, 1508.610336687640029, 213.3588515476280065 ) ) ;
#83034=CARTESIAN_POINT ( 'NONE',  ( 1.702405985064999960, 1516.999105586269934, 205.8518611507970206 ) ) ;
#83064=CARTESIAN_POINT ( 'NONE',  ( 8.143458402570486143, 1511.512562116153504, 205.2850637399104698 ) ) ;
#83080=CARTESIAN_POINT ( 'NONE',  ( -3.261635970955000019, 1516.613881697390070, 202.1867125516770045 ) ) ;
#83083=CARTESIAN_POINT ( 'NONE',  ( 16.65017489173500209, 1513.596256836700150, 195.0134922709670207 ) ) ;
#83099=AXIS2_PLACEMENT_3D ( 'NONE', #37852, #13716, #64173 ) ;
#83108=CARTESIAN_POINT ( 'NONE',  ( 7.538480495275000415, 1511.326779185850000, 202.9524984073069618 ) ) ;
#83117=CARTESIAN_POINT ( 'NONE',  ( 1.710004548794999968, 1516.557392317769882, 215.6678473207969944 ) ) ;
#83123=CARTESIAN_POINT ( 'NONE',  ( -6.949265684145000677, 1517.089216728169959, 205.6689289091970068 ) ) ;
#83125=CARTESIAN_POINT ( 'NONE',  ( -5.006259886824999228, 1516.939723362869927, 209.1347437590049765 ) ) ;
#83129=CARTESIAN_POINT ( 'NONE',  ( 6.383820954904999567, 1512.069761553120088, 217.4930739719970063 ) ) ;
#83140=CARTESIAN_POINT ( 'NONE',  ( -7.712490991114999694, 1516.666407245520077, 213.7387074786470009 ) ) ;
#83141=ADVANCED_FACE ( 'NONE', ( #79000 ), #63849, .F. ) ;
#83145=CARTESIAN_POINT ( 'NONE',  ( -7.709874534326499607, 1516.566488792059999, 210.6406471876519788 ) ) ;
#83146=CARTESIAN_POINT ( 'NONE',  ( 0.7579262867720020225, 1516.927039499179955, 210.8260166843570005 ) ) ;
#83161=CARTESIAN_POINT ( 'NONE',  ( -7.328676208015000526, 1516.833844030519913, 216.0648195994369871 ) ) ;
#83166=CARTESIAN_POINT ( 'NONE',  ( -7.719392420504999741, 1516.929962200689943, 202.5670673984569703 ) ) ;
#83168=CARTESIAN_POINT ( 'NONE',  ( -15.90990504886499757, 1514.921193539169963, 224.3246445042669848 ) ) ;
#83170=AXIS2_PLACEMENT_3D ( 'NONE', #1173, #103039, #103612 ) ;
#83202=CARTESIAN_POINT ( 'NONE',  ( 7.500396670941167798, 1516.934665496271919, 209.1219157010845322 ) ) ;
#83213=LINE ( 'NONE', #108972, #75026 ) ;
#83239=CARTESIAN_POINT ( 'NONE',  ( 2.493073829755000137, 1516.826109302209943, 211.9861720575370043 ) ) ;
#83242=CARTESIAN_POINT ( 'NONE',  ( 2.298048923505000118, 1516.764084769670262, 212.5672535042169784 ) ) ;
#83245=CARTESIAN_POINT ( 'NONE',  ( -2.942030012410809636, 1512.314860016870171, 201.2300683927209946 ) ) ;
#83248=CARTESIAN_POINT ( 'NONE',  ( 5.777745395274999751, 1516.908489800550115, 202.5639360494670029 ) ) ;
#83264=CARTESIAN_POINT ( 'NONE',  ( 6.951175128784999657, 1517.170721208160103, 211.4121022339570004 ) ) ;
#83270=CARTESIAN_POINT ( 'NONE',  ( 2.282301578035000222, 1516.836638729160086, 207.4044134838369757 ) ) ;
#83287=CARTESIAN_POINT ( 'NONE',  ( 2.292307230374999616, 1516.548716157039962, 216.0554627912370051 ) ) ;
#83289=CARTESIAN_POINT ( 'NONE',  ( 7.718113422873809526, 1516.881120708040044, 208.9373617900340037 ) ) ;
#83317=CARTESIAN_POINT ( 'NONE',  ( -4.827505465935000295, 1511.354819475749991, 200.9509497084369798 ) ) ;
#83355=CARTESIAN_POINT ( 'NONE',  ( 7.719640903004999721, 1516.939452820819952, 209.1117431028050078 ) ) ;
#83389=CARTESIAN_POINT ( 'NONE',  ( -4.554954834814580522, 1508.731366863229823, 205.6342592302619892 ) ) ;
#83392=CARTESIAN_POINT ( 'NONE',  ( 6.547881374914999775, 1516.647534046129977, 205.6658385469270058 ) ) ;
#83395=CARTESIAN_POINT ( 'NONE',  ( 15.30763528260880157, 1512.674009804160050, 195.6562266886770090 ) ) ;
#83401=CARTESIAN_POINT ( 'NONE',  ( -14.15402813869910048, 1513.231391185889834, 193.8860313682340006 ) ) ;
#83482=CARTESIAN_POINT ( 'NONE',  ( -6.561995998525000040, 1517.083030555940013, 205.8633713531569924 ) ) ;
#83492=CARTESIAN_POINT ( 'NONE',  ( -16.60697873886304876, 1513.055456493683550, 221.1753219165195219 ) ) ;
#83496=CARTESIAN_POINT ( 'NONE',  ( 0.01265818781360149997, 1516.959716008189844, 210.8316124642570060 ) ) ;
#83504=DIRECTION ( 'NONE',  ( -0.4999999999998399058, 0.7071067811867739472, 0.4999999999998399058 ) ) ;
#83526=CARTESIAN_POINT ( 'NONE',  ( -1.708721022705000037, 1516.531533746980131, 201.8006767011069940 ) ) ;
#83527=CARTESIAN_POINT ( 'NONE',  ( 6.935801261535000428, 1516.621991115350056, 207.9918434378369909 ) ) ;
#83540=CARTESIAN_POINT ( 'NONE',  ( -6.105460705908933861, 1510.769285144274590, 201.6400650806163242 ) ) ;
#83546=CARTESIAN_POINT ( 'NONE',  ( 2.485217193935000068, 1516.534320418310244, 216.8308781079170160 ) ) ;
#83549=DIRECTION ( 'NONE',  ( -0.02617694830788839730, 0.9996573249755569268, 0.000000000000000000 ) ) ;
#83551=CARTESIAN_POINT ( 'NONE',  ( 2.879642153204999833, 1516.812046502680005, 212.5681757458869754 ) ) ;
#83570=CARTESIAN_POINT ( 'NONE',  ( -6.949574985774999547, 1517.102359858469754, 205.8627441332170065 ) ) ;
#83584=CARTESIAN_POINT ( 'NONE',  ( -13.08147547106499964, 1513.492015765619954, 195.3332637180670019 ) ) ;
#83589=CARTESIAN_POINT ( 'NONE',  ( -15.20279846676549873, 1514.921193439789931, 193.2119408159660168 ) ) ;
#83612=CARTESIAN_POINT ( 'NONE',  ( -15.28532365586499964, 1514.287526756679881, 194.0255556049669963 ) ) ;
#83614=CARTESIAN_POINT ( 'NONE',  ( -6.805045110652309326, 1517.051704409849890, 205.2482747741559876 ) ) ;
#83618=CARTESIAN_POINT ( 'NONE',  ( -1.709358701255000001, 1516.542957540330008, 202.1882582765869927 ) ) ;
#83622=CARTESIAN_POINT ( 'NONE',  ( 15.37702282283500033, 1512.655881406850085, 195.6173956022669813 ) ) ;
#83636=CARTESIAN_POINT ( 'NONE',  ( -7.625190063675000296, 1512.177707669779920, 211.6636587291770013 ) ) ;
#83648=CARTESIAN_POINT ( 'NONE',  ( 7.396545043135000164, 1511.069621805459974, 202.7496783315469884 ) ) ;
#83652=EDGE_CURVE ( 'NONE', #11573, #110638, #31990, .T. ) ;
#83657=CARTESIAN_POINT ( 'NONE',  ( 1.130607463874999885, 1516.632821972880038, 215.6700465578769865 ) ) ;
#83659=ADVANCED_FACE ( 'NONE', ( #47458 ), #64272, .F. ) ;
#83665=CARTESIAN_POINT ( 'NONE',  ( -0.01328397755539850039, 1516.939580991450157, 205.8601936452070049 ) ) ;
#83667=CARTESIAN_POINT ( 'NONE',  ( 3.460866170685000132, 1517.020847257979995, 209.8575449048190080 ) ) ;
#83679=CARTESIAN_POINT ( 'NONE',  ( 4.039897278065000208, 1516.787536375099990, 214.1203611275269907 ) ) ;
#83687=CARTESIAN_POINT ( 'NONE',  ( 2.300729626665000360, 1516.923170579120097, 210.8225527465970117 ) ) ;
#83703=CARTESIAN_POINT ( 'NONE',  ( 3.260378255074999565, 1516.582197289609894, 216.8321318079170226 ) ) ;
#83709=CARTESIAN_POINT ( 'NONE',  ( 6.940473334145000450, 1516.833525648419936, 202.5658237375970145 ) ) ;
#83710=CARTESIAN_POINT ( 'NONE',  ( -16.22329233456500219, 1513.248517198770060, 223.4469878791670112 ) ) ;
#83732=CARTESIAN_POINT ( 'NONE',  ( -3.487586080072700323, 1508.611352721110052, 213.7999951061069908 ) ) ;
#83756=EDGE_CURVE ( 'NONE', #93856, #65412, #74844, .T. ) ;
#83757=CARTESIAN_POINT ( 'NONE',  ( -3.424720339024999838, 1517.051704408389924, 217.6596685689069943 ) ) ;
#83768=CARTESIAN_POINT ( 'NONE',  ( -10.96015512746500065, 1512.830284628050094, 193.2119433744669834 ) ) ;
#83784=ORIENTED_EDGE ( 'NONE', *, *, #50906, .T. ) ;
#83789=CARTESIAN_POINT ( 'NONE',  ( -1.118903308544999975, 1517.003078582959688, 212.0031713441969998 ) ) ;
#83790=CARTESIAN_POINT ( 'NONE',  ( 7.708815788408339920, 1516.526058372639909, 206.7773338513199803 ) ) ;
#83793=CARTESIAN_POINT ( 'NONE',  ( 7.723480079395000253, 1517.086065052259983, 213.1573821953169841 ) ) ;
#83799=CARTESIAN_POINT ( 'NONE',  ( -3.262264688434999726, 1516.633288330999903, 202.5742890007669814 ) ) ;
#83812=CARTESIAN_POINT ( 'NONE',  ( 5.788097227154999302, 1517.099836525840146, 211.6039138304569747 ) ) ;
#83817=CARTESIAN_POINT ( 'NONE',  ( 7.708745647785000266, 1516.523379810429788, 207.4137536659370085 ) ) ;
#83825=B_SPLINE_SURFACE_WITH_KNOTS ( 'NONE', 5, 5, ( 
 ( #52312, #28188, #44453, #87559, #95398, #53981 ),
 ( #71896, #37693, #27097, #97059, #46122, #79714 ),
 ( #78597, #2473, #86435, #1343, #70238, #104345 ),
 ( #35482, #10848, #9726, #20323, #1914, #79165 ),
 ( #11941, #36051, #36590, #95946, #88114, #11404 ),
 ( #37143, #26520, #60718, #43891, #69675, #103798 ) ),
 .UNSPECIFIED., .F., .F., .F.,
 ( 6, 6 ),
 ( 6, 6 ),
 ( 5.893385646620069807, 9.819835850959931278 ),
 ( -0.0002904017899300670230, 0.5000000000000000000 ),
 .UNSPECIFIED. ) ;
#83832=CARTESIAN_POINT ( 'NONE',  ( 7.334328272665000092, 1517.005755693489846, 214.1256940922069987 ) ) ;
#83834=AXIS2_PLACEMENT_3D ( 'NONE', #26751, #25631, #85537 ) ;
#83835=CARTESIAN_POINT ( 'NONE',  ( -7.321844861203470778, 1508.611350403038159, 214.6352815287768010 ) ) ;
#83836=CARTESIAN_POINT ( 'NONE',  ( -3.452289220704999551, 1517.069378699710114, 215.6835323934670328 ) ) ;
#83856=ORIENTED_EDGE ( 'NONE', *, *, #805, .T. ) ;
#83876=EDGE_LOOP ( 'NONE', ( #43418, #39033, #52465, #15054, #108366 ) ) ;
#83909=CARTESIAN_POINT ( 'NONE',  ( -3.455495871984999745, 1516.939877939420057, 209.1351200182310208 ) ) ;
#83921=CARTESIAN_POINT ( 'NONE',  ( -15.18091661680750093, 1512.335564144490036, 222.0139412780119983 ) ) ;
#83922=EDGE_CURVE ( 'NONE', #98379, #55385, #57913, .T. ) ;
#83947=CARTESIAN_POINT ( 'NONE',  ( -7.723480117524999855, 1517.086065052259983, 205.0863097070169943 ) ) ;
#83950=CARTESIAN_POINT ( 'NONE',  ( 15.28055237174110026, 1513.058738973280015, 195.1605214075740093 ) ) ;
#83954=AXIS2_PLACEMENT_3D ( 'NONE', #66576, #106879, #64913 ) ;
#83966=CARTESIAN_POINT ( 'NONE',  ( -7.770779690674999962, 1514.639648807489948, 203.1969910678269855 ) ) ;
#83971=B_SPLINE_SURFACE_WITH_KNOTS ( 'NONE', 5, 5, ( 
 ( #65441, #64892, #57593, #48075, #82768, #30706 ),
 ( #107963, #23940, #31260, #98999, #49187, #74943 ),
 ( #99551, #83317, #55931, #58135, #22836, #22276 ),
 ( #57041, #4951, #32371, #90050, #91716, #91167 ),
 ( #13333, #14443, #6061, #31812, #6612, #47525 ),
 ( #39093, #73270, #108520, #23404, #107410, #56478 ),
 ( #51661, #62866, #10765, #44372, #86907, #96419 ),
 ( #77956, #103135, #10197, #18031, #70702, #1262 ),
 ( #60630, #28661, #35401, #17460, #27008, #52223 ),
 ( #45490, #85799, #43806, #19697, #9097, #43262 ),
 ( #26435, #70151, #77409, #86350, #715, #1828 ),
 ( #61196, #69589, #37052, #95313, #18573, #19126 ) ),
 .UNSPECIFIED., .F., .F., .F.,
 ( 6, 3, 3, 6 ),
 ( 6, 6 ),
 ( 3.686514310900000257, 6.076675143260000134, 7.815970586829999789, 8.927001670169998349 ),
 ( 0.000000000000000000, 1.000000000000000000 ),
 .UNSPECIFIED. ) ;
#84024=EDGE_CURVE ( 'NONE', #71879, #71004, #58615, .T. ) ;
#84026=EDGE_LOOP ( 'NONE', ( #99030, #81861, #67970, #455, #12468, #66868 ) ) ;
#84041=CARTESIAN_POINT ( 'NONE',  ( 5.771797426184999580, 1516.647618671360078, 206.2459958378869942 ) ) ;
#84050=CARTESIAN_POINT ( 'NONE',  ( -16.72494119730692219, 1513.190421808320480, 221.5564311681714571 ) ) ;
#84054=CARTESIAN_POINT ( 'NONE',  ( -2.864043456445000135, 1516.811292230880099, 211.4208600009669965 ) ) ;
#84078=CARTESIAN_POINT ( 'NONE',  ( 1.275439612931326350, 1516.597747112960633, 216.5200775691153865 ) ) ;
#84083=CARTESIAN_POINT ( 'NONE',  ( -1.130002532395000037, 1516.621991115350056, 202.1860446705670142 ) ) ;
#84084=CARTESIAN_POINT ( 'NONE',  ( -0.7533003905399979772, 1516.992029636990083, 208.3816250717139837 ) ) ;
#84085=ORIENTED_EDGE ( 'NONE', *, *, #106868, .T. ) ;
#84087=CARTESIAN_POINT ( 'NONE',  ( 4.873051833723480719, 1511.395873688979691, 217.6024705955157970 ) ) ;
#84094=DIRECTION ( 'NONE',  ( 0.02616798426500960631, 0.9993150019883682011, -0.02616798426500970345 ) ) ;
#84103=CARTESIAN_POINT ( 'NONE',  ( 2.872700517194999748, 1516.559109716219837, 216.8315272385270021 ) ) ;
#84107=CARTESIAN_POINT ( 'NONE',  ( -4.030514550714999977, 1516.901952101700090, 213.7446888144170032 ) ) ;
#84113=AXIS2_PLACEMENT_3D ( 'NONE', #2228, #11700, #104653 ) ;
#84125=CARTESIAN_POINT ( 'NONE',  ( 1.119717716265000051, 1517.038650117239968, 205.6590103047369951 ) ) ;
#84172=CARTESIAN_POINT ( 'NONE',  ( -2.874588960795000148, 1516.606339319019980, 202.5748942495170013 ) ) ;
#84176=CARTESIAN_POINT ( 'NONE',  ( 16.23061965993500166, 1512.609537213029853, 197.8388957390669987 ) ) ;
#84206=EDGE_CURVE ( 'NONE', #68158, #23166, #51815, .T. ) ;
#84207=LINE ( 'NONE', #25385, #1948 ) ;
#84210=CARTESIAN_POINT ( 'NONE',  ( 4.617490466775000080, 1516.685667699390024, 216.4467608883869900 ) ) ;
#84211=CARTESIAN_POINT ( 'NONE',  ( -8.517173909402618648, 1511.399508273092124, 214.1045348855529369 ) ) ;
#84214=CARTESIAN_POINT ( 'NONE',  ( -4.590060415194109567, 1517.051704403100075, 216.8444262830430205 ) ) ;
#84217=CARTESIAN_POINT ( 'NONE',  ( 3.253141137235000091, 1516.858171774179937, 205.8542424163969997 ) ) ;
#84222=CARTESIAN_POINT ( 'NONE',  ( 7.570419115124999543, 1513.830194289070278, 215.4430188042069858 ) ) ;
#84230=CARTESIAN_POINT ( 'NONE',  ( 6.559168636745000391, 1516.960844870249957, 214.1244393295569921 ) ) ;
#84234=CARTESIAN_POINT ( 'NONE',  ( 7.096078592938200202, 1508.610125760119899, 215.7702303952080172 ) ) ;
#84236=CARTESIAN_POINT ( 'NONE',  ( -2.864043456445000135, 1516.811292230880099, 211.4208600009669965 ) ) ;
#84244=EDGE_LOOP ( 'NONE', ( #57813, #59008, #103485, #45535 ) ) ;
#84255=CARTESIAN_POINT ( 'NONE',  ( 4.035490712554999249, 1516.630499592039996, 216.8333966482170183 ) ) ;
#84260=CARTESIAN_POINT ( 'NONE',  ( 6.551643386774999023, 1516.807958722750072, 203.3403553877570005 ) ) ;
#84261=CARTESIAN_POINT ( 'NONE',  ( 7.260305718849559220, 1509.032998983409925, 215.6421393903620753 ) ) ;
#84283=CARTESIAN_POINT ( 'NONE',  ( -3.487584424475879796, 1508.551704408389924, 214.1089243866350103 ) ) ;
#84288=DIRECTION ( 'NONE',  ( -0.8236474686100957454, 0.5669078173028199163, -0.01484500364209119690 ) ) ;
#84295=CARTESIAN_POINT ( 'NONE',  ( 2.229731609205000353, 1512.142919181319940, 216.7158852195469763 ) ) ;
#84341=CARTESIAN_POINT ( 'NONE',  ( 1.134357970594999987, 1516.744381837270112, 213.1504571913470159 ) ) ;
#84343=CARTESIAN_POINT ( 'NONE',  ( 5.399591297624999342, 1511.369014903080142, 217.1050657870570149 ) ) ;
#84347=CARTESIAN_POINT ( 'NONE',  ( -2.487103457664999961, 1516.577434278289957, 202.5755431900869894 ) ) ;
#84364=CARTESIAN_POINT ( 'NONE',  ( -3.251394400264999707, 1516.757508073510053, 210.8375504612070017 ) ) ;
#84372=CARTESIAN_POINT ( 'NONE',  ( -4.626591905484999323, 1517.096587378560116, 207.4170511287669854 ) ) ;
#84389=CARTESIAN_POINT ( 'NONE',  ( 3.458526497885000328, 1516.742629295279812, 214.1194197574270106 ) ) ;
#84392=CARTESIAN_POINT ( 'NONE',  ( -0.7391220051939990654, 1517.130100026000036, 216.0715493048870144 ) ) ;
#84394=CARTESIAN_POINT ( 'NONE',  ( 7.721597366031249798, 1517.014167129519819, 209.4083824335259862 ) ) ;
#84411=EDGE_LOOP ( 'NONE', ( #5594, #47633, #55569, #109728, #28948, #28972 ) ) ;
#84415=CIRCLE ( 'NONE', #37667, 7.500000000000000000 ) ;
#84449=LINE ( 'NONE', #84981, #96625 ) ;
#84468=CARTESIAN_POINT ( 'NONE',  ( -2.292217048824999992, 1516.941178807709775, 209.1350424789999920 ) ) ;
#84487=CARTESIAN_POINT ( 'NONE',  ( -7.512750246095000861, 1509.038615934239942, 214.6352815282469919 ) ) ;
#84499=CARTESIAN_POINT ( 'NONE',  ( 6.548821941055000373, 1516.688761843659904, 205.0844676760469838 ) ) ;
#84502=CARTESIAN_POINT ( 'NONE',  ( 15.30900797519679912, 1512.850289816009990, 195.4165148025099938 ) ) ;
#84517=CARTESIAN_POINT ( 'NONE',  ( -3.487592469391230132, 1509.038615938009798, 204.6345961782960217 ) ) ;
#84549=CARTESIAN_POINT ( 'NONE',  ( 2.297085715815000206, 1516.718889242609976, 213.1486234561869821 ) ) ;
#84553=VERTEX_POINT ( 'NONE', #78169 ) ;
#84589=CARTESIAN_POINT ( 'NONE',  ( 4.028307740155000261, 1516.797038924770050, 205.8554964580370097 ) ) ;
#84598=CARTESIAN_POINT ( 'NONE',  ( -16.20149550001009686, 1514.624327922590282, 223.9881805485040616 ) ) ;
#84602=CARTESIAN_POINT ( 'NONE',  ( -5.770820179264999794, 1516.591755933730155, 210.8331571987770019 ) ) ;
#84608=SHAPE_DEFINITION_REPRESENTATION ( #108163, #60858 ) ;
#84618=DIRECTION ( 'NONE',  ( -0.7071067811865474617, -4.750184379286195842E-17, -0.7071067811865474617 ) ) ;
#84623=CARTESIAN_POINT ( 'NONE',  ( 2.282008349603394048, 1516.544479074524361, 216.2688515719049462 ) ) ;
#84628=CARTESIAN_POINT ( 'NONE',  ( -5.780232115465000042, 1516.760434454289907, 201.7950504087270076 ) ) ;
#84629=CARTESIAN_POINT ( 'NONE',  ( 4.042388501175000037, 1517.045004075700035, 209.8579434088520088 ) ) ;
#84654=CARTESIAN_POINT ( 'NONE',  ( -0.7369042090349989804, 1517.080322339569875, 214.1333973382469935 ) ) ;
#84670=ORIENTED_EDGE ( 'NONE', *, *, #43456, .F. ) ;
#84671=CARTESIAN_POINT ( 'NONE',  ( -2.298369507954999946, 1516.779243033999819, 205.8702346062869992 ) ) ;
#84712=CARTESIAN_POINT ( 'NONE',  ( -15.33574365116500182, 1514.703592237370003, 193.3867305263669891 ) ) ;
#84715=CARTESIAN_POINT ( 'NONE',  ( -6.701092706527290055, 1517.051709179880163, 205.3286261131629828 ) ) ;
#84716=CARTESIAN_POINT ( 'NONE',  ( 7.722580314274999580, 1517.051704408389924, 210.6910072246569996 ) ) ;
#84719=CARTESIAN_POINT ( 'NONE',  ( -2.292940207144999576, 1516.565291103010168, 202.5758065368070220 ) ) ;
#84722=CARTESIAN_POINT ( 'NONE',  ( 16.28235094783499903, 1514.570049710740022, 194.2914897994669730 ) ) ;
#84735=CARTESIAN_POINT ( 'NONE',  ( 15.90990255763500016, 1516.814170398969964, 193.9190501556669801 ) ) ;
#84746=CARTESIAN_POINT ( 'NONE',  ( 6.439137434935000570, 1514.557408760799945, 201.1783224906369867 ) ) ;
#84755=CARTESIAN_POINT ( 'NONE',  ( 4.035490712554999249, 1516.630499592039996, 216.8333966482170183 ) ) ;
#84756=CARTESIAN_POINT ( 'NONE',  ( -8.150371712873907271, 1511.506728505250976, 212.9804710034640038 ) ) ;
#84762=CARTESIAN_POINT ( 'NONE',  ( 6.546951682585000043, 1516.606339319019980, 206.2472570094369928 ) ) ;
#84767=CARTESIAN_POINT ( 'NONE',  ( 7.378505815095000031, 1513.311928781879942, 216.7671994646370024 ) ) ;
#84776=CARTESIAN_POINT ( 'NONE',  ( -1.703779643355000095, 1517.057265928030120, 213.1670284501570052 ) ) ;
#84780=CARTESIAN_POINT ( 'NONE',  ( 6.725587746340760731, 1508.728101425929935, 216.3255536485930293 ) ) ;
#84781=CARTESIAN_POINT ( 'NONE',  ( -3.445407572115000150, 1516.764084769670262, 211.4198948937369948 ) ) ;
#84794=CARTESIAN_POINT ( 'NONE',  ( -1.710012758625000018, 1517.232977404109988, 216.8491730849570160 ) ) ;
#84795=CARTESIAN_POINT ( 'NONE',  ( -5.303300877965000382, 1513.301704408390151, 198.8687976239669979 ) ) ;
#84799=CARTESIAN_POINT ( 'NONE',  ( -2.292940207144999576, 1516.565291103010168, 202.5758065368070220 ) ) ;
#84818=CARTESIAN_POINT ( 'NONE',  ( -7.599227184291730275, 1512.341036968809931, 211.3567690145959830 ) ) ;
#84828=CARTESIAN_POINT ( 'NONE',  ( 4.427981723884999887, 1510.423579818969984, 216.6708627338570068 ) ) ;
#84836=CARTESIAN_POINT ( 'NONE',  ( 7.467587119939531171, 1516.687838964707225, 208.2872662270863486 ) ) ;
#84877=CARTESIAN_POINT ( 'NONE',  ( 1.712644716155000024, 1516.636036526019780, 214.1174694231270053 ) ) ;
#84878=CARTESIAN_POINT ( 'NONE',  ( 5.385523161694999672, 1511.435001052829875, 217.7746220723570048 ) ) ;
#84885=CARTESIAN_POINT ( 'NONE',  ( 3.259101798884999734, 1517.102359858469754, 202.1722709844570147 ) ) ;
#84901=CARTESIAN_POINT ( 'NONE',  ( -7.321169269124999879, 1516.531533746980131, 210.8305669548069829 ) ) ;
#84906=CARTESIAN_POINT ( 'NONE',  ( -0.007128875282218469743, 1517.006509894990131, 208.3750284165899984 ) ) ;
#84921=CARTESIAN_POINT ( 'NONE',  ( -2.480187054844999572, 1517.025470194390209, 213.7472054950769973 ) ) ;
#84924=CARTESIAN_POINT ( 'NONE',  ( -3.260357166894999992, 1517.133889586189980, 216.8465783791270098 ) ) ;
#84926=CARTESIAN_POINT ( 'NONE',  ( 7.720004413545239252, 1516.953334728320215, 209.1872673121889932 ) ) ;
#84950=ADVANCED_FACE ( 'NONE', ( #7534 ), #65184, .T. ) ;
#84963=B_SPLINE_SURFACE_WITH_KNOTS ( 'NONE', 5, 5, ( 
 ( #65831, #4263, #56316, #90449, #38396, #107813, #64182, #13726, #55787 ),
 ( #31099, #40057, #74237, #108368, #20475, #54685, #88811, #72572, #106699 ),
 ( #12095, #89903, #13174, #77390, #94169, #1806, #43784, #41162, #44349 ),
 ( #60051, #103686, #693, #9614, #26415, #34271, #100511, #18554, #77934 ),
 ( #26987, #1241, #78492, #95292, #94730, #66392, #32211, #18008, #91567 ),
 ( #85774, #23790, #75337, #52747, #83710, #15390, #57979, #14843, #6460 ),
 ( #51637, #35378, #17439, #150, #23243, #49032, #52201, #86329, #68453 ),
 ( #9074, #86881, #10175, #57442, #103114, #43242, #92113, #35943, #99948 ),
 ( #69567, #34822, #61175, #69009, #74779, #60607, #40608, #25849, #83168 ) ),
 .UNSPECIFIED., .F., .F., .F.,
 ( 6, 3, 6 ),
 ( 6, 3, 6 ),
 ( 9.902195898180000455, 12.38020728900000123, 16.40090783169999966 ),
 ( 0.000000000000000000, 0.5000000000000000000, 1.000000000000000000 ),
 .UNSPECIFIED. ) ;
#84966=VERTEX_POINT ( 'NONE', #97617 ) ;
#84981=CARTESIAN_POINT ( 'NONE',  ( -1.906460855849449881E-08, 1515.051704408389924, 204.7920544413669859 ) ) ;
#84988=PLANE ( 'NONE',  #83834 ) ;
#85006=CARTESIAN_POINT ( 'NONE',  ( 1.127928333405000094, 1516.989863902050047, 209.1117210464550169 ) ) ;
#85011=ADVANCED_FACE ( 'NONE', ( #83014 ), #57832, .F. ) ;
#85013=VERTEX_POINT ( 'NONE', #107109 ) ;
#85016=CARTESIAN_POINT ( 'NONE',  ( -15.29028528244239915, 1512.571279492540043, 222.4326579091490146 ) ) ;
#85039=VECTOR ( 'NONE', #8282, 1000.000000000000000 ) ;
#85040=CARTESIAN_POINT ( 'NONE',  ( -4.236980942262600358, 1508.610336716400070, 204.5878351888970030 ) ) ;
#85042=CARTESIAN_POINT ( 'NONE',  ( -2.879642191334999879, 1516.812046502680005, 205.6755161564470313 ) ) ;
#85045=CARTESIAN_POINT ( 'NONE',  ( 15.25688964212639931, 1512.464953430890091, 195.9853556598569924 ) ) ;
#85070=DIRECTION ( 'NONE',  ( 0.000000000000000000, -6.123233995736769734E-17, -1.000000000000000000 ) ) ;
#85080=EDGE_CURVE ( 'NONE', #4206, #36027, #51758, .T. ) ;
#85081=DIRECTION ( 'NONE',  ( -0.9996573249755689172, 0.02617694830742899742, -1.602875797806941519E-18 ) ) ;
#85091=CARTESIAN_POINT ( 'NONE',  ( 5.785582913545000316, 1516.981965530290154, 213.1542438721070027 ) ) ;
#85135=EDGE_CURVE ( 'NONE', #60389, #8432, #543, .T. ) ;
#85139=CARTESIAN_POINT ( 'NONE',  ( 6.546951682585000043, 1516.606339319019980, 206.2472570094369928 ) ) ;
#85153=CARTESIAN_POINT ( 'NONE',  ( -4.026614517785000125, 1516.699825673279975, 210.8361802174170236 ) ) ;
#85165=ADVANCED_FACE ( 'NONE', ( #104077 ), #32614, .T. ) ;
#85177=CARTESIAN_POINT ( 'NONE',  ( 4.327793175846784024, 1516.734711358257528, 215.2529812453810223 ) ) ;
#85182=CARTESIAN_POINT ( 'NONE',  ( -3.262264688434999726, 1516.633288330999903, 202.5742890007669814 ) ) ;
#85183=CARTESIAN_POINT ( 'NONE',  ( 1.133653140995000141, 1516.978425811520083, 209.8592968530090275 ) ) ;
#85204=CARTESIAN_POINT ( 'NONE',  ( 0.7899257907088232944, 1516.710726079306141, 216.8354974527231036 ) ) ;
#85207=CARTESIAN_POINT ( 'NONE',  ( 4.159841809088510978, 1508.728286212990042, 213.5483455248779876 ) ) ;
#85221=CARTESIAN_POINT ( 'NONE',  ( 4.996642160164999957, 1516.697242742309982, 206.2447328616370044 ) ) ;
#85242=CARTESIAN_POINT ( 'NONE',  ( -14.59144169897830956, 1514.407829430023639, 192.7405808733855395 ) ) ;
#85268=CARTESIAN_POINT ( 'NONE',  ( -7.719392420504999741, 1516.929962200689943, 202.5670673984569703 ) ) ;
#85302=CARTESIAN_POINT ( 'NONE',  ( -4.035536263215000474, 1517.086065052259983, 216.8453260496270047 ) ) ;
#85303=CARTESIAN_POINT ( 'NONE',  ( -8.003699198419786498, 1511.683921177773755, 212.5077785452298826 ) ) ;
#85310=CARTESIAN_POINT ( 'NONE',  ( 4.027051405805000428, 1516.733363207009916, 206.6306575737070261 ) ) ;
#85315=CARTESIAN_POINT ( 'NONE',  ( 7.469619891705000292, 1513.342361861140034, 216.8722327131270049 ) ) ;
#85320=B_SPLINE_CURVE_WITH_KNOTS ( 'NONE', 5,
 ( #82645, #56348, #13205, #91028, #20503, #89390 ),
 .UNSPECIFIED., .F., .F.,
 ( 6, 6 ),
 ( 4.250950522260000142, 7.082025451739999866 ),
 .UNSPECIFIED. ) ;
#85321=CARTESIAN_POINT ( 'NONE',  ( -6.372167638625000130, 1511.069621805459974, 201.7253008890070021 ) ) ;
#85325=CARTESIAN_POINT ( 'NONE',  ( -2.868433836634999512, 1517.020727862619879, 214.1341630384669941 ) ) ;
#85328=CARTESIAN_POINT ( 'NONE',  ( 5.513240537208758951, 1508.551563895499839, 216.2888651833050062 ) ) ;
#85329=CARTESIAN_POINT ( 'NONE',  ( 2.493699768634999536, 1516.858326417339867, 211.5985794462469869 ) ) ;
#85348=CARTESIAN_POINT ( 'NONE',  ( 3.451033388965000004, 1517.025653221279981, 203.3353183697670090 ) ) ;
#85425=CARTESIAN_POINT ( 'NONE',  ( -2.479246885834999858, 1516.983612918759945, 213.1658362778269691 ) ) ;
#85433=CARTESIAN_POINT ( 'NONE',  ( -2.877113108595000135, 1516.697242742309982, 204.1252037719370094 ) ) ;
#85439=CARTESIAN_POINT ( 'NONE',  ( -6.153783059604999828, 1516.954809569559984, 216.8418890038570055 ) ) ;
#85447=CARTESIAN_POINT ( 'NONE',  ( -4.995994825704999975, 1516.665179208830068, 211.6114635085770033 ) ) ;
#85451=CARTESIAN_POINT ( 'NONE',  ( -6.562094107424999656, 1517.122674412569950, 208.3832410274270046 ) ) ;
#85467=CARTESIAN_POINT ( 'NONE',  ( 5.782749401605000727, 1516.858301627840092, 214.8983370654769942 ) ) ;
#85468=CARTESIAN_POINT ( 'NONE',  ( 7.599227146160510316, 1512.341036968809931, 206.8869228877400133 ) ) ;
#85474=VERTEX_POINT ( 'NONE', #88421 ) ;
#85500=VECTOR ( 'NONE', #95309, 1000.000000000000114 ) ;
#85507=CARTESIAN_POINT ( 'NONE',  ( -2.048720034851359895, 1516.528429087750055, 201.4129680643380027 ) ) ;
#85537=DIRECTION ( 'NONE',  ( -1.000000000000000000, 0.000000000000000000, 0.000000000000000000 ) ) ;
#85553=CARTESIAN_POINT ( 'NONE',  ( -3.261652325025000021, 1516.939580991450157, 209.1351299096569960 ) ) ;
#85563=CARTESIAN_POINT ( 'NONE',  ( 5.004475574535000248, 1517.026025493960105, 201.3999380438669959 ) ) ;
#85587=CARTESIAN_POINT ( 'NONE',  ( 7.322105067625000352, 1516.572193931679976, 206.2485165713470110 ) ) ;
#85590=CARTESIAN_POINT ( 'NONE',  ( 15.16689668216860021, 1513.426431439620046, 194.7669068285340188 ) ) ;
#85595=CARTESIAN_POINT ( 'NONE',  ( -14.81380081930790027, 1513.941944658620059, 194.2161487120590095 ) ) ;
#85640=CARTESIAN_POINT ( 'NONE',  ( -6.936398393775000670, 1516.667393516340098, 213.1585948090369698 ) ) ;
#85669=CIRCLE ( 'NONE', #108949, 0.9999999999998898659 ) ;
#85676=ORIENTED_EDGE ( 'NONE', *, *, #94494, .F. ) ;
#85689=CARTESIAN_POINT ( 'NONE',  ( 3.253141137235000091, 1516.858171774179937, 205.8542424163969997 ) ) ;
#85700=CARTESIAN_POINT ( 'NONE',  ( -16.78028220709281726, 1513.363094763815525, 221.9574106988646065 ) ) ;
#85704=CARTESIAN_POINT ( 'NONE',  ( 3.462948796544999652, 1516.956048353049937, 211.4063724288770061 ) ) ;
#85705=ADVANCED_FACE ( 'NONE', ( #23817 ), #55816, .F. ) ;
#85717=ORIENTED_EDGE ( 'NONE', *, *, #53861, .F. ) ;
#85725=AXIS2_PLACEMENT_3D ( 'NONE', #39349, #49417, #108200 ) ;
#85732=CARTESIAN_POINT ( 'NONE',  ( 1.706797785944999868, 1517.164987839469859, 203.3324512698969784 ) ) ;
#85733=CARTESIAN_POINT ( 'NONE',  ( -7.332063977575000280, 1516.939491476980038, 209.1325772641960157 ) ) ;
#85738=CARTESIAN_POINT ( 'NONE',  ( 2.968351152030138440, 1512.111360402368518, 217.0109328861994982 ) ) ;
#85759=CARTESIAN_POINT ( 'NONE',  ( -4.487358994564536907, 1509.034509900238845, 205.3201110865223029 ) ) ;
#85773=CARTESIAN_POINT ( 'NONE',  ( 9.258462863084998773, 1517.051704408389924, 196.7308630447670055 ) ) ;
#85774=CARTESIAN_POINT ( 'NONE',  ( -15.29601662286500030, 1513.169116394660023, 223.2466004030669922 ) ) ;
#85780=VECTOR ( 'NONE', #39559, 1000.000000000000000 ) ;
#85781=CARTESIAN_POINT ( 'NONE',  ( 1.701729820345000199, 1516.969638403840008, 206.2395199527169893 ) ) ;
#85786=EDGE_CURVE ( 'NONE', #10258, #1893, #74423, .T. ) ;
#85791=CARTESIAN_POINT ( 'NONE',  ( -1.906499846882070084E-08, 1516.801704408389924, 209.1218459511669892 ) ) ;
#85799=CARTESIAN_POINT ( 'NONE',  ( -2.841932056525000139, 1512.089957059379913, 201.3490862420470080 ) ) ;
#85805=CARTESIAN_POINT ( 'NONE',  ( -14.31745300034082291, 1514.209337176663212, 192.5996944249964429 ) ) ;
#85806=EDGE_CURVE ( 'NONE', #40123, #74608, #73022, .T. ) ;
#85821=B_SPLINE_SURFACE_WITH_KNOTS ( 'NONE', 5, 5, ( 
 ( #28826, #105539, #36672, #70310, #37227, #96020, #70865, #72489, #78674, #46199, #104977, #27716, #37779, #3650, #28267, #45653, #63024, #106080, #53491, #20946, #12018, #62460, #3097, #71423, #80333, #55152, #63559, #1991, #61355, #96583, #10923, #45099, #89273 ),
 ( #52935, #44528, #12570, #19855, #79239, #46750, #95474, #18741, #80881, #2547, #4177, #87071, #98770, #91482, #5831, #30465, #64097, #73598, #22579, #4712, #90921, #13637, #6916, #106618, #73034, #22032, #39421, #107728, #57895, #55700, #5266, #108828, #47277 ),
 ( #31013, #82536, #15302, #66310, #65193, #41072, #29904, #14761, #98218, #49494, #89821, #99305, #39972, #38855, #56229, #107173, #6373, #92030, #90359, #83618, #40519, #48949, #21488, #83080, #64651, #32125, #56783, #14207, #48393, #13093, #81400, #74147, #47826 ),
 ( #108278, #100427, #31565, #65741, #23156, #81960, #99859, #57358, #74696, #23710, #52260, #32675, #93126, #34878, #50044, #101506, #109399, #66854, #94789, #50588, #84719, #100963, #84172, #16393, #8565, #75788, #69067, #207, #103167, #8018, #42185, #59546, #85268 ),
 ( #76898, #42737, #76335, #7471, #34331, #109940, #110485, #86385, #15839, #94222, #33764, #41633, #85835, #51694, #67961, #93659, #68508, #9135, #33218, #26468, #25907, #102071, #60663, #18066, #24260, #58440, #25353, #92567, #43298, #9673, #58998, #67407, #24793 ),
 ( #16940, #102607, #51142, #60105, #17496, #77447, #75250, #748, #29244, #54479, #28697, #1294, #97013, #78548, #80201, #87509, #28138, #36541, #97552, #103744, #53934, #61232, #27046, #70189, #20275, #37089, #69622, #104298, #88615, #37644, #55021, #95347, #71292 ),
 ( #2972, #1864, #89148, #27587, #19733, #88068, #11896, #77989, #53363, #35998, #20825, #10230, #35435, #45526, #43843, #18608, #52807, #105405, #86939, #62903, #46070, #3519, #44407, #79667, #11356, #10799, #61770, #71850, #95896, #44969, #19157, #79116, #105966 ),
 ( #63434, #2424, #70738, #104850, #62328, #96453, #6233, #57772, #21360, #98088, #90231, #12433, #5136, #38188, #29788, #82942, #56102, #55566, #81832, #46623, #23582, #23021, #81282, #74563, #99175, #4598, #108142, #22456, #47156, #80755, #13515, #39291, #89692 ),
 ( #100298, #12973, #31435, #65616, #48819, #48263, #82406, #4063, #56657, #64523, #38732, #72370, #72908, #90791, #14073, #91353, #106500, #21905, #107047, #63975, #30333, #98638, #5702, #66179, #47703, #73465, #39847, #107598, #74010, #57224, #14633, #30881, #99729 ),
 ( #65061, #40386, #108698, #31989, #16262, #40939, #103032, #84589, #67272, #85689, #24115, #26329, #50465, #42050, #109264, #8987, #91891, #100827, #66724, #58856, #15166, #7880, #6776, #32549, #51554, #24655, #58307, #76201, #49354, #83482, #102484, #49906, #43158 ),
 ( #25773, #75117, #110346, #85139, #84041, #33621, #92428, #67816, #59972, #68932, #15704, #61, #34192, #17358, #16803, #51006, #7339, #25217, #33083, #41504, #34742, #59421, #92987, #101930, #612, #77314, #93533, #75662, #109805, #76750, #101365, #8425, #42596 ),
 ( #68376, #94088, #103604, #71140, #45921, #86802, #80055, #105260, #45382, #17919, #2825, #95208, #96871, #104156, #44828, #53224, #3376, #9536, #70588, #77857, #43704, #10093, #36943, #53793, #86245, #44267, #28554, #54334, #71709, #1166, #87930, #62753, #37503 ),
 ( #20140, #11219, #105827, #26903, #61625, #35861, #88466, #60524, #52116, #78409, #11750, #35296, #1721, #94646, #69481, #61092, #70045, #27443, #18469, #52666, #95757, #104704, #19022, #87364, #96310, #10659, #78981, #2285, #36397, #27999, #62184, #19589, #79520 ),
 ( #48121, #21769, #20677, #64379, #89000, #40255, #55970, #4464, #22876, #72235, #74437, #98501, #90094, #46481, #57086, #29105, #38057, #3928, #106900, #63291, #13377, #54876, #80614, #99593, #72772, #106360, #47565, #97406, #12287, #39711, #97944, #91209, #4995 ),
 ( #29646, #81689, #22320, #21213, #39140, #63833, #73316, #108003, #6100, #55421, #82260, #5560, #65484, #64929, #99042, #89555, #107453, #81151, #12844, #82807, #30748, #30186, #56522, #48683, #14491, #90649, #47025, #38593, #13933, #73875, #31300, #91756, #7215 ),
 ( #109674, #76621, #23983, #23448, #92860, #93962, #57643, #92306, #41921, #41373, #75539, #76077, #100163, #110773, #66597, #8301, #32418, #50876, #15032, #68256, #8850, #110217, #102363, #50343, #24537, #93412, #66040, #17227, #49230, #32950, #33490, #6654, #58178 ),
 ( #83355, #16136, #51423, #40807, #15576, #67692, #67139, #101237, #101800, #74986, #34063, #100701, #42462, #49778, #85006, #109134, #25648, #43032, #25090, #59838, #84468, #58725, #59295, #85553, #83909, #7756, #16678, #108563, #31853, #34617, #95083, #36831, #51985 ),
 ( #10524, #45258, #493, #86673, #69352, #54215, #43583, #68802, #78846, #20019, #102903, #60390, #70464, #86126, #36274, #11091, #79393, #77732, #2157, #44699, #9969, #9420, #87235, #1045, #44140, #88340, #17785, #96186, #78274, #35167, #87805, #53661, #1588 ),
 ( #94511, #71021, #11631, #103462, #26769, #35725, #77190, #69913, #26202, #60956, #105141, #104026, #18349, #27321, #52541, #61503, #2706, #95632, #28431, #53096, #18901, #62061, #104585, #27880, #19462, #62631, #96748, #54758, #30068, #63716, #56951, #45809, #12173 ),
 ( #81569, #4873, #79942, #89982, #97826, #46363, #99469, #13256, #46913, #21654, #65362, #5431, #81035, #91080, #3258, #37944, #22748, #80498, #37385, #47445, #71586, #105707, #28989, #39015, #88888, #73193, #90529, #47991, #3814, #107338, #30633, #55306, #72124 ),
 ( #89440, #63177, #97283, #64821, #12731, #106240, #56397, #22201, #4345, #64259, #98929, #13805, #29526, #39588, #82129, #38475, #72652, #98383, #73760, #107883, #55862, #20554, #21104, #106778, #31173, #23320, #9160, #108443, #18089, #85859, #91637, #60690, #27071 ),
 ( #6532, #75411, #65909, #109551, #94813, #103769, #14913, #34901, #69088, #52284, #51724, #43324, #14363, #60128, #66470, #49105, #69648, #94246, #15461, #102630, #35458, #86409, #49654, #61255, #48555, #773, #82692, #5982, #31724, #23861, #17520, #57512, #40684 ),
 ( #40130, #34355, #1317, #74313, #109001, #77471, #58054, #92189, #103189, #100028, #9698, #83239, #26494, #74857, #43866, #32286, #78010, #100579, #83789, #7084, #68532, #41239, #25930, #29262, #70213, #36562, #44990, #11915, #63455, #52830, #10820, #80224, #36022 ),
 ( #45547, #46092, #95370, #2446, #19179, #70759, #104871, #105987, #44427, #28160, #3541, #104317, #97573, #71871, #10251, #78571, #62349, #1886, #37665, #20845, #79137, #95917, #27611, #79686, #88637, #88088, #18634, #96473, #86960, #19753, #53383, #97034, #61796 ),
 ( #87532, #11375, #53954, #2992, #37112, #71312, #105427, #28716, #62923, #20297, #54501, #101883, #67770, #16, #26856, #77814, #110302, #34150, #61043, #78366, #95715, #33578, #1123, #95167, #61582, #43662, #8383, #18980, #68335, #60477, #17873, #52623, #7838 ),
 ( #42006, #93490, #102442, #52071, #85091, #44222, #9495, #1673, #25728, #51508, #68889, #94595, #84549, #94047, #76155, #50964, #42551, #103553, #77273, #25174, #8940, #59378, #16761, #571, #59930, #35814, #76703, #17313, #43114, #34697, #85640, #69997, #102991 ),
 ( #26288, #86204, #35254, #69438, #104111, #18423, #86761, #10049, #27399, #42947, #17698, #68714, #16057, #9340, #33978, #50260, #77106, #68173, #92781, #15504, #25009, #84921, #67059, #42379, #75988, #69265, #58102, #24459, #59210, #43502, #7134, #67607, #60302 ),
 ( #86042, #83832, #41289, #101716, #75463, #102819, #77646, #41832, #84389, #109597, #102280, #26113, #110686, #960, #93329, #94422, #7676, #32869, #76535, #35084, #101165, #110138, #25561, #16592, #50789, #59754, #49703, #51902, #33411, #103371, #8214, #414, #58648 ),
 ( #93875, #34532, #51332, #17141, #85467, #92233, #8766, #37855, #86591, #54130, #37305, #3725, #96662, #61423, #72041, #87149, #2621, #70940, #105619, #60874, #36198, #18819, #26675, #103944, #95000, #28346, #80411, #18268, #9883, #19933, #35633, #88258, #71500 ),
 ( #70382, #52461, #27242, #95546, #45727, #19370, #44051, #61979, #78190, #1502, #53573, #2067, #20468, #69827, #53014, #96094, #87720, #10438, #62541, #79863, #11550, #104499, #10998, #45170, #105056, #54679, #36747, #44610, #3173, #78752, #27792, #79311, #28903 ),
 ( #88805, #63098, #97195, #12088, #46283, #29984, #63634, #73111, #22112, #4257, #90443, #13168, #6454, #106158, #72566, #98297, #38931, #39506, #47357, #106693, #49026, #73679, #107252, #82041, #14837, #65824, #30546, #40602, #29435, #90995, #97748, #83161, #89353 ),
 ( #38390, #21573, #64176, #5904, #91561, #55782, #21019, #40050, #14285, #55223, #48475, #89897, #31643, #64735, #13720, #98849, #12648, #46826, #5346, #80956, #81484, #4785, #82613, #99387, #56310, #47905, #74231, #99942, #107806, #31093, #22665, #108362, #65275 ),
 ( #23237, #56865, #57436, #108913, #66386, #94298, #50126, #84255, #32205, #83703, #92650, #8092, #75331, #34409, #110562, #102686, #15925, #41705, #59081, #84794, #74772, #7551, #100505, #41156, #109472, #93735, #67484, #23784, #110015, #57973, #85914, #101587, #75865 ) ),
 .UNSPECIFIED., .F., .F., .F.,
 ( 6, 3, 3, 3, 3, 3, 3, 3, 3, 3, 6 ),
 ( 6, 3, 3, 3, 3, 3, 3, 3, 3, 3, 6 ),
 ( 0.000000000000000000, 1.936717162300000128, 3.873434324599999812, 4.841792905749999321, 5.810151486899999718, 7.746868649199999624, 9.683585811500000418, 10.65194439270000082, 11.62030297379999944, 13.55702013610000023, 15.49373729840000102 ),
 ( 0.000000000000000000, 1.936717162300000128, 3.873434324599999812, 4.841792905749999321, 5.810151486899999718, 7.746868649199999624, 9.683585811500000418, 10.65194439270000082, 11.62030297379999944, 13.55702013610000023, 15.49373729840000102 ),
 .UNSPECIFIED. ) ;
#85826=( BOUNDED_CURVE ( )  B_SPLINE_CURVE ( 3, ( #11412, #1921, #55078, #61832 ),
 .UNSPECIFIED., .F., .T. ) 
 B_SPLINE_CURVE_WITH_KNOTS ( ( 4, 4 ),
 ( 5.447131836145489459, 6.315249268837946239 ),
 .UNSPECIFIED. ) 
 CURVE ( )  GEOMETRIC_REPRESENTATION_ITEM ( )  RATIONAL_B_SPLINE_CURVE ( ( 1.000000000000000000, 0.9381775381419560356, 0.9381775381419560356, 1.000000000000000000 ) ) 
 REPRESENTATION_ITEM ( '' )  );
#85835=CARTESIAN_POINT ( 'NONE',  ( 2.288357407604999949, 1517.116049120239950, 203.3334095979369920 ) ) ;
#85859=CARTESIAN_POINT ( 'NONE',  ( -6.546039433425000276, 1516.565291103010168, 211.4147861392469849 ) ) ;
#85862=CARTESIAN_POINT ( 'NONE',  ( 6.563811411605000146, 1514.071098020780028, 201.4679970645470064 ) ) ;
#85869=AXIS2_PLACEMENT_3D ( 'NONE', #33199, #25889, #186 ) ;
#85871=CARTESIAN_POINT ( 'NONE',  ( -2.484577695354999616, 1517.170512887980067, 216.4602579296269766 ) ) ;
#85872=CARTESIAN_POINT ( 'NONE',  ( -7.932506210237777466, 1511.860476874699089, 212.2635995054286582 ) ) ;
#85878=CARTESIAN_POINT ( 'NONE',  ( 2.477373605864999995, 1516.891731298979948, 206.2406231745169976 ) ) ;
#85885=CARTESIAN_POINT ( 'NONE',  ( 7.170545778634999756, 1512.974587999920004, 216.1941441599169877 ) ) ;
#85894=CARTESIAN_POINT ( 'NONE',  ( -5.000083865865000199, 1516.858456333729919, 214.1306941701269864 ) ) ;
#85897=CARTESIAN_POINT ( 'NONE',  ( -7.720817095325030799, 1516.984411380829897, 208.9454551635660380 ) ) ;
#85898=CARTESIAN_POINT ( 'NONE',  ( -2.282915221395000138, 1516.876240617270014, 211.6158662526670184 ) ) ;
#85914=CARTESIAN_POINT ( 'NONE',  ( -6.942354311545000378, 1516.905946377369901, 216.8406094761369900 ) ) ;
#85919=CARTESIAN_POINT ( 'NONE',  ( -6.559168674874999105, 1516.960844870249957, 204.1192525727769862 ) ) ;
#85939=CARTESIAN_POINT ( 'NONE',  ( -4.364199128832369823, 1509.032029411810072, 213.2377089278639914 ) ) ;
#85973=ORIENTED_EDGE ( 'NONE', *, *, #71079, .F. ) ;
#85976=CARTESIAN_POINT ( 'NONE',  ( 7.545803617137186947, 1510.531931299321286, 203.4140010686424773 ) ) ;
#85995=DIRECTION ( 'NONE',  ( -0.02616798426453448984, 0.9993150019883495494, -0.02616798426619649023 ) ) ;
#85997=CARTESIAN_POINT ( 'NONE',  ( 5.009478067315000338, 1516.886345593249871, 213.7343532441369973 ) ) ;
#86004=CARTESIAN_POINT ( 'NONE',  ( 7.712490952985000980, 1516.666407245520077, 204.5049844236870058 ) ) ;
#86011=CARTESIAN_POINT ( 'NONE',  ( -6.445219260712940823, 1513.425324099833460, 216.7494849698516362 ) ) ;
#86019=CARTESIAN_POINT ( 'NONE',  ( -5.771797464315000070, 1516.647618671360078, 211.9976960644470125 ) ) ;
#86023=CARTESIAN_POINT ( 'NONE',  ( -4.042388539304999640, 1517.045004075700035, 208.3857484934819979 ) ) ;
#86027=( BOUNDED_CURVE ( )  B_SPLINE_CURVE ( 3, ( #78420, #52675, #3386, #70054 ),
 .UNSPECIFIED., .F., .T. ) 
 B_SPLINE_CURVE_WITH_KNOTS ( ( 4, 4 ),
 ( 1.997881027491174929E-12, 0.4510268114855899291 ),
 .UNSPECIFIED. ) 
 CURVE ( )  GEOMETRIC_REPRESENTATION_ITEM ( )  RATIONAL_B_SPLINE_CURVE ( ( 1.000000000000000000, 0.9831196230105693212, 0.9831196230105693212, 1.000000000000000000 ) ) 
 REPRESENTATION_ITEM ( '' )  );
#86042=CARTESIAN_POINT ( 'NONE',  ( 7.721907888235000073, 1517.026025493960105, 214.1263215447669950 ) ) ;
#86045=CARTESIAN_POINT ( 'NONE',  ( -5.779627092215000594, 1516.977993847330026, 216.8424961055369806 ) ) ;
#86047=CARTESIAN_POINT ( 'NONE',  ( 7.722102888894769812, 1517.033472268840114, 209.4823235324890334 ) ) ;
#86049=ORIENTED_EDGE ( 'NONE', *, *, #19250, .F. ) ;
#86070=LINE ( 'NONE', #58127, #77084 ) ;
#86080=CARTESIAN_POINT ( 'NONE',  ( -1.856688514214469787, 1516.535411464260051, 201.4127852243740051 ) ) ;
#86126=CARTESIAN_POINT ( 'NONE',  ( 1.715109447055000125, 1516.963431999339946, 209.8570730874349977 ) ) ;
#86135=CARTESIAN_POINT ( 'NONE',  ( -15.31201882530910119, 1512.804203059170050, 222.7675833470860027 ) ) ;
#86142=CARTESIAN_POINT ( 'NONE',  ( -2.297629659184999618, 1516.970035769810011, 208.3868227339359862 ) ) ;
#86159=CARTESIAN_POINT ( 'NONE',  ( -2.492130661305000050, 1516.778761582560037, 205.6761608547170113 ) ) ;
#86204=CARTESIAN_POINT ( 'NONE',  ( 7.334957356574999920, 1517.030858226499959, 213.7381182667970165 ) ) ;
#86238=CARTESIAN_POINT ( 'NONE',  ( 15.18044682235556664, 1511.791180387471059, 197.3654389570463081 ) ) ;
#86241=CARTESIAN_POINT ( 'NONE',  ( -7.002187114500163290, 1516.573284371974751, 211.8084850268393495 ) ) ;
#86245=CARTESIAN_POINT ( 'NONE',  ( -3.462620856235000044, 1516.938330505699923, 206.6435391121569864 ) ) ;
#86259=CARTESIAN_POINT ( 'NONE',  ( -6.546001388695000145, 1516.557392317769882, 210.8318505190270002 ) ) ;
#86291=CARTESIAN_POINT ( 'NONE',  ( 2.289624432225000117, 1517.154223579619838, 202.5582500624169882 ) ) ;
#86292=CARTESIAN_POINT ( 'NONE',  ( 5.781585778145000631, 1516.939646076049939, 209.1093989964429909 ) ) ;
#86295=CARTESIAN_POINT ( 'NONE',  ( 3.208451221193931779, 1511.804171812530058, 217.0732872714422115 ) ) ;
#86307=CARTESIAN_POINT ( 'NONE',  ( -16.66966706706500290, 1516.995662938509895, 194.6788146269670108 ) ) ;
#86328=DIRECTION ( 'NONE',  ( 0.7071067811865474617, -3.909376183068731469E-17, -0.7071067811865474617 ) ) ;
#86329=CARTESIAN_POINT ( 'NONE',  ( -16.51584608446500013, 1514.088841912139969, 223.6140043943670150 ) ) ;
#86333=CARTESIAN_POINT ( 'NONE',  ( 0.7351097711180020200, 1516.977504706749869, 206.6301902066870184 ) ) ;
#86350=CARTESIAN_POINT ( 'NONE',  ( -2.541812797074999963, 1512.177707669779920, 201.4966559065569811 ) ) ;
#86366=CYLINDRICAL_SURFACE ( 'NONE', #82079, 0.9999999999999569233 ) ;
#86376=CARTESIAN_POINT ( 'NONE',  ( -5.513258784733920059, 1508.551704615640119, 216.1343122518819939 ) ) ;
#86385=CARTESIAN_POINT ( 'NONE',  ( 4.032397901875000024, 1516.981965530290154, 203.3362630185569913 ) ) ;
#86400=CARTESIAN_POINT ( 'NONE',  ( -3.487592469735000478, 1508.551704408389924, 214.1089243866569802 ) ) ;
#86409=CARTESIAN_POINT ( 'NONE',  ( -2.476733514145000203, 1516.858326417339867, 211.6155457388669845 ) ) ;
#86412=CARTESIAN_POINT ( 'NONE',  ( 7.014484243095000515, 1513.886778333999928, 201.4788231846570170 ) ) ;
#86420=CARTESIAN_POINT ( 'NONE',  ( 16.59156834624142718, 1513.042027792519093, 197.1096995654986301 ) ) ;
#86422=CARTESIAN_POINT ( 'NONE',  ( -5.004475612664999851, 1517.026025493960105, 216.8437538584669824 ) ) ;
#86430=CARTESIAN_POINT ( 'NONE',  ( -1.136547623115000016, 1516.839862955080207, 206.6438706166370025 ) ) ;
#86435=CARTESIAN_POINT ( 'NONE',  ( -7.096089203739619933, 1508.610128855429821, 202.4734964306379936 ) ) ;
#86440=CARTESIAN_POINT ( 'NONE',  ( -6.003588571597879842, 1511.304111283970087, 201.4516922765099878 ) ) ;
#86448=CARTESIAN_POINT ( 'NONE',  ( 1.711311228545000063, 1516.591755933730155, 214.8926661113670207 ) ) ;
#86452=CARTESIAN_POINT ( 'NONE',  ( 6.951175128784999657, 1517.170721208160103, 211.4121022339570004 ) ) ;
#86467=CARTESIAN_POINT ( 'NONE',  ( 4.999456390405000228, 1516.830644417779922, 204.5005780481670001 ) ) ;
#86478=CARTESIAN_POINT ( 'NONE',  ( 8.126234247455000670, 1514.923664147150021, 215.2485921136969864 ) ) ;
#86525=CARTESIAN_POINT ( 'NONE',  ( 7.542447022002694013, 1510.549724834208519, 203.3709729786484672 ) ) ;
#86544=EDGE_CURVE ( 'NONE', #107607, #21616, #75382, .T. ) ;
#86547=CARTESIAN_POINT ( 'NONE',  ( -2.480187054844999572, 1517.025470194390209, 213.7472054950769973 ) ) ;
#86548=CARTESIAN_POINT ( 'NONE',  ( 2.549111447265000052, 1512.332007210709889, 216.7517165153469989 ) ) ;
#86549=EDGE_CURVE ( 'NONE', #71414, #108462, #80794, .T. ) ;
#86553=CARTESIAN_POINT ( 'NONE',  ( -4.038637500854999729, 1516.734985836460055, 203.3481771172569950 ) ) ;
#86563=CARTESIAN_POINT ( 'NONE',  ( 7.330468880873466375, 1514.095142040203882, 201.0173238986526201 ) ) ;
#86569=CARTESIAN_POINT ( 'NONE',  ( -3.445685115514999897, 1516.778761582560037, 211.6139765934069885 ) ) ;
#86575=CARTESIAN_POINT ( 'NONE',  ( -7.726684725664999753, 1517.208444099459939, 207.9957078235169945 ) ) ;
#86591=CARTESIAN_POINT ( 'NONE',  ( 3.457266605394999637, 1516.691414181030041, 214.8945738789770132 ) ) ;
#86598=ORIENTED_EDGE ( 'NONE', *, *, #95268, .T. ) ;
#86601=CARTESIAN_POINT ( 'NONE',  ( 8.473110443205881026, 1511.778877376279979, 203.0322686476939964 ) ) ;
#86655=( BOUNDED_CURVE ( )  B_SPLINE_CURVE ( 3, ( #99278, #91998, #22554, #49465 ),
 .UNSPECIFIED., .F., .F. ) 
 B_SPLINE_CURVE_WITH_KNOTS ( ( 4, 4 ),
 ( 5.499719231641273964, 7.069826864254338261 ),
 .UNSPECIFIED. ) 
 CURVE ( )  GEOMETRIC_REPRESENTATION_ITEM ( )  RATIONAL_B_SPLINE_CURVE ( ( 1.000000000000000000, 0.8049001529481599748, 0.8049001529481599748, 1.000000000000000000 ) ) 
 REPRESENTATION_ITEM ( '' )  );
#86673=CARTESIAN_POINT ( 'NONE',  ( 6.562094069294999166, 1517.122674412569950, 209.8604508749069737 ) ) ;
#86686=CARTESIAN_POINT ( 'NONE',  ( 7.717505752974999744, 1516.857914730730045, 201.4043401791270185 ) ) ;
#86690=VERTEX_POINT ( 'NONE', #77029 ) ;
#86692=CARTESIAN_POINT ( 'NONE',  ( -6.563915562015000482, 1517.184063036290127, 207.9975562766469750 ) ) ;
#86698=FACE_OUTER_BOUND ( 'NONE', #108525, .T. ) ;
#86702=ADVANCED_FACE ( 'NONE', ( #42308 ), #58575, .T. ) ;
#86709=CARTESIAN_POINT ( 'NONE',  ( -5.011367984924999242, 1516.974592746400049, 205.6720686163770324 ) ) ;
#86731=CARTESIAN_POINT ( 'NONE',  ( 4.621897824414999967, 1516.858533673840157, 213.7337256555570093 ) ) ;
#86761=CARTESIAN_POINT ( 'NONE',  ( 4.621897824414999967, 1516.858533673840157, 213.7337256555570093 ) ) ;
#86773=DIRECTION ( 'NONE',  ( -0.7071067811865475727, -6.078560574715863648E-17, 0.7071067811865475727 ) ) ;
#86786=DIRECTION ( 'NONE',  ( 1.000000000000000000, 0.000000000000000000, 0.000000000000000000 ) ) ;
#86789=ORIENTED_EDGE ( 'NONE', *, *, #95268, .F. ) ;
#86797=CARTESIAN_POINT ( 'NONE',  ( -7.054635634474425210, 1516.562299717372071, 211.6679574601893421 ) ) ;
#86802=CARTESIAN_POINT ( 'NONE',  ( 4.995994787574999485, 1516.665179208830068, 206.6322283937570035 ) ) ;
#86816=CARTESIAN_POINT ( 'NONE',  ( 6.562635822504999439, 1517.111322026010157, 211.9927976380170094 ) ) ;
#86822=ADVANCED_FACE ( 'NONE', ( #87637 ), #85821, .F. ) ;
#86838=CARTESIAN_POINT ( 'NONE',  ( 7.444963621915969831, 1508.731180391410135, 203.6086381548180100 ) ) ;
#86843=CARTESIAN_POINT ( 'NONE',  ( 4.033653264325000265, 1517.028034847769959, 202.5611037067669997 ) ) ;
#86844=CARTESIAN_POINT ( 'NONE',  ( 1.127928333405000094, 1516.989863902050047, 209.1117210464550169 ) ) ;
#86848=ORIENTED_EDGE ( 'NONE', *, *, #108950, .T. ) ;
#86881=CARTESIAN_POINT ( 'NONE',  ( -15.10381384906500202, 1513.853571676670072, 223.9969891008670118 ) ) ;
#86885=CARTESIAN_POINT ( 'NONE',  ( -6.950214971414999887, 1517.129577905929864, 206.2502655435069983 ) ) ;
#86888=CARTESIAN_POINT ( 'NONE',  ( -3.487592467065000257, 1509.038615934239942, 204.6345961781970004 ) ) ;
#86900=EDGE_CURVE ( 'NONE', #21931, #110691, #33291, .T. ) ;
#86907=CARTESIAN_POINT ( 'NONE',  ( -3.049363967234999695, 1511.141271963170084, 201.5540345636269990 ) ) ;
#86939=CARTESIAN_POINT ( 'NONE',  ( -1.133517003235000153, 1516.713079096360161, 204.5117660986770147 ) ) ;
#86952=CARTESIAN_POINT ( 'NONE',  ( -3.487592467601667856, 1508.909942010301620, 213.6124651694365184 ) ) ;
#86960=CARTESIAN_POINT ( 'NONE',  ( -5.772403812434999892, 1516.676340709600026, 212.3853678745870184 ) ) ;
#86963=CARTESIAN_POINT ( 'NONE',  ( 7.750386742905000403, 1513.342361861130030, 201.6522260404070153 ) ) ;
#86970=CARTESIAN_POINT ( 'NONE',  ( -6.865869646824999784, 1512.784460098860109, 216.3356833388470193 ) ) ;
#86971=CARTESIAN_POINT ( 'NONE',  ( 16.06220691697101799, 1512.836811624714528, 198.0093864833502550 ) ) ;
#86981=EDGE_LOOP ( 'NONE', ( #62170, #17115, #8307, #94720 ) ) ;
#86982=CARTESIAN_POINT ( 'NONE',  ( -1.136004312195000088, 1516.815173273089840, 206.2562091229970065 ) ) ;
#86998=CARTESIAN_POINT ( 'NONE',  ( 1.712644716155000024, 1516.636036526019780, 214.1174694231270053 ) ) ;
#87001=CARTESIAN_POINT ( 'NONE',  ( 6.375350481660589708, 1511.068351247050032, 216.5169480941279971 ) ) ;
#87003=CARTESIAN_POINT ( 'NONE',  ( -0.7353365779029981120, 1516.995911393979895, 212.0011643880069698 ) ) ;
#87011=CARTESIAN_POINT ( 'NONE',  ( -7.563688229914999894, 1510.983859056260144, 212.0526840097969909 ) ) ;
#87020=CARTESIAN_POINT ( 'NONE',  ( -0.01289782690309849988, 1516.939723362869927, 204.1155860834069813 ) ) ;
#87040=ORIENTED_EDGE ( 'NONE', *, *, #40920, .T. ) ;
#87062=CARTESIAN_POINT ( 'NONE',  ( 7.160751159672980926, 1516.545310091885540, 206.8877586002222131 ) ) ;
#87071=CARTESIAN_POINT ( 'NONE',  ( 2.484577657225000014, 1517.170512887980067, 201.7834339727070017 ) ) ;
#87079=CARTESIAN_POINT ( 'NONE',  ( -4.730384201341079731, 1508.603735221695615, 205.6342535013503721 ) ) ;
#87103=CARTESIAN_POINT ( 'NONE',  ( -4.030514550714999977, 1516.901952101700090, 213.7446888144170032 ) ) ;
#87104=CARTESIAN_POINT ( 'NONE',  ( 2.766744922505000037, 1511.930588878439949, 216.8060890453470222 ) ) ;
#87105=EDGE_CURVE ( 'NONE', #13404, #100973, #87873, .T. ) ;
#87106=EDGE_LOOP ( 'NONE', ( #56837, #54593, #108267, #7104, #64425, #84670, #11507 ) ) ;
#87110=CARTESIAN_POINT ( 'NONE',  ( 1.705466410464999916, 1517.120861839400050, 204.1076508302870138 ) ) ;
#87115=CARTESIAN_POINT ( 'NONE',  ( 7.329930013194999816, 1516.881930554049859, 201.4037113026670056 ) ) ;
#87118=EDGE_LOOP ( 'NONE', ( #79213, #30217 ) ) ;
#87126=CARTESIAN_POINT ( 'NONE',  ( 2.298369469825000344, 1516.779243033999819, 212.3734572960470075 ) ) ;
#87132=CARTESIAN_POINT ( 'NONE',  ( -3.455495871984999745, 1516.939877939420057, 209.1351200182310208 ) ) ;
#87149=CARTESIAN_POINT ( 'NONE',  ( 0.7553264358530019651, 1516.745833913490060, 214.8974710475970085 ) ) ;
#87152=CARTESIAN_POINT ( 'NONE',  ( -5.004475612664999851, 1517.026025493960105, 216.8437538584669824 ) ) ;
#87188=PLANE ( 'NONE',  #48249 ) ;
#87215=LINE ( 'NONE', #35148, #31854 ) ;
#87228=B_SPLINE_CURVE_WITH_KNOTS ( 'NONE', 3,
 ( #84487, #34637, #69932, #76096, #34083, #95651, #103482, #26787, #77209, #33508 ),
 .UNSPECIFIED., .F., .F.,
 ( 4, 2, 2, 2, 4 ),
 ( 0.000000000000000000, 0.2500000000000000000, 0.5000000000000000000, 0.7500000000000000000, 1.000000000000000000 ),
 .UNSPECIFIED. ) ;
#87235=CARTESIAN_POINT ( 'NONE',  ( -2.868112169295000236, 1516.855632454399938, 209.8795095036720113 ) ) ;
#87243=DIRECTION ( 'NONE',  ( 0.02616798426500960631, -0.9993150019883683122, -0.02616798426500960631 ) ) ;
#87251=CARTESIAN_POINT ( 'NONE',  ( -3.269025173884999802, 1517.026534522949987, 208.0024068424170025 ) ) ;
#87267=CARTESIAN_POINT ( 'NONE',  ( -4.042417815834999928, 1516.904492006980036, 205.6736390534169914 ) ) ;
#87288=CARTESIAN_POINT ( 'NONE',  ( -2.867803664234999772, 1516.994127245590107, 213.7465828294170080 ) ) ;
#87296=CYLINDRICAL_SURFACE ( 'NONE', #93125, 1.000000000000076383 ) ;
#87314=EDGE_CURVE ( 'NONE', #86690, #49508, #82061, .T. ) ;
#87358=CARTESIAN_POINT ( 'NONE',  ( -6.056985123442561125, 1516.746171222724342, 213.5452912592785424 ) ) ;
#87364=CARTESIAN_POINT ( 'NONE',  ( -3.269184946495000244, 1516.940296199220029, 206.8376465686969823 ) ) ;
#87374=VECTOR ( 'NONE', #29849, 1000.000000000000114 ) ;
#87379=CARTESIAN_POINT ( 'NONE',  ( -7.709681306425000713, 1516.559109716219837, 211.9945464874270158 ) ) ;
#87401=CARTESIAN_POINT ( 'NONE',  ( 7.508704985173280555, 1508.884117426920056, 203.6086456676949865 ) ) ;
#87406=CARTESIAN_POINT ( 'NONE',  ( 6.552897366944999469, 1516.858146885269889, 202.5651945608169910 ) ) ;
#87407=CARTESIAN_POINT ( 'NONE',  ( -2.865636847234999784, 1516.815173273089840, 210.2578502442970318 ) ) ;
#87427=CARTESIAN_POINT ( 'NONE',  ( -6.383820993025000057, 1512.069761553100079, 200.7506179303370288 ) ) ;
#87443=FACE_OUTER_BOUND ( 'NONE', #10668, .T. ) ;
#87452=CARTESIAN_POINT ( 'NONE',  ( 3.445685077385000294, 1516.778761582560037, 206.6297153089269898 ) ) ;
#87495=CARTESIAN_POINT ( 'NONE',  ( 3.487592428934999766, 1509.038615934169911, 204.6345961781970004 ) ) ;
#87509=CARTESIAN_POINT ( 'NONE',  ( 0.7369041709050019318, 1517.080322339569875, 204.1102945640870132 ) ) ;
#87512=FACE_OUTER_BOUND ( 'NONE', #89867, .T. ) ;
#87532=CARTESIAN_POINT ( 'NONE',  ( 7.724423394095000894, 1517.122088787240045, 212.5760185856570104 ) ) ;
#87543=CARTESIAN_POINT ( 'NONE',  ( 16.57651862990214653, 1513.029502680801215, 197.1488735994816750 ) ) ;
#87554=CARTESIAN_POINT ( 'NONE',  ( 1.118104729594999958, 1516.965971551240045, 206.8221779662269739 ) ) ;
#87559=CARTESIAN_POINT ( 'NONE',  ( -7.444964753889919074, 1508.731183030150078, 203.6086348057779958 ) ) ;
#87563=CARTESIAN_POINT ( 'NONE',  ( 15.16811419108810099, 1512.319979277499897, 196.2625218158190137 ) ) ;
#87573=CARTESIAN_POINT ( 'NONE',  ( 2.295485501044999932, 1516.651306816259876, 214.1175719399469983 ) ) ;
#87575=CARTESIAN_POINT ( 'NONE',  ( 6.003588533468550814, 1511.304111283970087, 216.7919996258230242 ) ) ;
#87577=CARTESIAN_POINT ( 'NONE',  ( 6.950214933285000285, 1517.129577905929864, 211.9934263588270085 ) ) ;
#87586=CARTESIAN_POINT ( 'NONE',  ( -16.67046855446390197, 1516.551188146170034, 196.0483986024819956 ) ) ;
#87595=CARTESIAN_POINT ( 'NONE',  ( -6.946748557085000719, 1516.983995446890049, 204.1186252050270014 ) ) ;
#87633=DIRECTION ( 'NONE',  ( 1.000000000000000000, 0.000000000000000000, 0.000000000000000000 ) ) ;
#87637=FACE_OUTER_BOUND ( 'NONE', #61344, .T. ) ;
#87641=CARTESIAN_POINT ( 'NONE',  ( 7.883416839195001025, 1512.215430505229961, 206.1881785102070239 ) ) ;
#87668=CARTESIAN_POINT ( 'NONE',  ( -2.868433836634999512, 1517.020727862619879, 214.1341630384669941 ) ) ;
#87669=CARTESIAN_POINT ( 'NONE',  ( 4.805077557904999352, 1510.399296111369949, 216.6702268425969748 ) ) ;
#87676=( BOUNDED_CURVE ( )  B_SPLINE_CURVE ( 3, ( #316, #77011, #34442, #9788 ),
 .UNSPECIFIED., .F., .F. ) 
 B_SPLINE_CURVE_WITH_KNOTS ( ( 4, 4 ),
 ( 4.424456909600460008, 5.579818660903430150 ),
 .UNSPECIFIED. ) 
 CURVE ( )  GEOMETRIC_REPRESENTATION_ITEM ( )  RATIONAL_B_SPLINE_CURVE ( ( 1.000000000000000000, 0.8918208900286694885, 0.8918208900286694885, 1.000000000000000000 ) ) 
 REPRESENTATION_ITEM ( '' )  );
#87679=CARTESIAN_POINT ( 'NONE',  ( 3.255967386345000047, 1516.989560013210166, 204.1101670940770134 ) ) ;
#87685=CARTESIAN_POINT ( 'NONE',  ( 4.364199625590375220, 1509.032014613821502, 205.0059826343180873 ) ) ;
#87689=ORIENTED_EDGE ( 'NONE', *, *, #82218, .F. ) ;
#87691=CARTESIAN_POINT ( 'NONE',  ( -11.90084016216500196, 1512.572572334140204, 216.0729386259769740 ) ) ;
#87697=CARTESIAN_POINT ( 'NONE',  ( 5.012317068235000228, 1517.020727862619879, 211.9902797687369969 ) ) ;
#87702=CARTESIAN_POINT ( 'NONE',  ( 6.949703334655000120, 1517.130100026000036, 209.8609679372960102 ) ) ;
#87720=CARTESIAN_POINT ( 'NONE',  ( 0.01171160595180150039, 1516.939568781210028, 215.6786969668069958 ) ) ;
#87722=LINE ( 'NONE', #36200, #38830 ) ;
#87731=CARTESIAN_POINT ( 'NONE',  ( 8.209489800525210157, 1511.433089852210060, 203.5668989247379841 ) ) ;
#87805=CARTESIAN_POINT ( 'NONE',  ( -6.938478822895000064, 1516.719999691880048, 209.8757167055200057 ) ) ;
#87821=EDGE_LOOP ( 'NONE', ( #36864, #77355, #39320, #2758, #98130, #106275, #107829, #46870, #88488 ) ) ;
#87823=CARTESIAN_POINT ( 'NONE',  ( 1.122033391945000069, 1516.972341476009888, 208.3659064338399673 ) ) ;
#87831=CARTESIAN_POINT ( 'NONE',  ( 8.794242744369535458, 1511.655929346016364, 202.9804211893913362 ) ) ;
#87835=DIRECTION ( 'NONE',  ( -0.02616798426500960631, 0.9993150019883682011, 0.02616798426500960631 ) ) ;
#87840=CARTESIAN_POINT ( 'NONE',  ( 2.282915183265000092, 1516.876240617270014, 206.6278256496669883 ) ) ;
#87857=CARTESIAN_POINT ( 'NONE',  ( -2.868433836634999512, 1517.020727862619879, 214.1341630384669941 ) ) ;
#87873=LINE ( 'NONE', #105771, #96582 ) ;
#87926=CARTESIAN_POINT ( 'NONE',  ( -6.069631065962992622, 1516.744148413207085, 213.5279290861298307 ) ) ;
#87930=CARTESIAN_POINT ( 'NONE',  ( -6.950833568235000648, 1517.156142772249950, 206.6378959915070084 ) ) ;
#87934=CARTESIAN_POINT ( 'NONE',  ( 13.96015159390320726, 1516.660421270692950, 226.2743875082219063 ) ) ;
#87937=CARTESIAN_POINT ( 'NONE',  ( 13.62888593203049936, 1517.051704413129983, 191.9442378289920157 ) ) ;
#87941=CARTESIAN_POINT ( 'NONE',  ( -7.709032175815000443, 1516.534320418310244, 211.6070631641669877 ) ) ;
#87950=CARTESIAN_POINT ( 'NONE',  ( 14.72260980806426112, 1514.508970282057362, 225.4219501776639163 ) ) ;
#87969=ORIENTED_EDGE ( 'NONE', *, *, #77466, .F. ) ;
#87970=CARTESIAN_POINT ( 'NONE',  ( 2.287084270065000258, 1517.068517094990057, 204.1085709707169826 ) ) ;
#87971=CARTESIAN_POINT ( 'NONE',  ( 2.494757998004999866, 1516.937508036699910, 210.8228737931069929 ) ) ;
#87993=CARTESIAN_POINT ( 'NONE',  ( -6.462730663574999923, 1512.074228084999959, 200.5954301961770057 ) ) ;
#87994=ORIENTED_EDGE ( 'NONE', *, *, #8299, .F. ) ;
#88011=CARTESIAN_POINT ( 'NONE',  ( 15.33574361303499956, 1514.703592237370003, 224.8569613759669892 ) ) ;
#88018=CARTESIAN_POINT ( 'NONE',  ( -0.01323705180209850014, 1516.939658295650133, 206.6356258303270010 ) ) ;
#88035=CARTESIAN_POINT ( 'NONE',  ( 5.912224431970154015, 1510.631883404490736, 216.6440474061008388 ) ) ;
#88068=CARTESIAN_POINT ( 'NONE',  ( 4.999456390405000228, 1516.830644417779922, 204.5005780481670001 ) ) ;
#88088=CARTESIAN_POINT ( 'NONE',  ( -4.028307778284999863, 1516.797038924770050, 212.3881954442970255 ) ) ;
#88098=CARTESIAN_POINT ( 'NONE',  ( -8.502796056335000685, 1512.371933174390051, 215.9657241866970026 ) ) ;
#88108=ORIENTED_EDGE ( 'NONE', *, *, #96646, .F. ) ;
#88109=CARTESIAN_POINT ( 'NONE',  ( 2.863787855735000054, 1516.788317650260069, 207.4054531903269947 ) ) ;
#88114=CARTESIAN_POINT ( 'NONE',  ( -6.140086983543329602, 1508.880866264950100, 201.6144240918179946 ) ) ;
#88127=CARTESIAN_POINT ( 'NONE',  ( -7.328049318385000177, 1516.809497469189864, 215.6772390872569929 ) ) ;
#88129=CARTESIAN_POINT ( 'NONE',  ( 6.150612979054229434, 1511.023286695659863, 216.6047038587689997 ) ) ;
#88131=CARTESIAN_POINT ( 'NONE',  ( -5.772403812434999892, 1516.676340709600026, 212.3853678745870184 ) ) ;
#88148=CARTESIAN_POINT ( 'NONE',  ( 3.255340926295000159, 1516.962555622980062, 204.4977466407669908 ) ) ;
#88182=CARTESIAN_POINT ( 'NONE',  ( -14.37690903976499968, 1514.216506490359961, 192.5504339357670176 ) ) ;
#88198=CARTESIAN_POINT ( 'NONE',  ( -8.324963459575000613, 1511.468585915670019, 214.5031579459970033 ) ) ;
#88217=CARTESIAN_POINT ( 'NONE',  ( 5.781490544344999982, 1516.807958722750072, 215.6734893570070142 ) ) ;
#88218=CARTESIAN_POINT ( 'NONE',  ( 2.385772184054999911, 1512.160709093490141, 216.7163506116569920 ) ) ;
#88226=CARTESIAN_POINT ( 'NONE',  ( -0.01306004006829850073, 1516.939762005280045, 204.5032625402269844 ) ) ;
#88230=CARTESIAN_POINT ( 'NONE',  ( 6.554778533645000849, 1516.929962200689943, 201.4024535497269994 ) ) ;
#88239=CARTESIAN_POINT ( 'NONE',  ( 5.786527562335000319, 1517.025653221279981, 212.5728793591970032 ) ) ;
#88244=CARTESIAN_POINT ( 'NONE',  ( -5.775625115495000017, 1516.745833913490060, 209.8771724060850090 ) ) ;
#88258=CARTESIAN_POINT ( 'NONE',  ( -7.326795561505000443, 1516.760434454289907, 214.9020780475669881 ) ) ;
#88267=CARTESIAN_POINT ( 'NONE',  ( 8.640078715520209229, 1511.774605969369986, 202.9607466897689960 ) ) ;
#88275=LINE ( 'NONE', #53592, #5647 ) ;
#88288=CARTESIAN_POINT ( 'NONE',  ( -8.652776130911478347, 1511.435001053830092, 214.5073691320910143 ) ) ;
#88295=CARTESIAN_POINT ( 'NONE',  ( -0.5361381215162029923, 1516.779489719179992, 201.4063938103320197 ) ) ;
#88321=VERTEX_POINT ( 'NONE', #37761 ) ;
#88325=ADVANCED_FACE ( 'NONE', ( #29345 ), #19273, .T. ) ;
#88330=DIRECTION ( 'NONE',  ( -0.01484500364209119690, 0.5669078173028199163, 0.8236474686100957454 ) ) ;
#88340=CARTESIAN_POINT ( 'NONE',  ( -4.031168805994999715, 1516.805675336850072, 209.8787446699039947 ) ) ;
#88343=LINE ( 'NONE', #104029, #48363 ) ;
#88349=CARTESIAN_POINT ( 'NONE',  ( 4.034908559714999399, 1517.068717944079935, 201.7859449365070077 ) ) ;
#88352=B_SPLINE_CURVE_WITH_KNOTS ( 'NONE', 5,
 ( #103098, #42118, #110414, #25283, #85759, #68997 ),
 .UNSPECIFIED., .F., .F.,
 ( 6, 6 ),
 ( 0.000000000000000000, 1.000000000000000000 ),
 .UNSPECIFIED. ) ;
#88356=CARTESIAN_POINT ( 'NONE',  ( -4.625790014595000166, 1517.104192383289956, 208.0004623403669939 ) ) ;
#88372=CARTESIAN_POINT ( 'NONE',  ( 5.771149074885000729, 1516.616791731099966, 206.6334853027970269 ) ) ;
#88390=CARTESIAN_POINT ( 'NONE',  ( 7.719392382375000139, 1516.929962200689943, 215.6766245038770080 ) ) ;
#88396=CARTESIAN_POINT ( 'NONE',  ( 3.873571330434599780, 1517.051704409849890, 202.3168006365660005 ) ) ;
#88407=DIRECTION ( 'NONE',  ( 0.000000000000000000, 1.000000000000000000, -6.123233995736769734E-17 ) ) ;
#88421=CARTESIAN_POINT ( 'NONE',  ( 6.126746143464999683, 1514.923664147150021, 200.9956116846470309 ) ) ;
#88429=CARTESIAN_POINT ( 'NONE',  ( 11.90084012403499969, 1512.572572334140204, 202.1707532763570043 ) ) ;
#88436=LINE ( 'NONE', #2802, #51555 ) ;
#88439=EDGE_CURVE ( 'NONE', #93856, #19743, #23264, .T. ) ;
#88466=CARTESIAN_POINT ( 'NONE',  ( 4.608146781254999880, 1516.677239312369920, 206.8257210811669893 ) ) ;
#88479=CARTESIAN_POINT ( 'NONE',  ( -5.513435596820279727, 1509.038615934079871, 216.6345961782780023 ) ) ;
#88486=CARTESIAN_POINT ( 'NONE',  ( 14.28812837704985661, 1514.188985847965341, 225.6571130645534424 ) ) ;
#88488=ORIENTED_EDGE ( 'NONE', *, *, #71588, .F. ) ;
#88490=VECTOR ( 'NONE', #42366, 999.9999999999998863 ) ;
#88497=FACE_OUTER_BOUND ( 'NONE', #21257, .T. ) ;
#88508=CARTESIAN_POINT ( 'NONE',  ( -5.784008673325000238, 1516.911981270829983, 204.1205073037870079 ) ) ;
#88531=CARTESIAN_POINT ( 'NONE',  ( -6.169347562924999195, 1511.326779185850000, 201.5833654368269947 ) ) ;
#88546=CARTESIAN_POINT ( 'NONE',  ( 11.59188835883499991, 1512.902436350919970, 225.5633015321670030 ) ) ;
#88557=CARTESIAN_POINT ( 'NONE',  ( 3.445201488374999954, 1516.743010792419909, 207.4064848398570291 ) ) ;
#88563=FACE_OUTER_BOUND ( 'NONE', #64183, .T. ) ;
#88615=CARTESIAN_POINT ( 'NONE',  ( -5.784008673325000238, 1516.911981270829983, 204.1205073037870079 ) ) ;
#88618=ADVANCED_FACE ( 'NONE', ( #79648 ), #46049, .T. ) ;
#88619=DIRECTION ( 'NONE',  ( -0.02616798426500960631, -0.9993150019883682011, 0.02616798426500970345 ) ) ;
#88637=CARTESIAN_POINT ( 'NONE',  ( -3.446942109845000157, 1516.842852731759876, 212.3891375753969726 ) ) ;
#88647=CARTESIAN_POINT ( 'NONE',  ( -7.163002535094999956, 1512.132770473890105, 215.9896253418369838 ) ) ;
#88658=CARTESIAN_POINT ( 'NONE',  ( 5.770820141135000192, 1516.591755933730155, 207.4105347035570048 ) ) ;
#88663=FACE_OUTER_BOUND ( 'NONE', #6157, .T. ) ;
#88667=CARTESIAN_POINT ( 'NONE',  ( 14.86137034542100110, 1512.142158944850053, 196.7831344732769878 ) ) ;
#88669=CARTESIAN_POINT ( 'NONE',  ( -6.048292043943890306, 1511.681069547209972, 200.4825432859090029 ) ) ;
#88670=DIRECTION ( 'NONE',  ( -0.4999997527789440399, 0.7071067730516870098, 0.5000002587253580266 ) ) ;
#88675=CARTESIAN_POINT ( 'NONE',  ( 6.555393117025000826, 1516.809497469189864, 216.4498952504870033 ) ) ;
#88677=CARTESIAN_POINT ( 'NONE',  ( 5.890586664718879817, 1511.182265711489890, 216.8011604359759872 ) ) ;
#88679=CARTESIAN_POINT ( 'NONE',  ( -1.702406023195000007, 1516.999105586269934, 212.3918307515370145 ) ) ;
#88697=CARTESIAN_POINT ( 'NONE',  ( -5.784638357945000031, 1516.939574742129935, 204.5080835752170003 ) ) ;
#88729=DIRECTION ( 'NONE',  ( 0.6768489701308448847, 0.6839977328998089190, -0.2720708970484284062 ) ) ;
#88732=CARTESIAN_POINT ( 'NONE',  ( -14.20095109106500075, 1513.466724478469814, 192.5929703138669993 ) ) ;
#88744=ORIENTED_EDGE ( 'NONE', *, *, #85080, .F. ) ;
#88755=( NAMED_UNIT ( * ) PLANE_ANGLE_UNIT ( ) SI_UNIT ( $, .RADIAN. ) );
#88768=CARTESIAN_POINT ( 'NONE',  ( 6.944231748164999551, 1516.882690742909972, 215.6753703478370028 ) ) ;
#88769=CARTESIAN_POINT ( 'NONE',  ( 2.258825551794999775, 1511.942942747529969, 216.7106486523369995 ) ) ;
#88776=CARTESIAN_POINT ( 'NONE',  ( -4.041472511874999896, 1516.858649670339901, 205.0922732913970208 ) ) ;
#88788=CARTESIAN_POINT ( 'NONE',  ( -2.284199401535000007, 1516.940296199220029, 212.3910308785969789 ) ) ;
#88791=CARTESIAN_POINT ( 'NONE',  ( -1.906499758064230099E-08, 1515.051704408389924, 209.1218459511669892 ) ) ;
#88793=CARTESIAN_POINT ( 'NONE',  ( -2.486220139904999904, 1516.939658295650133, 209.1350829839039989 ) ) ;
#88801=LINE ( 'NONE', #3719, #63006 ) ;
#88805=CARTESIAN_POINT ( 'NONE',  ( 7.718763505904999711, 1516.905946377369901, 216.0642002436470079 ) ) ;
#88810=CARTESIAN_POINT ( 'NONE',  ( -5.779603138255000161, 1516.738222552470233, 201.4074744291170020 ) ) ;
#88811=CARTESIAN_POINT ( 'NONE',  ( -16.20447082416500351, 1512.376261820769969, 220.4782031007670184 ) ) ;
#88845=CARTESIAN_POINT ( 'NONE',  ( 0.2440728571770119926, 1517.002586324550066, 201.4005528731310051 ) ) ;
#88849=CARTESIAN_POINT ( 'NONE',  ( 12.62550843869419914, 1512.222316757839963, 224.1785689195619966 ) ) ;
#88862=VECTOR ( 'NONE', #58643, 1000.000000000000114 ) ;
#88863=LINE ( 'NONE', #45228, #20452 ) ;
#88888=CARTESIAN_POINT ( 'NONE',  ( -3.445201526505000000, 1516.743010792419909, 210.8372070624770060 ) ) ;
#88896=CARTESIAN_POINT ( 'NONE',  ( -7.717505791104999346, 1516.857914730730045, 201.4043401791270185 ) ) ;
#88907=CARTESIAN_POINT ( 'NONE',  ( 8.748307446421703659, 1511.491070485854152, 203.4049457530220195 ) ) ;
#88910=AXIS2_PLACEMENT_3D ( 'NONE', #53565, #36739, #96655 ) ;
#88916=CARTESIAN_POINT ( 'NONE',  ( -2.880592967115000125, 1516.859514182039902, 206.2568738160869941 ) ) ;
#88931=CARTESIAN_POINT ( 'NONE',  ( -1.906509838889290056E-08, 1508.551704408389924, 204.1347675157070114 ) ) ;
#88932=CARTESIAN_POINT ( 'NONE',  ( 6.945490048805000427, 1516.932669162149978, 214.9002185338470099 ) ) ;
#88933=DIRECTION ( 'NONE',  ( 0.000000000000000000, 6.123233995736769734E-17, 1.000000000000000000 ) ) ;
#88937=CARTESIAN_POINT ( 'NONE',  ( 4.075310198389409777, 1517.051704406860154, 202.0559764476869873 ) ) ;
#88981=CARTESIAN_POINT ( 'NONE',  ( -3.487592469735000478, 1508.551704408389924, 214.1089243866569802 ) ) ;
#89000=CARTESIAN_POINT ( 'NONE',  ( 5.770820141135000192, 1516.591755933730155, 207.4105347035570048 ) ) ;
#89020=CARTESIAN_POINT ( 'NONE',  ( 14.81823676263572587, 1514.585431681391583, 225.3567438282504440 ) ) ;
#89040=CARTESIAN_POINT ( 'NONE',  ( 2.286446325635000054, 1517.042661899400173, 204.4961520670869959 ) ) ;
#89043=EDGE_CURVE ( 'NONE', #104774, #76367, #30545, .T. ) ;
#89065=CARTESIAN_POINT ( 'NONE',  ( -6.277682590474999991, 1511.927085655870087, 201.2403123398769935 ) ) ;
#89080=CARTESIAN_POINT ( 'NONE',  ( 12.28497684303499859, 1512.406775501100128, 225.6610851038670091 ) ) ;
#89087=CARTESIAN_POINT ( 'NONE',  ( 12.07722019555130544, 1511.957228877181251, 223.9708055708832148 ) ) ;
#89090=CARTESIAN_POINT ( 'NONE',  ( -5.788436372295000076, 1517.116049120239950, 206.8334885244969712 ) ) ;
#89134=CARTESIAN_POINT ( 'NONE',  ( 3.487592430751666583, 1508.603735221695615, 204.3914617688909345 ) ) ;
#89148=CARTESIAN_POINT ( 'NONE',  ( 6.937338745574999521, 1516.706638732659940, 204.5037262658370025 ) ) ;
#89163=ADVANCED_FACE ( 'NONE', ( #2270 ), #52649, .T. ) ;
#89178=CARTESIAN_POINT ( 'NONE',  ( -6.166911790614999944, 1513.656171171930055, 216.7076464020170192 ) ) ;
#89179=CARTESIAN_POINT ( 'NONE',  ( 16.01537988097770437, 1514.821748395666646, 194.0245274743359118 ) ) ;
#89186=CARTESIAN_POINT ( 'NONE',  ( -4.427981762014999489, 1510.423579818969984, 201.5728291684769999 ) ) ;
#89190=CARTESIAN_POINT ( 'NONE',  ( -2.882326017515000061, 1516.969638403840008, 207.4201161117570109 ) ) ;
#89202=CARTESIAN_POINT ( 'NONE',  ( -5.567226385628840646, 1511.487400615810202, 200.5687758574929944 ) ) ;
#89208=CARTESIAN_POINT ( 'NONE',  ( 4.617490466775000080, 1516.685667699390024, 216.4467608883869900 ) ) ;
#89212=CARTESIAN_POINT ( 'NONE',  ( 5.972112752736340013, 1511.562335007999991, 217.9146188711339960 ) ) ;
#89214=CARTESIAN_POINT ( 'NONE',  ( 2.448631922079805179, 1516.534705479064542, 216.8308881910905370 ) ) ;
#89215=CARTESIAN_POINT ( 'NONE',  ( -3.446329813785000251, 1516.812046502680005, 212.0014881234369852 ) ) ;
#89231=ORIENTED_EDGE ( 'NONE', *, *, #36766, .T. ) ;
#89232=CARTESIAN_POINT ( 'NONE',  ( -0.7564342523539989704, 1516.783665406140017, 204.5091745923169810 ) ) ;
#89259=CARTESIAN_POINT ( 'NONE',  ( 7.951441301218317825, 1511.804171812503228, 205.9133947108762186 ) ) ;
#89269=CARTESIAN_POINT ( 'NONE',  ( -12.30406198576499932, 1511.972232048389969, 194.0466686572669914 ) ) ;
#89273=CARTESIAN_POINT ( 'NONE',  ( -7.717505791104999346, 1516.857914730730045, 201.4043401791270185 ) ) ;
#89277=CARTESIAN_POINT ( 'NONE',  ( 7.594504641424999924, 1512.160709093490141, 206.7360737480470050 ) ) ;
#89283=VERTEX_POINT ( 'NONE', #27779 ) ;
#89288=CARTESIAN_POINT ( 'NONE',  ( -7.618992712005001167, 1511.297452611760036, 212.2897357890169872 ) ) ;
#89296=SURFACE_STYLE_FILL_AREA ( #46220 ) ;
#89306=VERTEX_POINT ( 'NONE', #47343 ) ;
#89311=CARTESIAN_POINT ( 'NONE',  ( -6.937965698444999774, 1516.732530461250008, 214.1275461716370216 ) ) ;
#89317=CARTESIAN_POINT ( 'NONE',  ( 1.704794803334999997, 1517.096587378560116, 204.4952540647470016 ) ) ;
#89332=CARTESIAN_POINT ( 'NONE',  ( -0.7356989727169980231, 1517.020847257979995, 212.5827121409169820 ) ) ;
#89338=CARTESIAN_POINT ( 'NONE',  ( -7.711493580499960032, 1516.628317670949855, 210.2679642827060036 ) ) ;
#89339=CARTESIAN_POINT ( 'NONE',  ( -0.7468175536419978666, 1517.006509894990131, 209.1289748073840258 ) ) ;
#89353=CARTESIAN_POINT ( 'NONE',  ( -7.716252091104999877, 1516.810037859429940, 216.0641906620670056 ) ) ;
#89358=CARTESIAN_POINT ( 'NONE',  ( -6.555393155154999540, 1516.809497469189864, 201.7937966518470034 ) ) ;
#89379=CARTESIAN_POINT ( 'NONE',  ( -4.487249792034999629, 1509.038615934239942, 209.1727295022979831 ) ) ;
#89390=CARTESIAN_POINT ( 'NONE',  ( -3.487592469735000478, 1508.551704408389924, 214.1089243866569802 ) ) ;
#89400=CARTESIAN_POINT ( 'NONE',  ( 13.13649027217820020, 1512.464953430860078, 224.3787356123430072 ) ) ;
#89440=CARTESIAN_POINT ( 'NONE',  ( 7.726331925474999807, 1517.194972660189933, 211.4133602680070112 ) ) ;
#89444=VECTOR ( 'NONE', #46457, 1000.000000000000114 ) ;
#89447=CARTESIAN_POINT ( 'NONE',  ( -2.873329398885000163, 1516.572193931679976, 201.7997408644770019 ) ) ;
#89461=VECTOR ( 'NONE', #39526, 1000.000000000000000 ) ;
#89468=CARTESIAN_POINT ( 'NONE',  ( 7.669726159795000164, 1510.984078637139874, 204.3009007237270112 ) ) ;
#89469=CARTESIAN_POINT ( 'NONE',  ( 2.864326087304999824, 1516.826109302209943, 206.6287721023469999 ) ) ;
#89473=VERTEX_POINT ( 'NONE', #69128 ) ;
#89486=CARTESIAN_POINT ( 'NONE',  ( -6.551643424905000401, 1516.807958722750072, 214.9033365145770063 ) ) ;
#89488=CARTESIAN_POINT ( 'NONE',  ( 7.708967986252149629, 1516.531870573939841, 207.1906748737330020 ) ) ;
#89541=ORIENTED_EDGE ( 'NONE', *, *, #73025, .T. ) ;
#89555=CARTESIAN_POINT ( 'NONE',  ( 0.7374508827770021036, 1516.978425811520083, 207.9881927911069965 ) ) ;
#89567=CARTESIAN_POINT ( 'NONE',  ( -5.513435592011666664, 1508.603735221805437, 216.3914617690659554 ) ) ;
#89576=VERTEX_POINT ( 'NONE', #29305 ) ;
#89591=CARTESIAN_POINT ( 'NONE',  ( 5.775236792744999903, 1516.804776704140068, 204.1142572851869943 ) ) ;
#89592=ORIENTED_EDGE ( 'NONE', *, *, #91338, .F. ) ;
#89612=CARTESIAN_POINT ( 'NONE',  ( -7.643022785574999034, 1513.886778333989923, 202.1073616889970026 ) ) ;
#89621=VERTEX_POINT ( 'NONE', #70808 ) ;
#89627=CARTESIAN_POINT ( 'NONE',  ( 15.36700631263500050, 1514.600163677630007, 224.7419540494670116 ) ) ;
#89633=EDGE_CURVE ( 'NONE', #2864, #42578, #45816, .T. ) ;
#89635=CARTESIAN_POINT ( 'NONE',  ( 2.282301578035000222, 1516.836638729160086, 207.4044134838369757 ) ) ;
#89692=CARTESIAN_POINT ( 'NONE',  ( -7.723480117524999855, 1517.086065052259983, 205.0863097070169943 ) ) ;
#89694=ORIENTED_EDGE ( 'NONE', *, *, #25752, .F. ) ;
#89706=CARTESIAN_POINT ( 'NONE',  ( -2.282301616165000269, 1516.836638729160086, 210.8392784184970026 ) ) ;
#89721=ORIENTED_EDGE ( 'NONE', *, *, #68157, .T. ) ;
#89727=CARTESIAN_POINT ( 'NONE',  ( -15.20279581456499862, 1516.814170398969964, 193.2119433744669834 ) ) ;
#89738=CARTESIAN_POINT ( 'NONE',  ( 4.995623452895000760, 1516.636036526019780, 207.4092012159470073 ) ) ;
#89749=CARTESIAN_POINT ( 'NONE',  ( -5.745732830054069318, 1511.535603804869879, 200.5210532146669777 ) ) ;
#89756=CARTESIAN_POINT ( 'NONE',  ( 3.455377977254999955, 1516.627618683580067, 216.0573038954169931 ) ) ;
#89760=CARTESIAN_POINT ( 'NONE',  ( 5.010422963235000360, 1516.929569650079884, 213.1529883219070030 ) ) ;
#89778=CARTESIAN_POINT ( 'NONE',  ( -5.785582951674999919, 1516.981965530290154, 205.0894480302270040 ) ) ;
#89784=CARTESIAN_POINT ( 'NONE',  ( -1.906499846882070084E-08, 1517.051704408389924, 209.1218459511669892 ) ) ;
#89806=CARTESIAN_POINT ( 'NONE',  ( 7.902600983353781139, 1511.989325512384539, 206.0920258474665161 ) ) ;
#89807=ADVANCED_FACE ( 'NONE', ( #45862 ), #87296, .F. ) ;
#89817=CARTESIAN_POINT ( 'NONE',  ( -11.40944913866499988, 1511.843510977570077, 193.5978051729669858 ) ) ;
#89820=EDGE_CURVE ( 'NONE', #36699, #108962, #35310, .T. ) ;
#89821=CARTESIAN_POINT ( 'NONE',  ( 2.871580388595000422, 1517.129577905929864, 202.1716309988170224 ) ) ;
#89831=EDGE_LOOP ( 'NONE', ( #86598, #48167, #35659, #44563 ) ) ;
#89832=CARTESIAN_POINT ( 'NONE',  ( 8.359890770754999423, 1517.051704408389924, 212.3516885548369828 ) ) ;
#89859=CARTESIAN_POINT ( 'NONE',  ( 3.457266605394999637, 1516.691414181030041, 214.8945738789770132 ) ) ;
#89866=CARTESIAN_POINT ( 'NONE',  ( 4.030514512585000375, 1516.901952101700090, 204.4990030879170320 ) ) ;
#89867=EDGE_LOOP ( 'NONE', ( #14873, #6780, #31682, #12467, #89694, #11288, #96202, #27229, #70339 ) ) ;
#89878=CARTESIAN_POINT ( 'NONE',  ( -3.253141175365000137, 1516.858171774179937, 212.3894494859370070 ) ) ;
#89883=CARTESIAN_POINT ( 'NONE',  ( -7.709221527022020126, 1516.541553964140121, 211.7112638145030132 ) ) ;
#89884=CARTESIAN_POINT ( 'NONE',  ( -1.700259714084999763, 1516.898441858519845, 210.8400494336869997 ) ) ;
#89897=CARTESIAN_POINT ( 'NONE',  ( 2.485845998894999909, 1516.545806094630279, 216.4433018439569878 ) ) ;
#89902=CARTESIAN_POINT ( 'NONE',  ( 2.290886266485000267, 1517.184383877180153, 201.7830921018669983 ) ) ;
#89903=CARTESIAN_POINT ( 'NONE',  ( -15.25940260716499886, 1512.044075975079977, 221.6912987172670171 ) ) ;
#89907=CARTESIAN_POINT ( 'NONE',  ( 7.554100936931009258, 1510.639750819960000, 203.5987926776629706 ) ) ;
#89935=CARTESIAN_POINT ( 'NONE',  ( -0.7166913390183430321, 1516.729697371089969, 201.4076976688539844 ) ) ;
#89980=VERTEX_POINT ( 'NONE', #32496 ) ;
#89982=CARTESIAN_POINT ( 'NONE',  ( 6.564578685215000320, 1517.199196846569976, 210.8299485595169926 ) ) ;
#89985=CARTESIAN_POINT ( 'NONE',  ( -6.933879441005000643, 1516.560253536979872, 211.6083207129769903 ) ) ;
#89992=CARTESIAN_POINT ( 'NONE',  ( -7.718134667564999774, 1516.881930554049859, 201.7919159189069944 ) ) ;
#90005=CARTESIAN_POINT ( 'NONE',  ( -1.700259714084999763, 1516.898441858519845, 210.8400494336869997 ) ) ;
#90009=CARTESIAN_POINT ( 'NONE',  ( 8.652776102125001145, 1511.435001052829875, 203.7363227704070141 ) ) ;
#90010=CARTESIAN_POINT ( 'NONE',  ( -5.012317106364999830, 1517.020727862619879, 206.2534121335969814 ) ) ;
#90014=EDGE_LOOP ( 'NONE', ( #24894, #68953, #25919, #33983, #61242, #33260 ) ) ;
#90025=CARTESIAN_POINT ( 'NONE',  ( 6.557909882634999299, 1516.908489800550115, 214.8995913655070069 ) ) ;
#90026=EDGE_LOOP ( 'NONE', ( #70899, #69591, #47836, #47744 ) ) ;
#90027=CARTESIAN_POINT ( 'NONE',  ( 7.709003288537009446, 1516.533218713809902, 207.2190329785249787 ) ) ;
#90050=CARTESIAN_POINT ( 'NONE',  ( -4.495269895834999474, 1510.967342883699985, 201.4658172643670184 ) ) ;
#90083=CARTESIAN_POINT ( 'NONE',  ( -5.649719788644999241, 1514.216922324319739, 217.7705376956769783 ) ) ;
#90094=CARTESIAN_POINT ( 'NONE',  ( 2.282301578035000222, 1516.836638729160086, 207.4044134838369757 ) ) ;
#90115=CARTESIAN_POINT ( 'NONE',  ( 13.59249326269330638, 1513.749562428420177, 225.8724118782147627 ) ) ;
#90123=CARTESIAN_POINT ( 'NONE',  ( 4.832613787568170061, 1508.551704408610021, 205.6342609684550098 ) ) ;
#90131=CARTESIAN_POINT ( 'NONE',  ( -2.295485539174999978, 1516.651306816259876, 204.1261199623870368 ) ) ;
#90132=ORIENTED_EDGE ( 'NONE', *, *, #219, .T. ) ;
#90167=CARTESIAN_POINT ( 'NONE',  ( 14.87514313063500104, 1513.853571676670072, 224.2256597811669963 ) ) ;
#90173=CARTESIAN_POINT ( 'NONE',  ( -1.137296688934999800, 1516.908147884120126, 207.4199954749970232 ) ) ;
#90215=SURFACE_STYLE_FILL_AREA ( #108125 ) ;
#90231=CARTESIAN_POINT ( 'NONE',  ( 2.866857893004999713, 1516.951766529250108, 205.0784797119270024 ) ) ;
#90248=CARTESIAN_POINT ( 'NONE',  ( -1.700259714084999763, 1516.898441858519845, 210.8400494336869997 ) ) ;
#90275=CARTESIAN_POINT ( 'NONE',  ( 2.291514297774999598, 1517.194972660189933, 201.3955140066269962 ) ) ;
#90276=CARTESIAN_POINT ( 'NONE',  ( 5.775625077365000415, 1516.745833913490060, 208.3665194962490261 ) ) ;
#90287=CARTESIAN_POINT ( 'NONE',  ( -5.803572394938940171, 1510.929912129060085, 201.5255253609520025 ) ) ;
#90289=CARTESIAN_POINT ( 'NONE',  ( -5.857434716771726890, 1510.600498191483894, 201.5911444504724841 ) ) ;
#90294=CARTESIAN_POINT ( 'NONE',  ( -1.708102627415000185, 1517.199196846569976, 215.6864246554469844 ) ) ;
#90298=CARTESIAN_POINT ( 'NONE',  ( 0.7572979362240020995, 1516.829948096479939, 212.5714934102470011 ) ) ;
#90318=CARTESIAN_POINT ( 'NONE',  ( -7.722536802824999214, 1517.050041317280147, 204.5049460973469877 ) ) ;
#90344=CARTESIAN_POINT ( 'NONE',  ( 8.392690843783809029, 1511.399183828317064, 204.5144203855979583 ) ) ;
#90356=CARTESIAN_POINT ( 'NONE',  ( -14.56792387476500039, 1513.484013041540038, 193.8069907496669657 ) ) ;
#90359=CARTESIAN_POINT ( 'NONE',  ( -1.130002532395000037, 1516.621991115350056, 202.1860446705670142 ) ) ;
#90373=DIRECTION ( 'NONE',  ( 0.4999999999998399058, 0.7071067811867739472, -0.4999999999998399058 ) ) ;
#90383=CARTESIAN_POINT ( 'NONE',  ( 8.526415735925001016, 1512.074228085009963, 202.6591153066570143 ) ) ;
#90394=CARTESIAN_POINT ( 'NONE',  ( -6.552897405075000847, 1516.858146885269889, 215.6784973415170157 ) ) ;
#90403=CARTESIAN_POINT ( 'NONE',  ( -5.011367984924999242, 1516.974592746400049, 205.6720686163770324 ) ) ;
#90405=CARTESIAN_POINT ( 'NONE',  ( 2.292217010694999946, 1516.941178807709775, 209.1086494233340147 ) ) ;
#90411=VERTEX_POINT ( 'NONE', #33569 ) ;
#90417=CARTESIAN_POINT ( 'NONE',  ( 3.461047291624999911, 1516.858765657450249, 212.5691103191969944 ) ) ;
#90424=CARTESIAN_POINT ( 'NONE',  ( -7.709487050242899819, 1516.551695078709827, 211.8815864275139802 ) ) ;
#90426=CARTESIAN_POINT ( 'NONE',  ( -6.933587693644999383, 1516.542957540330008, 210.8312046333570038 ) ) ;
#90439=CARTESIAN_POINT ( 'NONE',  ( 7.599227146160510316, 1512.341036968809931, 206.8869228877400133 ) ) ;
#90442=EDGE_CURVE ( 'NONE', #36663, #86690, #71237, .T. ) ;
#90443=CARTESIAN_POINT ( 'NONE',  ( 2.873958851594999864, 1516.588006113850042, 216.0563744999969913 ) ) ;
#90448=CARTESIAN_POINT ( 'NONE',  ( -5.005071046424999892, 1516.710692850270107, 201.7963041449669959 ) ) ;
#90449=CARTESIAN_POINT ( 'NONE',  ( -15.18044686046500047, 1511.791180387469922, 220.8782529452670076 ) ) ;
#90489=CARTESIAN_POINT ( 'NONE',  ( 12.85932411630730066, 1512.319979277509901, 224.2899601613300149 ) ) ;
#90493=CARTESIAN_POINT ( 'NONE',  ( -7.722580352405000070, 1517.051704408389924, 207.5526846776770071 ) ) ;
#90503=CARTESIAN_POINT ( 'NONE',  ( -14.72576942166499947, 1512.123542805230272, 221.3115653187670091 ) ) ;
#90529=CARTESIAN_POINT ( 'NONE',  ( -4.608021707265000266, 1516.660388280709867, 210.8351633799069873 ) ) ;
#90532=CARTESIAN_POINT ( 'NONE',  ( -3.446942109845000157, 1516.842852731759876, 212.3891375753969726 ) ) ;
#90538=CARTESIAN_POINT ( 'NONE',  ( 1.710012720495000194, 1517.232977404109988, 201.3945188173769907 ) ) ;
#90545=EDGE_CURVE ( 'NONE', #100973, #71414, #86070, .T. ) ;
#90548=EDGE_LOOP ( 'NONE', ( #26025, #15897, #79408 ) ) ;
#90554=CARTESIAN_POINT ( 'NONE',  ( 1.135898785685000023, 1516.958737650239982, 210.2414381519470226 ) ) ;
#90561=CARTESIAN_POINT ( 'NONE',  ( 6.548200587644999793, 1516.632821972880038, 207.9912384682270101 ) ) ;
#90576=ADVANCED_FACE ( 'NONE', ( #95025 ), #97225, .T. ) ;
#90578=CARTESIAN_POINT ( 'NONE',  ( 2.485845998894999909, 1516.545806094630279, 216.4433018439569878 ) ) ;
#90580=CARTESIAN_POINT ( 'NONE',  ( 7.716234671763589681, 1516.809374097749924, 208.6912322278259921 ) ) ;
#90597=ORIENTED_EDGE ( 'NONE', *, *, #12098, .F. ) ;
#90611=CARTESIAN_POINT ( 'NONE',  ( -5.385523200472070116, 1511.435001055929888, 200.4690698413500058 ) ) ;
#90619=ORIENTED_EDGE ( 'NONE', *, *, #14901, .T. ) ;
#90645=CARTESIAN_POINT ( 'NONE',  ( -8.602963518122210829, 1511.535621886429908, 214.8679164923370024 ) ) ;
#90649=CARTESIAN_POINT ( 'NONE',  ( -4.044319925355000400, 1517.073005577650065, 208.0013022344469960 ) ) ;
#90654=VECTOR ( 'NONE', #70099, 1000.000000000000114 ) ;
#90678=CARTESIAN_POINT ( 'NONE',  ( 4.115882519823130359, 1509.032029208890208, 204.7576547855990157 ) ) ;
#90687=CARTESIAN_POINT ( 'NONE',  ( -7.335901033725000353, 1517.068717944079935, 205.0869373723870126 ) ) ;
#90696=CARTESIAN_POINT ( 'NONE',  ( -13.58541698226610173, 1512.759354980439866, 193.8094473928580044 ) ) ;
#90714=DIRECTION ( 'NONE',  ( 4.336808689942001466E-16, -0.02617694830786544691, 0.9996573249755575929 ) ) ;
#90731=CARTESIAN_POINT ( 'NONE',  ( 10.96771871715767155, 1512.594959757391052, 225.0393121556896290 ) ) ;
#90737=ADVANCED_FACE ( 'NONE', ( #8117 ), #3694, .T. ) ;
#90783=CARTESIAN_POINT ( 'NONE',  ( -3.864359895900485231, 1511.505225070758115, 200.9696564112188923 ) ) ;
#90791=CARTESIAN_POINT ( 'NONE',  ( 1.702754371344999962, 1517.014196759610059, 205.6580786742169948 ) ) ;
#90807=CARTESIAN_POINT ( 'NONE',  ( 6.563915523884999992, 1517.184063036290127, 210.2461356256870033 ) ) ;
#90819=CARTESIAN_POINT ( 'NONE',  ( -6.126746181595000174, 1514.923664147150021, 217.2480802176870043 ) ) ;
#90820=CARTESIAN_POINT ( 'NONE',  ( 16.58691039599694150, 1514.105081323590866, 194.9569398562394724 ) ) ;
#90832=CARTESIAN_POINT ( 'NONE',  ( 4.487249753806469954, 1509.038615938009798, 205.6342535008409982 ) ) ;
#90833=CARTESIAN_POINT ( 'NONE',  ( 1.704170714124999986, 1516.927039499179955, 208.3639196453299860 ) ) ;
#90845=CARTESIAN_POINT ( 'NONE',  ( -6.123056464990721537, 1510.784366232218872, 201.6446126835382131 ) ) ;
#90850=CARTESIAN_POINT ( 'NONE',  ( 1.129386202275000084, 1516.613712827999962, 216.4452363774470030 ) ) ;
#90856=CARTESIAN_POINT ( 'NONE',  ( 2.428364288097684565, 1516.533847659095727, 216.8308657282840954 ) ) ;
#90857=CARTESIAN_POINT ( 'NONE',  ( 5.011367946795000528, 1516.974592746400049, 212.5716232859570027 ) ) ;
#90860=CARTESIAN_POINT ( 'NONE',  ( 3.487585849221220169, 1508.611352722540005, 213.7999951158270164 ) ) ;
#90875=CARTESIAN_POINT ( 'NONE',  ( -0.01322039564809850132, 1516.939819969850078, 205.0847949345169923 ) ) ;
#90907=CARTESIAN_POINT ( 'NONE',  ( 8.133924938042731867, 1511.520894735510410, 205.3152396615298585 ) ) ;
#90917=CARTESIAN_POINT ( 'NONE',  ( -15.36700635076499921, 1514.600163677630007, 193.5017378528669667 ) ) ;
#90921=CARTESIAN_POINT ( 'NONE',  ( -2.291676311554999845, 1516.534976163889951, 201.8006522243570089 ) ) ;
#90924=CARTESIAN_POINT ( 'NONE',  ( 15.47073870303499987, 1511.939906524110256, 196.6289149681670096 ) ) ;
#90933=CARTESIAN_POINT ( 'NONE',  ( -5.779603138333690993, 1516.738222555248967, 201.4074744776068258 ) ) ;
#90936=CARTESIAN_POINT ( 'NONE',  ( -7.891777524685001488, 1512.314860029340025, 212.0638756013070179 ) ) ;
#90956=CARTESIAN_POINT ( 'NONE',  ( -4.034280953785000179, 1517.049325831759916, 216.0701676760970145 ) ) ;
#90963=CARTESIAN_POINT ( 'NONE',  ( 6.935133380425000382, 1516.613881697390070, 205.8602099992770036 ) ) ;
#90965=CARTESIAN_POINT ( 'NONE',  ( -4.618583430005000601, 1516.939762005280045, 209.1349059721700030 ) ) ;
#90968=CARTESIAN_POINT ( 'NONE',  ( 6.479185118354999773, 1511.503799556579906, 216.5023728028170069 ) ) ;
#90975=VECTOR ( 'NONE', #50222, 1000.000000000000000 ) ;
#90977=CARTESIAN_POINT ( 'NONE',  ( -7.323974644434999348, 1516.647924054489977, 213.1579656147470132 ) ) ;
#90982=CARTESIAN_POINT ( 'NONE',  ( 7.726331925474999807, 1517.194972660189933, 211.4133602680070112 ) ) ;
#90995=CARTESIAN_POINT ( 'NONE',  ( -6.553524415734999664, 1516.882690742909972, 216.0660777183969969 ) ) ;
#91000=CARTESIAN_POINT ( 'NONE',  ( 4.616272296565000488, 1517.030858226499959, 201.7868885755270014 ) ) ;
#91028=CARTESIAN_POINT ( 'NONE',  ( -4.429773623542629934, 1508.551704408389924, 213.9240755698690180 ) ) ;
#91038=CARTESIAN_POINT ( 'NONE',  ( 13.77006422079479897, 1512.900351074060154, 224.4275834823730236 ) ) ;
#91080=CARTESIAN_POINT ( 'NONE',  ( 1.718203463455000080, 1516.898441858519845, 210.8221056461869978 ) ) ;
#91083=CARTESIAN_POINT ( 'NONE',  ( 7.336844642415000450, 1517.106845464700200, 212.5753907958570039 ) ) ;
#91093=CARTESIAN_POINT ( 'NONE',  ( -7.331812124104999384, 1516.906641539930206, 202.5676945058570197 ) ) ;
#91112=CARTESIAN_POINT ( 'NONE',  ( 3.269025135755000200, 1517.026534522949987, 210.2412850599169758 ) ) ;
#91117=CARTESIAN_POINT ( 'NONE',  ( 7.656028667734999793, 1510.967342883699985, 204.6265760743969793 ) ) ;
#91118=CARTESIAN_POINT ( 'NONE',  ( 0.7350231981660010350, 1516.970035769810011, 206.8242163110469960 ) ) ;
#91122=CARTESIAN_POINT ( 'NONE',  ( -0.2572001039731363070, 1516.857224341873234, 201.6176683814753403 ) ) ;
#91127=CARTESIAN_POINT ( 'NONE',  ( -1.906499846882070084E-08, 1509.038615934239942, 201.6090957241369779 ) ) ;
#91136=CARTESIAN_POINT ( 'NONE',  ( 0.01073129396420149928, 1516.939491476980038, 216.4539099096770087 ) ) ;
#91138=CARTESIAN_POINT ( 'NONE',  ( 7.714513390629210932, 1516.743641023210103, 208.4557674029649945 ) ) ;
#91161=EDGE_CURVE ( 'NONE', #89473, #96332, #34710, .T. ) ;
#91167=CARTESIAN_POINT ( 'NONE',  ( -4.427981762014999489, 1510.423579818969984, 201.5728291684769999 ) ) ;
#91209=CARTESIAN_POINT ( 'NONE',  ( -7.339749373344999661, 1517.224900789629828, 207.4124613591469881 ) ) ;
#91213=B_SPLINE_SURFACE_WITH_KNOTS ( 'NONE', 5, 5, ( 
 ( #47851, #108855, #100991, #6402, #41660, #48976, #83108, #81985, #83648 ),
 ( #75816, #90383, #48421, #6943, #92595, #64679, #98796, #5293, #39451 ),
 ( #65220, #14232, #82564, #51727, #16421, #77475, #69091, #52836, #8592 ),
 ( #42764, #102634, #76924, #76363, #35461, #25935, #61258, #69651, #78013 ),
 ( #43870, #86963, #110512, #60131, #233, #52287, #59572, #94816, #1320 ),
 ( #776, #33794, #103772, #86412, #34905, #34360, #18093, #17524, #50614 ),
 ( #10254, #18637, #102100, #44430, #85862, #93152, #43327, #27075, #9163 ),
 ( #94250, #103192, #84746, #9702, #26497, #78574, #59027, #16966, #60693 ),
 ( #33245, #95373, #67435, #8044, #101533, #24822, #42212, #67988, #25380 ) ),
 .UNSPECIFIED., .F., .F., .F.,
 ( 6, 3, 6 ),
 ( 6, 3, 6 ),
 ( 3.580107477810000383, 6.558749095569999632, 9.700153431689999550 ),
 ( 0.000000000000000000, 0.5000000000000000000, 1.000000000000000000 ),
 .UNSPECIFIED. ) ;
#91221=CARTESIAN_POINT ( 'NONE',  ( -15.05672298745219884, 1512.222316757829958, 221.7473544089129973 ) ) ;
#91227=DIRECTION ( 'NONE',  ( 0.000000000000000000, -1.000000000000000000, 6.123233995736769734E-17 ) ) ;
#91239=FACE_OUTER_BOUND ( 'NONE', #60056, .T. ) ;
#91240=CARTESIAN_POINT ( 'NONE',  ( -9.638115897709079505, 1516.551188146539971, 203.7504991310609910 ) ) ;
#91241=EDGE_CURVE ( 'NONE', #76367, #64503, #101616, .T. ) ;
#91248=CARTESIAN_POINT ( 'NONE',  ( 4.609996581545000360, 1516.769879638719885, 205.6626893540170329 ) ) ;
#91258=CARTESIAN_POINT ( 'NONE',  ( -12.33871149695520053, 1512.142158944850053, 194.2604755866809967 ) ) ;
#91266=DIRECTION ( 'NONE',  ( -0.02616798426500965835, 0.9993150019883683122, -0.02616798426500970692 ) ) ;
#91289=CARTESIAN_POINT ( 'NONE',  ( 11.92849869075366698, 1511.839858410422266, 224.1270719350856098 ) ) ;
#91322=CARTESIAN_POINT ( 'NONE',  ( 8.652776089875690246, 1511.435001055579960, 203.7363227723449768 ) ) ;
#91338=EDGE_CURVE ( 'NONE', #7555, #66010, #53672, .T. ) ;
#91353=CARTESIAN_POINT ( 'NONE',  ( 0.7356989345870019736, 1517.020847257979995, 205.6609797614169963 ) ) ;
#91361=EDGE_CURVE ( 'NONE', #78418, #33692, #9134, .T. ) ;
#91369=CARTESIAN_POINT ( 'NONE',  ( -2.865636847234999784, 1516.815173273089840, 210.2578502442970318 ) ) ;
#91398=CARTESIAN_POINT ( 'NONE',  ( 4.616272296565000488, 1517.030858226499959, 201.7868885755270014 ) ) ;
#91399=CARTESIAN_POINT ( 'NONE',  ( 4.031168767865001001, 1516.805675336850072, 208.3649472324300120 ) ) ;
#91413=DIRECTION ( 'NONE',  ( -2.460711850760000078E-19, 5.183526052191769474E-17, 1.000000000000000000 ) ) ;
#91424=CARTESIAN_POINT ( 'NONE',  ( 4.041472473744999405, 1516.858649670339901, 213.1514186109370144 ) ) ;
#91440=ORIENTED_EDGE ( 'NONE', *, *, #18594, .T. ) ;
#91441=CARTESIAN_POINT ( 'NONE',  ( 7.322709686834999232, 1516.596789218710001, 205.8608388005369818 ) ) ;
#91467=CARTESIAN_POINT ( 'NONE',  ( 8.566419661001074104, 1511.406468244436383, 203.9918518157900280 ) ) ;
#91475=CARTESIAN_POINT ( 'NONE',  ( -7.548952336147771724, 1510.510563530936906, 214.7720805601384768 ) ) ;
#91482=CARTESIAN_POINT ( 'NONE',  ( 1.709384572955000126, 1517.224900789629828, 201.7820965968870155 ) ) ;
#91485=CARTESIAN_POINT ( 'NONE',  ( 16.38335852923500013, 1512.258183966700017, 197.2512110842670268 ) ) ;
#91518=CARTESIAN_POINT ( 'NONE',  ( 5.780861236055000241, 1516.783701990830195, 216.0610654530370027 ) ) ;
#91527=CARTESIAN_POINT ( 'NONE',  ( -0.01327408612949850138, 1516.939877939420057, 205.6663500982469941 ) ) ;
#91529=CARTESIAN_POINT ( 'NONE',  ( -5.781585816274999345, 1516.939646076049939, 209.1342929058909874 ) ) ;
#91532=CARTESIAN_POINT ( 'NONE',  ( 6.088832710385000624, 1511.778199792620171, 217.5949148583070212 ) ) ;
#91541=CARTESIAN_POINT ( 'NONE',  ( -4.030514550714999977, 1516.901952101700090, 213.7446888144170032 ) ) ;
#91545=CARTESIAN_POINT ( 'NONE',  ( -7.710855588274700523, 1516.603953730829971, 210.3964488831069843 ) ) ;
#91546=CARTESIAN_POINT ( 'NONE',  ( -7.710967015764999211, 1516.608208975040043, 210.2506035313070072 ) ) ;
#91561=CARTESIAN_POINT ( 'NONE',  ( 5.780232077335000440, 1516.760434454289907, 216.4486414936069991 ) ) ;
#91566=CARTESIAN_POINT ( 'NONE',  ( -1.130607502004999931, 1516.632821972880038, 202.5736453444569918 ) ) ;
#91567=CARTESIAN_POINT ( 'NONE',  ( -16.88678284756500148, 1513.362623229679912, 222.0540973537669913 ) ) ;
#91574=VECTOR ( 'NONE', #22450, 1000.000000000000000 ) ;
#91594=DIRECTION ( 'NONE',  ( 1.000000000000000000, 0.000000000000000000, 0.000000000000000000 ) ) ;
#91629=LINE ( 'NONE', #14905, #12705 ) ;
#91637=CARTESIAN_POINT ( 'NONE',  ( -6.933616859135000254, 1516.548716157039962, 211.4141532006069895 ) ) ;
#91640=CARTESIAN_POINT ( 'NONE',  ( 5.786527562335000319, 1517.025653221279981, 212.5728793591970032 ) ) ;
#91647=CARTESIAN_POINT ( 'NONE',  ( -4.036748876935000396, 1516.667393516340098, 202.1854475764570225 ) ) ;
#91662=CARTESIAN_POINT ( 'NONE',  ( -4.026614517785000125, 1516.699825673279975, 210.8361802174170236 ) ) ;
#91667=CARTESIAN_POINT ( 'NONE',  ( 8.100204432595001336, 1511.336728379370243, 204.5829771873069944 ) ) ;
#91668=CARTESIAN_POINT ( 'NONE',  ( -7.339749373344999661, 1517.224900789629828, 207.4124613591469881 ) ) ;
#91669=ORIENTED_EDGE ( 'NONE', *, *, #96732, .T. ) ;
#91677=CARTESIAN_POINT ( 'NONE',  ( -7.012921583605000286, 1508.551704408389924, 209.1218459511669892 ) ) ;
#91685=CARTESIAN_POINT ( 'NONE',  ( -6.940473372275000052, 1516.833525648419936, 215.6778681647369922 ) ) ;
#91716=CARTESIAN_POINT ( 'NONE',  ( -4.461625834204999919, 1510.696675236759802, 201.5656797203170072 ) ) ;
#91729=CYLINDRICAL_SURFACE ( 'NONE', #60525, 4.999999999999991118 ) ;
#91743=CARTESIAN_POINT ( 'NONE',  ( -15.90990259576500065, 1515.867682058960099, 224.3246417466669982 ) ) ;
#91756=CARTESIAN_POINT ( 'NONE',  ( -7.339107240745000205, 1517.203017563489766, 207.9963360818169917 ) ) ;
#91782=CARTESIAN_POINT ( 'NONE',  ( 4.429773098726779601, 1508.551704408389924, 204.3196138220149862 ) ) ;
#91790=CARTESIAN_POINT ( 'NONE',  ( -4.679794214673830055, 1508.610718243669908, 205.2601826376400140 ) ) ;
#91792=CARTESIAN_POINT ( 'NONE',  ( -1.133517003235000153, 1516.713079096360161, 204.5117660986770147 ) ) ;
#91795=CARTESIAN_POINT ( 'NONE',  ( 15.29490961578690111, 1512.594488815709838, 195.7754158856819799 ) ) ;
#91800=CARTESIAN_POINT ( 'NONE',  ( -12.37943801505299923, 1512.150422497879845, 194.2281132779359893 ) ) ;
#91802=B_SPLINE_CURVE_WITH_KNOTS ( 'NONE', 3,
 ( #69477, #61620, #52111, #94640, #45376, #35292, #2820, #36394, #62180, #19585, #87358, #10654, #87926, #96306, #79516, #103598, #71136, #34738, #17915, #9532, #86241, #43700, #26898, #86797, #61087, #10088, #44262, #78404, #44823, #95752, #78976, #21053, #51117, #76866, #720, #43269 ),
 .UNSPECIFIED., .F., .F.,
 ( 4, 2, 2, 1, 1, 1, 1, 1, 2, 2, 2, 2, 2, 2, 1, 1, 1, 2, 2, 2, 2, 4 ),
 ( 0.000000000000000000, 0.1250000000010887402, 0.1875000000016285029, 0.2187500000019007851, 0.2343750000020369817, 0.2421875000021050661, 0.2460937500021389279, 0.2480468750021558033, 0.2490234375021619373, 0.2500000000021680435, 0.3750000000025698887, 0.4375000000027749469, 0.4687500000028848590, 0.4843750000029383163, 0.4921875000029651281, 0.4960937500029829472, 0.4980468750029918845, 0.4990234375029963809, 0.5000000000030008218, 0.6250000000022466473, 0.7500000000014925838, 1.000000000000000000 ),
 .UNSPECIFIED. ) ;
#91841=CARTESIAN_POINT ( 'NONE',  ( -1.906561486464399589E-08, 1509.038615934239942, 204.6345961781970004 ) ) ;
#91847=EDGE_CURVE ( 'NONE', #6679, #27843, #8539, .T. ) ;
#91886=CARTESIAN_POINT ( 'NONE',  ( -4.668584239039048178, 1511.396718925044297, 200.7090070923989629 ) ) ;
#91891=CARTESIAN_POINT ( 'NONE',  ( -0.01328397755539850039, 1516.939580991450157, 205.8601936452070049 ) ) ;
#91904=CARTESIAN_POINT ( 'NONE',  ( 1.137296650804999976, 1516.908147884120126, 210.8236964273370120 ) ) ;
#91914=ORIENTED_EDGE ( 'NONE', *, *, #52786, .F. ) ;
#91934=EDGE_LOOP ( 'NONE', ( #50054, #106289, #31440, #82843 ) ) ;
#91935=CARTESIAN_POINT ( 'NONE',  ( -7.330554171554999776, 1516.857992118400034, 201.7925428541169879 ) ) ;
#91936=CARTESIAN_POINT ( 'NONE',  ( -3.267039729984999585, 1517.012231669750008, 208.3862772893259887 ) ) ;
#91937=ORIENTED_EDGE ( 'NONE', *, *, #61786, .T. ) ;
#91950=CARTESIAN_POINT ( 'NONE',  ( -5.963459923460841416, 1510.663752962396302, 201.6086580195713793 ) ) ;
#91955=CARTESIAN_POINT ( 'NONE',  ( 2.291047489114999891, 1516.524310051880093, 216.8306159772470210 ) ) ;
#91959=CARTESIAN_POINT ( 'NONE',  ( 2.106986098057376910, 1516.527651687830030, 216.8307034810665357 ) ) ;
#91960=CARTESIAN_POINT ( 'NONE',  ( -4.998515195425000002, 1516.787536375099990, 213.1617432482970003 ) ) ;
#91964=CARTESIAN_POINT ( 'NONE',  ( 4.115862957632160146, 1509.032029411810072, 213.4860450609340319 ) ) ;
#91980=CARTESIAN_POINT ( 'NONE',  ( 2.284199363404999961, 1516.940296199220029, 205.8526610237369994 ) ) ;
#91987=CARTESIAN_POINT ( 'NONE',  ( 7.499999980935001531, 1516.051704408390151, 209.1218459511669892 ) ) ;
#91997=AXIS2_PLACEMENT_3D ( 'NONE', #24993, #7119, #33399 ) ;
#91998=CARTESIAN_POINT ( 'NONE',  ( 3.915802106908682578, 1515.051704408389924, 204.7920544193095509 ) ) ;
#92002=CARTESIAN_POINT ( 'NONE',  ( -13.41825681932545145, 1513.652787279354925, 192.3476914628060399 ) ) ;
#92028=CARTESIAN_POINT ( 'NONE',  ( -7.457021550593670334, 1517.051697240460271, 204.7417221852770126 ) ) ;
#92030=CARTESIAN_POINT ( 'NONE',  ( -0.7538707734179979081, 1516.719999691880048, 202.1833671473370089 ) ) ;
#92033=CARTESIAN_POINT ( 'NONE',  ( 15.46083481443499963, 1513.125294087170005, 194.9058848310670271 ) ) ;
#92043=ORIENTED_EDGE ( 'NONE', *, *, #54284, .T. ) ;
#92046=CARTESIAN_POINT ( 'NONE',  ( -7.615555667685000252, 1511.534866634170157, 211.9602929371470168 ) ) ;
#92060=ORIENTED_EDGE ( 'NONE', *, *, #78018, .F. ) ;
#92065=CARTESIAN_POINT ( 'NONE',  ( -2.289624470354999719, 1517.154223579619838, 215.6854418399169901 ) ) ;
#92072=CARTESIAN_POINT ( 'NONE',  ( 4.997250153905000047, 1516.727068157269969, 205.8570671527170077 ) ) ;
#92074=CARTESIAN_POINT ( 'NONE',  ( -6.949703372784999722, 1517.130100026000036, 208.3827239650380250 ) ) ;
#92086=CARTESIAN_POINT ( 'NONE',  ( -2.480187054844999572, 1517.025470194390209, 213.7472054950769973 ) ) ;
#92091=CARTESIAN_POINT ( 'NONE',  ( -4.997718276504999224, 1516.693851263360102, 210.2547950466569944 ) ) ;
#92106=CARTESIAN_POINT ( 'NONE',  ( 12.49293096393500058, 1511.939906524110256, 224.5925846732669982 ) ) ;
#92112=CARTESIAN_POINT ( 'NONE',  ( -5.005700239535000762, 1516.732530461250008, 202.1838802717869896 ) ) ;
#92113=CARTESIAN_POINT ( 'NONE',  ( -16.11449822786499908, 1514.335759350750095, 224.1254885330670277 ) ) ;
#92114=CARTESIAN_POINT ( 'NONE',  ( 7.512750208045280154, 1509.038615934079871, 214.6352815289239970 ) ) ;
#92132=LINE ( 'NONE', #15407, #55184 ) ;
#92134=CARTESIAN_POINT ( 'NONE',  ( -3.487587101833019787, 1509.038630936360050, 213.6090953315220133 ) ) ;
#92148=EDGE_LOOP ( 'NONE', ( #4378, #19477, #110642, #31305 ) ) ;
#92189=CARTESIAN_POINT ( 'NONE',  ( 4.043366220174999803, 1516.951766529250108, 211.9887038632370206 ) ) ;
#92192=CARTESIAN_POINT ( 'NONE',  ( -2.284199401535000007, 1516.940296199220029, 212.3910308785969789 ) ) ;
#92199=CARTESIAN_POINT ( 'NONE',  ( 2.871580388595000422, 1517.129577905929864, 202.1716309988170224 ) ) ;
#92213=CARTESIAN_POINT ( 'NONE',  ( 0.01319650876840149957, 1516.941178807709775, 211.4140629809269853 ) ) ;
#92219=CARTESIAN_POINT ( 'NONE',  ( 0.7352271172030020452, 1516.963431999339946, 207.4067364850470199 ) ) ;
#92233=CARTESIAN_POINT ( 'NONE',  ( 5.007588646914999941, 1516.804776704140068, 214.8970827629769644 ) ) ;
#92236=CARTESIAN_POINT ( 'NONE',  ( -4.034280953785000179, 1517.049325831759916, 216.0701676760970145 ) ) ;
#92257=ORIENTED_EDGE ( 'NONE', *, *, #80132, .T. ) ;
#92301=CARTESIAN_POINT ( 'NONE',  ( -7.951026619593350553, 1511.645702024530010, 215.1361908920979999 ) ) ;
#92306=CARTESIAN_POINT ( 'NONE',  ( 4.031168767865001001, 1516.805675336850072, 208.3649472324300120 ) ) ;
#92339=CARTESIAN_POINT ( 'NONE',  ( -2.878693287274999957, 1516.766397346390022, 205.0941487061870134 ) ) ;
#92347=CARTESIAN_POINT ( 'NONE',  ( -12.97811974145500002, 1512.378201925219855, 193.9098824635940161 ) ) ;
#92366=CARTESIAN_POINT ( 'NONE',  ( 7.512750207965000371, 1509.038615934239942, 209.1218459511669892 ) ) ;
#92421=CARTESIAN_POINT ( 'NONE',  ( 15.52404075915854165, 1511.843510977572350, 197.7123968315431171 ) ) ;
#92423=CARTESIAN_POINT ( 'NONE',  ( -3.208454056331284665, 1511.804172066353431, 201.1704017881504569 ) ) ;
#92428=CARTESIAN_POINT ( 'NONE',  ( 4.609064303374999838, 1516.723920667490120, 206.2441009858569885 ) ) ;
#92438=CARTESIAN_POINT ( 'NONE',  ( -16.78598030348177161, 1513.543684532448196, 222.3294674479041930 ) ) ;
#92444=CARTESIAN_POINT ( 'NONE',  ( 6.563254890855000134, 1517.139039350860003, 211.6051684241269868 ) ) ;
#92474=CARTESIAN_POINT ( 'NONE',  ( 2.872208710164999790, 1517.145312756229941, 201.7840522196070197 ) ) ;
#92475=CARTESIAN_POINT ( 'NONE',  ( -1.135898823814999847, 1516.958737650239982, 208.0022537503870126 ) ) ;
#92478=CARTESIAN_POINT ( 'NONE',  ( 4.668464111452093945, 1511.396722025383042, 217.5346420084381407 ) ) ;
#92479=ORIENTED_EDGE ( 'NONE', *, *, #47144, .T. ) ;
#92496=CARTESIAN_POINT ( 'NONE',  ( -3.260357166894999992, 1517.133889586189980, 216.8465783791270098 ) ) ;
#92501=CARTESIAN_POINT ( 'NONE',  ( 1.323175339562953301, 1516.595782308469779, 216.8324875441551001 ) ) ;
#92502=CARTESIAN_POINT ( 'NONE',  ( -2.480813923114999930, 1517.051603658920158, 214.1347848340070072 ) ) ;
#92505=CARTESIAN_POINT ( 'NONE',  ( 4.833437557692500164, 1508.551704408439946, 213.0319999308929937 ) ) ;
#92517=CIRCLE ( 'NONE', #1353, 5.000000000000000888 ) ;
#92520=CARTESIAN_POINT ( 'NONE',  ( 3.253141137235000091, 1516.858171774179937, 205.8542424163969997 ) ) ;
#92542=CARTESIAN_POINT ( 'NONE',  ( -14.77680793217355060, 1514.552080547093510, 192.8582046779301606 ) ) ;
#92559=CARTESIAN_POINT ( 'NONE',  ( -7.407689820122348223, 1511.025938507596948, 215.4649457401752102 ) ) ;
#92567=CARTESIAN_POINT ( 'NONE',  ( -5.007588685045000432, 1516.804776704140068, 203.3466091393569855 ) ) ;
#92571=CARTESIAN_POINT ( 'NONE',  ( 15.60002305023500035, 1512.080583811389943, 196.3149055962669820 ) ) ;
#92576=ORIENTED_EDGE ( 'NONE', *, *, #37851, .F. ) ;
#92589=EDGE_CURVE ( 'NONE', #71163, #98390, #104421, .T. ) ;
#92595=CARTESIAN_POINT ( 'NONE',  ( 7.881533592224999829, 1511.927085655870087, 202.8441633797569921 ) ) ;
#92600=EDGE_CURVE ( 'NONE', #36027, #4206, #9217, .T. ) ;
#92605=CARTESIAN_POINT ( 'NONE',  ( -7.328676208015000526, 1516.833844030519913, 216.0648195994369871 ) ) ;
#92606=CARTESIAN_POINT ( 'NONE',  ( -7.976350790930257340, 1511.738149258256499, 212.4166275968371735 ) ) ;
#92613=CARTESIAN_POINT ( 'NONE',  ( -7.724423432224999608, 1517.122088787240045, 205.6676733166769964 ) ) ;
#92615=CARTESIAN_POINT ( 'NONE',  ( 5.786847739675000213, 1517.104497701820037, 209.8595134730280165 ) ) ;
#92618=CARTESIAN_POINT ( 'NONE',  ( 7.521073031005000686, 1513.760531203580058, 215.9563302536469962 ) ) ;
#92630=CARTESIAN_POINT ( 'NONE',  ( 6.947377783174999877, 1517.009964551830080, 213.7374907746170152 ) ) ;
#92637=CARTESIAN_POINT ( 'NONE',  ( 4.044321679994999919, 1517.001127920769704, 211.4073335515969916 ) ) ;
#92640=CARTESIAN_POINT ( 'NONE',  ( -15.90990259576500065, 1516.551704408390151, 220.0820010595669771 ) ) ;
#92650=CARTESIAN_POINT ( 'NONE',  ( 2.872700517194999748, 1516.559109716219837, 216.8315272385270021 ) ) ;
#92651=FACE_OUTER_BOUND ( 'NONE', #78665, .T. ) ;
#92656=CARTESIAN_POINT ( 'NONE',  ( 7.714371502985000184, 1516.738222552470233, 203.3422428319769892 ) ) ;
#92738=CARTESIAN_POINT ( 'NONE',  ( 3.461047291624999911, 1516.858765657450249, 212.5691103191969944 ) ) ;
#92740=CARTESIAN_POINT ( 'NONE',  ( 7.500396670941167798, 1516.934665496271919, 209.1219157010845322 ) ) ;
#92745=CARTESIAN_POINT ( 'NONE',  ( -3.261635970955000019, 1516.613881697390070, 202.1867125516770045 ) ) ;
#92759=CARTESIAN_POINT ( 'NONE',  ( 5.788436334164999586, 1517.116049120239950, 211.4102033778369787 ) ) ;
#92763=B_SPLINE_CURVE_WITH_KNOTS ( 'NONE', 5,
 ( #90439, #80953, #29981, #54676, #38928, #81480, #98846, #28899, #22107, #73108, #105615, #5343 ),
 .UNSPECIFIED., .F., .F.,
 ( 6, 3, 3, 6 ),
 ( -8.927001670199999239, -7.815970586859999791, -6.076675143290000136, -3.686514310890000701 ),
 .UNSPECIFIED. ) ;
#92765=CARTESIAN_POINT ( 'NONE',  ( -2.882326017515000061, 1516.969638403840008, 207.4201161117570109 ) ) ;
#92781=CARTESIAN_POINT ( 'NONE',  ( -1.121383629864999953, 1517.104192383289956, 213.7476359466970166 ) ) ;
#92785=CARTESIAN_POINT ( 'NONE',  ( 5.005700201405000271, 1516.732530461250008, 216.0598116305469887 ) ) ;
#92787=CARTESIAN_POINT ( 'NONE',  ( 7.721072739912949956, 1516.994132466350038, 209.3346182140349754 ) ) ;
#92790=AXIS2_PLACEMENT_3D ( 'NONE', #40172, #31218, #56994 ) ;
#92850=EDGE_CURVE ( 'NONE', #72650, #66010, #72487, .T. ) ;
#92855=CARTESIAN_POINT ( 'NONE',  ( -7.533847566356209668, 1510.598356033829987, 215.0345739407800068 ) ) ;
#92860=CARTESIAN_POINT ( 'NONE',  ( 5.775625077365000415, 1516.745833913490060, 208.3665194962490261 ) ) ;
#92864=AXIS2_PLACEMENT_3D ( 'NONE', #106181, #107277, #63656 ) ;
#92870=CARTESIAN_POINT ( 'NONE',  ( -15.19278571033129843, 1512.351864386150055, 222.0468280374129790 ) ) ;
#92896=CARTESIAN_POINT ( 'NONE',  ( -0.7564342523539989704, 1516.783665406140017, 204.5091745923169810 ) ) ;
#92898=ORIENTED_EDGE ( 'NONE', *, *, #60395, .F. ) ;
#92900=CARTESIAN_POINT ( 'NONE',  ( 15.31201878717920017, 1512.804203059160045, 195.4761085552559905 ) ) ;
#92919=ORIENTED_EDGE ( 'NONE', *, *, #11025, .T. ) ;
#92935=AXIS2_PLACEMENT_3D ( 'NONE', #90083, #66586, #64920 ) ;
#92941=VECTOR ( 'NONE', #67264, 1000.000000000000114 ) ;
#92958=DIRECTION ( 'NONE',  ( 0.4999999999998399058, 0.7071067811867739472, -0.4999999999998399058 ) ) ;
#92977=CARTESIAN_POINT ( 'NONE',  ( -9.638115897704999213, 1516.551704408390151, 203.7504991310570119 ) ) ;
#92981=FACE_OUTER_BOUND ( 'NONE', #48723, .T. ) ;
#92983=CARTESIAN_POINT ( 'NONE',  ( -5.513435588854999736, 1508.551704408389924, 216.1347675159770176 ) ) ;
#92987=CARTESIAN_POINT ( 'NONE',  ( -2.880592967115000125, 1516.859514182039902, 206.2568738160869941 ) ) ;
#92996=CARTESIAN_POINT ( 'NONE',  ( -16.61266726653357040, 1514.059034353336983, 223.2167079213704710 ) ) ;
#93000=CARTESIAN_POINT ( 'NONE',  ( -4.995623491025000362, 1516.636036526019780, 210.8344906863870278 ) ) ;
#93006=DIRECTION ( 'NONE',  ( 2.479303797136877383E-05, 0.02617627755937491918, -0.9996573422320469415 ) ) ;
#93011=ORIENTED_EDGE ( 'NONE', *, *, #15964, .T. ) ;
#93025=CARTESIAN_POINT ( 'NONE',  ( 0.2572000660973332575, 1516.857224341794563, 216.6260235208673635 ) ) ;
#93031=CARTESIAN_POINT ( 'NONE',  ( 4.034908559714999399, 1517.068717944079935, 201.7859449365070077 ) ) ;
#93032=CARTESIAN_POINT ( 'NONE',  ( 6.562094069294999166, 1517.122674412569950, 209.8604508749069737 ) ) ;
#93035=CARTESIAN_POINT ( 'NONE',  ( 3.547742475963274966, 1511.610050756757573, 217.1750692285095568 ) ) ;
#93043=LINE ( 'NONE', #32604, #60306 ) ;
#93052=CARTESIAN_POINT ( 'NONE',  ( -0.7396922758749979732, 1517.135701590510052, 216.4591432822169850 ) ) ;
#93053=ORIENTED_EDGE ( 'NONE', *, *, #64711, .T. ) ;
#93056=CARTESIAN_POINT ( 'NONE',  ( 3.458526497885000328, 1516.742629295279812, 214.1194197574270106 ) ) ;
#93074=CARTESIAN_POINT ( 'NONE',  ( 2.477986732234999767, 1516.922519270759949, 205.8529865360470126 ) ) ;
#93113=CARTESIAN_POINT ( 'NONE',  ( -6.141397734697970456, 1509.034509440879901, 216.6345626749620124 ) ) ;
#93125=AXIS2_PLACEMENT_3D ( 'NONE', #54270, #44199, #104641 ) ;
#93126=CARTESIAN_POINT ( 'NONE',  ( 2.289624432225000117, 1517.154223579619838, 202.5582500624169882 ) ) ;
#93129=CARTESIAN_POINT ( 'NONE',  ( 16.01627747153500181, 1512.526319173689899, 195.5274977073669902 ) ) ;
#93148=LINE ( 'NONE', #74171, #98371 ) ;
#93152=CARTESIAN_POINT ( 'NONE',  ( 6.402238466425000496, 1513.914017980340077, 201.5343560373169964 ) ) ;
#93159=CARTESIAN_POINT ( 'NONE',  ( 6.942344691835000248, 1516.810037859429940, 216.8380980232070101 ) ) ;
#93164=DIRECTION ( 'NONE',  ( 1.000000000000000000, 0.000000000000000000, 0.000000000000000000 ) ) ;
#93166=CARTESIAN_POINT ( 'NONE',  ( -0.7576635715699989726, 1516.855632454399938, 206.2537338009369989 ) ) ;
#93171=CARTESIAN_POINT ( 'NONE',  ( 8.041028920664999191, 1514.881364185380107, 215.2179418010969982 ) ) ;
#93173=ORIENTED_EDGE ( 'NONE', *, *, #63454, .F. ) ;
#93182=CARTESIAN_POINT ( 'NONE',  ( 7.334957356574999920, 1517.030858226499959, 213.7381182667970165 ) ) ;
#93185=FACE_OUTER_BOUND ( 'NONE', #16078, .T. ) ;
#93186=CARTESIAN_POINT ( 'NONE',  ( 6.950833530105000158, 1517.156142772249950, 211.6057959108269984 ) ) ;
#93206=CARTESIAN_POINT ( 'NONE',  ( 0.7386049046750020608, 1517.122674412569950, 202.5597518628069906 ) ) ;
#93237=AXIS2_PLACEMENT_3D ( 'NONE', #46171, #80300, #35527 ) ;
#93249=CARTESIAN_POINT ( 'NONE',  ( 7.136265425265223783, 1516.548173715040548, 206.8118382600278267 ) ) ;
#93288=CARTESIAN_POINT ( 'NONE',  ( 2.296124850935000072, 1516.677239312369920, 213.7299927514870319 ) ) ;
#93291=EDGE_CURVE ( 'NONE', #80871, #2901, #38728, .T. ) ;
#93292=ORIENTED_EDGE ( 'NONE', *, *, #61773, .F. ) ;
#93294=CARTESIAN_POINT ( 'NONE',  ( -2.873958889724999910, 1516.588006113850042, 202.1873174023370154 ) ) ;
#93308=CARTESIAN_POINT ( 'NONE',  ( -4.987078454554999318, 1508.551704408389924, 205.6342535004969818 ) ) ;
#93309=CARTESIAN_POINT ( 'NONE',  ( -3.445201526505000000, 1516.743010792419909, 210.8372070624770060 ) ) ;
#93314=CARTESIAN_POINT ( 'NONE',  ( 2.865636809105000182, 1516.815173273089840, 207.9858416580370033 ) ) ;
#93328=FACE_OUTER_BOUND ( 'NONE', #110670, .T. ) ;
#93329=CARTESIAN_POINT ( 'NONE',  ( 1.132949076425000090, 1516.693851263360102, 214.1195642086070166 ) ) ;
#93332=CARTESIAN_POINT ( 'NONE',  ( -6.942354311545000378, 1516.905946377369901, 216.8406094761369900 ) ) ;
#93399=B_SPLINE_CURVE_WITH_KNOTS ( 'NONE', 3,
 ( #13023, #21417, #66235, #98701, #39900, #55629, #47210, #47755, #21960, #15223, #99786, #23077, #90289, #5759, #81890, #91950, #49416, #30944, #6297, #83540, #90845, #48320, #106556, #5193, #73524, #107657, #99230, #22508, #14130 ),
 .UNSPECIFIED., .F., .F.,
 ( 4, 2, 2, 1, 1, 2, 2, 2, 2, 2, 2, 2, 1, 2, 2, 4 ),
 ( 0.000000000000000000, 0.1250000000022731261, 0.1875000000034070802, 0.2187500000039730719, 0.2343750000041630310, 0.2421875000041678883, 0.2500000000041727732, 0.3750000000024993341, 0.4375000000016680546, 0.5000000000008367751, 0.6249999999991767696, 0.6874999999983395504, 0.7187499999981038501, 0.7343749999981645793, 0.7499999999982251975, 1.000000000000000000 ),
 .UNSPECIFIED. ) ;
#93406=CARTESIAN_POINT ( 'NONE',  ( -7.554100975061009748, 1510.639750819960000, 214.6448992246709793 ) ) ;
#93412=CARTESIAN_POINT ( 'NONE',  ( -4.042388539304999640, 1517.045004075700035, 208.3857484934819979 ) ) ;
#93440=CARTESIAN_POINT ( 'NONE',  ( -1.135460355084999762, 1516.790374942449944, 205.8685445508469911 ) ) ;
#93490=CARTESIAN_POINT ( 'NONE',  ( 7.335900995594999863, 1517.068717944079935, 213.1567545299469657 ) ) ;
#93526=CARTESIAN_POINT ( 'NONE',  ( 14.72576938353500076, 1512.123542805230272, 196.9321265835669976 ) ) ;
#93529=CARTESIAN_POINT ( 'NONE',  ( -2.344512155952720001, 1516.526058380829909, 201.4130301786289863 ) ) ;
#93533=CARTESIAN_POINT ( 'NONE',  ( -4.624736897314999595, 1516.994127245590107, 206.2540423059970180 ) ) ;
#93545=CARTESIAN_POINT ( 'NONE',  ( 3.462620818104999998, 1516.938330505699923, 211.6001527901769919 ) ) ;
#93572=CARTESIAN_POINT ( 'NONE',  ( -7.329925260535000042, 1516.833976295079992, 201.4049670291269933 ) ) ;
#93573=CARTESIAN_POINT ( 'NONE',  ( -6.944466780504999548, 1516.939530130779985, 209.1331108864249870 ) ) ;
#93576=CARTESIAN_POINT ( 'NONE',  ( 4.982648642978618980, 1511.399506464539627, 217.6390045414088092 ) ) ;
#93612=CARTESIAN_POINT ( 'NONE',  ( -6.949265684145000677, 1517.089216728169959, 205.6689289091970068 ) ) ;
#93634=CARTESIAN_POINT ( 'NONE',  ( -14.39972043569755655, 1514.266809408770769, 192.6372960624397308 ) ) ;
#93659=CARTESIAN_POINT ( 'NONE',  ( 0.7376675027960020170, 1517.104497701820037, 203.3349981924270082 ) ) ;
#93671=VERTEX_POINT ( 'NONE', #73870 ) ;
#93694=CARTESIAN_POINT ( 'NONE',  ( 2.485217193935000068, 1516.534320418310244, 216.8308781079170160 ) ) ;
#93695=CARTESIAN_POINT ( 'NONE',  ( -8.335875861980486690, 1511.410071747324082, 213.5558459922955308 ) ) ;
#93701=ADVANCED_FACE ( 'NONE', ( #57637 ), #52794, .T. ) ;
#93703=CARTESIAN_POINT ( 'NONE',  ( 4.608417506514999928, 1516.691389976299888, 206.6316000176769876 ) ) ;
#93709=CARTESIAN_POINT ( 'NONE',  ( 7.770779652545000360, 1514.639648807489948, 215.0467008345069928 ) ) ;
#93718=CARTESIAN_POINT ( 'NONE',  ( 3.457266605394999637, 1516.691414181030041, 214.8945738789770132 ) ) ;
#93721=CARTESIAN_POINT ( 'NONE',  ( 6.141399090249540116, 1509.034509426269778, 216.6345626869079979 ) ) ;
#93722=CARTESIAN_POINT ( 'NONE',  ( 4.043990307595000111, 1516.983612918759945, 211.6010928179370012 ) ) ;
#93730=CARTESIAN_POINT ( 'NONE',  ( 9.638115859575000499, 1516.551704408390151, 214.4931927712770232 ) ) ;
#93733=CARTESIAN_POINT ( 'NONE',  ( 12.18971934853500194, 1512.123542805230272, 223.8476153537669973 ) ) ;
#93735=CARTESIAN_POINT ( 'NONE',  ( -4.035536263215000474, 1517.086065052259983, 216.8453260496270047 ) ) ;
#93737=DIRECTION ( 'NONE',  ( -0.02616798426500960631, -0.9993150019883682011, -0.02616798426500960631 ) ) ;
#93740=CARTESIAN_POINT ( 'NONE',  ( -4.037378294184999383, 1516.688761843659904, 202.5730239910470232 ) ) ;
#93760=CARTESIAN_POINT ( 'NONE',  ( -3.822989278826689930, 1508.729442775010057, 213.6787569762799990 ) ) ;
#93767=CARTESIAN_POINT ( 'NONE',  ( 1.569161254424999985, 1517.051704408389924, 201.3992656178269840 ) ) ;
#93779=ORIENTED_EDGE ( 'NONE', *, *, #24912, .F. ) ;
#93781=CARTESIAN_POINT ( 'NONE',  ( 7.142873439723720352, 1516.547309683342064, 206.8320615317442162 ) ) ;
#93801=CARTESIAN_POINT ( 'NONE',  ( 7.428892750695719194, 1510.947106981214347, 202.8329269027580324 ) ) ;
#93823=CARTESIAN_POINT ( 'NONE',  ( 1.133516965105000107, 1516.713079096360161, 213.7319258036569920 ) ) ;
#93832=CARTESIAN_POINT ( 'NONE',  ( -0.01244697378919850002, 1516.939646076049939, 203.3402601539570185 ) ) ;
#93842=CARTESIAN_POINT ( 'NONE',  ( -11.40944913868885280, 1511.843510977571214, 193.5978051729433957 ) ) ;
#93844=CARTESIAN_POINT ( 'NONE',  ( -15.90990515426090113, 1514.921193439799936, 224.3246443988719818 ) ) ;
#93850=CARTESIAN_POINT ( 'NONE',  ( -2.476733514145000203, 1516.858326417339867, 211.6155457388669845 ) ) ;
#93855=CARTESIAN_POINT ( 'NONE',  ( 4.031168767865001001, 1516.805675336850072, 208.3649472324300120 ) ) ;
#93856=VERTEX_POINT ( 'NONE', #17087 ) ;
#93860=( BOUNDED_CURVE ( )  B_SPLINE_CURVE ( 3, ( #59188, #101691, #25539, #32844 ),
 .UNSPECIFIED., .F., .T. ) 
 B_SPLINE_CURVE_WITH_KNOTS ( ( 4, 4 ),
 ( 1.570952388538209288, 3.141745507188739239 ),
 .UNSPECIFIED. ) 
 CURVE ( )  GEOMETRIC_REPRESENTATION_ITEM ( )  RATIONAL_B_SPLINE_CURVE ( ( 1.000000000000000000, 0.8047386102906373129, 0.8047386102906373129, 1.000000000000000000 ) ) 
 REPRESENTATION_ITEM ( '' )  );
#93870=DIRECTION ( 'NONE',  ( -0.02616798426500965835, -0.9993150019883683122, 0.02616798426500970692 ) ) ;
#93875=CARTESIAN_POINT ( 'NONE',  ( 7.720650135305000994, 1516.977993847330026, 214.9014730243169993 ) ) ;
#93878=CARTESIAN_POINT ( 'NONE',  ( 5.779603100124999671, 1516.738222552470233, 216.8362174732170047 ) ) ;
#93913=CARTESIAN_POINT ( 'NONE',  ( -1.212902923111830011, 1516.615653621559886, 201.4106840095360269 ) ) ;
#93919=EDGE_LOOP ( 'NONE', ( #97967, #36293, #29606 ) ) ;
#93929=LINE ( 'NONE', #19285, #17769 ) ;
#93962=CARTESIAN_POINT ( 'NONE',  ( 5.000329995535000016, 1516.770163853809890, 208.3657552043160024 ) ) ;
#93993=EDGE_CURVE ( 'NONE', #14138, #72956, #84415, .T. ) ;
#93999=CARTESIAN_POINT ( 'NONE',  ( -0.7574260232259989456, 1516.837969789639828, 205.8660360680970030 ) ) ;
#94007=CARTESIAN_POINT ( 'NONE',  ( -14.92122233627069861, 1514.080593477140155, 194.3039127111239850 ) ) ;
#94047=CARTESIAN_POINT ( 'NONE',  ( 1.714334247185000049, 1516.699825673279975, 213.1484604498870112 ) ) ;
#94053=CARTESIAN_POINT ( 'NONE',  ( 5.371346801045000063, 1517.051704408389924, 199.4837300725270097 ) ) ;
#94064=LINE ( 'NONE', #35834, #78168 ) ;
#94088=CARTESIAN_POINT ( 'NONE',  ( 7.321455873725000174, 1516.545806094630279, 206.6359999332069890 ) ) ;
#94098=CARTESIAN_POINT ( 'NONE',  ( -16.44706025664929783, 1514.320576835004431, 223.5963406863797047 ) ) ;
#94102=CARTESIAN_POINT ( 'NONE',  ( -2.476450702264999748, 1516.843453247299749, 211.4215022863270121 ) ) ;
#94132=CARTESIAN_POINT ( 'NONE',  ( 2.288357407604999949, 1517.116049120239950, 203.3334095979369920 ) ) ;
#94133=CARTESIAN_POINT ( 'NONE',  ( 4.037050997585000189, 1516.939819969850078, 209.1086255745840106 ) ) ;
#94136=CARTESIAN_POINT ( 'NONE',  ( 2.941308709124147658, 1512.218044539111133, 217.0079618907426493 ) ) ;
#94143=CARTESIAN_POINT ( 'NONE',  ( -0.4403324739431219714, 1517.051704035390003, 216.6089087266339845 ) ) ;
#94169=CARTESIAN_POINT ( 'NONE',  ( -16.10875979846499817, 1511.961073825299991, 221.2567963359670102 ) ) ;
#94175=CARTESIAN_POINT ( 'NONE',  ( -4.625359562974999506, 1517.025470194390209, 206.6416589153869836 ) ) ;
#94182=( BOUNDED_CURVE ( )  B_SPLINE_CURVE ( 3, ( #64616, #63529, #107137, #20913 ),
 .UNSPECIFIED., .F., .F. ) 
 B_SPLINE_CURVE_WITH_KNOTS ( ( 4, 4 ),
 ( 1.965701907008354667E-12, 0.4510268114855934263 ),
 .UNSPECIFIED. ) 
 CURVE ( )  GEOMETRIC_REPRESENTATION_ITEM ( )  RATIONAL_B_SPLINE_CURVE ( ( 1.000000000000000000, 0.9831196230105666567, 0.9831196230105666567, 1.000000000000000000 ) ) 
 REPRESENTATION_ITEM ( '' )  );
#94197=CARTESIAN_POINT ( 'NONE',  ( -14.28806610630405238, 1514.188942798055677, 192.5865514699557082 ) ) ;
#94222=CARTESIAN_POINT ( 'NONE',  ( 3.257220602695000355, 1517.040132827679827, 203.3350082531769942 ) ) ;
#94225=CYLINDRICAL_SURFACE ( 'NONE', #66253, 0.9999999999999988898 ) ;
#94246=CARTESIAN_POINT ( 'NONE',  ( -0.7351098092479989576, 1516.977504706749869, 211.6135016956469883 ) ) ;
#94250=CARTESIAN_POINT ( 'NONE',  ( 6.534620444044999310, 1514.642928591849795, 201.0029630038770279 ) ) ;
#94259=CARTESIAN_POINT ( 'NONE',  ( 1.129386202275000084, 1516.613712827999962, 216.4452363774470030 ) ) ;
#94265=CARTESIAN_POINT ( 'NONE',  ( -0.01327257453019850021, 1516.940252185109784, 206.2479269295770052 ) ) ;
#94266=ORIENTED_EDGE ( 'NONE', *, *, #69240, .F. ) ;
#94268=CARTESIAN_POINT ( 'NONE',  ( 16.66966702893499885, 1516.995662938509895, 223.5648772753669959 ) ) ;
#94272=CARTESIAN_POINT ( 'NONE',  ( 7.743766081754999142, 1514.370494773850169, 215.3809789565369783 ) ) ;
#94274=VERTEX_POINT ( 'NONE', #26708 ) ;
#94281=CARTESIAN_POINT ( 'NONE',  ( 5.006329581384999727, 1516.755758396839838, 215.6722354023569892 ) ) ;
#94285=CARTESIAN_POINT ( 'NONE',  ( -4.995726007844999650, 1516.651306816259876, 211.4173314712770093 ) ) ;
#94290=EDGE_LOOP ( 'NONE', ( #27318, #105286, #70857, #21637 ) ) ;
#94298=CARTESIAN_POINT ( 'NONE',  ( 5.004442038985000174, 1516.690345681169902, 216.8349637732169697 ) ) ;
#94303=CARTESIAN_POINT ( 'NONE',  ( -1.712644754285000070, 1516.636036526019780, 204.1262224792070015 ) ) ;
#94341=CARTESIAN_POINT ( 'NONE',  ( 7.217397777882030852, 1516.541660446024480, 207.0726429044282781 ) ) ;
#94379=CARTESIAN_POINT ( 'NONE',  ( 4.621267883935000320, 1516.830644417779922, 214.1213023606370029 ) ) ;
#94386=CARTESIAN_POINT ( 'NONE',  ( -6.946748557085000719, 1516.983995446890049, 204.1186252050270014 ) ) ;
#94399=B_SPLINE_CURVE_WITH_KNOTS ( 'NONE', 3,
 ( #73914, #20329, #108042, #57125, #88667, #46126, #80256, #71900, #48721, #82846, #31894, #6136, #40293, #66079, #100204, #53412, #87563, #79169, #45024, #8886, #25129, #50376, #85045, #51458, #57681, #23489, #76112, #91795, #110252, #83395, #32986, #33526, #92900, #84502, #15072, #109172, #50914, #83950, #109711, #42499, #15614, #49268, #49821, #85590, #6693, #40849, #67728, #75022, #101835, #32459, #67175, #59332, #16173, #7792, #66634 ),
 .UNSPECIFIED., .F., .F.,
 ( 4, 3, 3, 3, 3, 3, 3, 3, 3, 3, 3, 3, 3, 3, 3, 3, 3, 3, 4 ),
 ( 9.902195898180000455, 10.17210527305349999, 10.45530577770620084, 10.70141353110000004, 11.00396970308270106, 11.32322756685590015, 11.52456852350000105, 11.84989040654489934, 12.16242387770419953, 12.38020728900000123, 12.74551463658920092, 13.12275145097810025, 13.53252099856839941, 13.95359103769039955, 14.40783883234119855, 14.91487510225679891, 15.44821056775730028, 15.94145638524550179, 16.40090783169999966 ),
 .UNSPECIFIED. ) ;
#94401=CARTESIAN_POINT ( 'NONE',  ( -2.477373643995000485, 1516.891731298979948, 212.0030687278169808 ) ) ;
#94405=CARTESIAN_POINT ( 'NONE',  ( 1.119592181715000079, 1516.958737650239982, 207.9859471464170326 ) ) ;
#94422=CARTESIAN_POINT ( 'NONE',  ( 0.7560907277860019482, 1516.770163853809890, 214.1221759657669850 ) ) ;
#94488=LINE ( 'NONE', #32932, #105265 ) ;
#94494=EDGE_CURVE ( 'NONE', #65542, #93856, #83009, .T. ) ;
#94499=CARTESIAN_POINT ( 'NONE',  ( -4.115882898156034919, 1509.032014410906640, 213.4860376516270719 ) ) ;
#94504=CARTESIAN_POINT ( 'NONE',  ( -7.867033286719529173, 1511.220110216749845, 214.5458993444780162 ) ) ;
#94511=CARTESIAN_POINT ( 'NONE',  ( 7.726684687535000151, 1517.208444099459939, 210.2479840788170122 ) ) ;
#94519=CARTESIAN_POINT ( 'NONE',  ( -15.26795443890799930, 1513.114148094120083, 223.1466213588239782 ) ) ;
#94527=CARTESIAN_POINT ( 'NONE',  ( 2.865636809105000182, 1516.815173273089840, 207.9858416580370033 ) ) ;
#94531=ORIENTED_EDGE ( 'NONE', *, *, #45442, .T. ) ;
#94545=CARTESIAN_POINT ( 'NONE',  ( -3.461360131404999763, 1516.874084700499907, 205.8683838714370040 ) ) ;
#94587=AXIS2_PLACEMENT_3D ( 'NONE', #17604, #51804, #103270 ) ;
#94595=CARTESIAN_POINT ( 'NONE',  ( 2.491188358395000080, 1516.733363207009916, 213.1488973760370129 ) ) ;
#94640=CARTESIAN_POINT ( 'NONE',  ( -5.189380558823482481, 1516.874058588360640, 214.5460175109637362 ) ) ;
#94643=B_SPLINE_CURVE_WITH_KNOTS ( 'NONE', 5,
 ( #11870, #46042, #63409, #97524, #16239, #91322 ),
 .UNSPECIFIED., .F., .F.,
 ( 6, 6 ),
 ( 0.000000000000000000, 1.000000000000000000 ),
 .UNSPECIFIED. ) ;
#94646=CARTESIAN_POINT ( 'NONE',  ( 1.700706776364999895, 1516.923170579120097, 206.8211163054370161 ) ) ;
#94657=CARTESIAN_POINT ( 'NONE',  ( -16.58691043322057368, 1514.105081324218872, 223.2867520483846420 ) ) ;
#94661=CARTESIAN_POINT ( 'NONE',  ( -7.708745685915000756, 1516.523379810429788, 210.8299382363969983 ) ) ;
#94671=VERTEX_POINT ( 'NONE', #103955 ) ;
#94679=ORIENTED_EDGE ( 'NONE', *, *, #37851, .T. ) ;
#94680=CARTESIAN_POINT ( 'NONE',  ( -12.39098292546499991, 1517.051704408389924, 199.8633830690170043 ) ) ;
#94685=CARTESIAN_POINT ( 'NONE',  ( 7.512750234439120156, 1509.038617475950105, 203.6086461444880058 ) ) ;
#94690=CARTESIAN_POINT ( 'NONE',  ( -1.709358701255000001, 1516.542957540330008, 202.1882582765869927 ) ) ;
#94691=CARTESIAN_POINT ( 'NONE',  ( -5.781585816274999345, 1516.939646076049939, 209.1342929058909874 ) ) ;
#94694=CARTESIAN_POINT ( 'NONE',  ( 4.583898368691166070, 1511.400233449630605, 217.5067962340223744 ) ) ;
#94720=ORIENTED_EDGE ( 'NONE', *, *, #23393, .T. ) ;
#94730=CARTESIAN_POINT ( 'NONE',  ( -16.44381314316499854, 1512.620989416249813, 222.6384675079670217 ) ) ;
#94735=CARTESIAN_POINT ( 'NONE',  ( -7.337793750624999944, 1517.145312756229941, 206.2496372219370073 ) ) ;
#94747=ADVANCED_FACE ( 'NONE', ( #79874 ), #5494, .T. ) ;
#94753=CARTESIAN_POINT ( 'NONE',  ( -5.513435705061030312, 1509.038615938849944, 201.6090957135359929 ) ) ;
#94789=CARTESIAN_POINT ( 'NONE',  ( -1.130607502004999931, 1516.632821972880038, 202.5736453444569918 ) ) ;
#94799=EDGE_LOOP ( 'NONE', ( #2848, #44232, #7908, #51659 ) ) ;
#94813=CARTESIAN_POINT ( 'NONE',  ( 5.788097227154999302, 1517.099836525840146, 211.6039138304569747 ) ) ;
#94816=CARTESIAN_POINT ( 'NONE',  ( 6.865869608695000181, 1512.784460098850104, 201.9080085634870159 ) ) ;
#94822=CARTESIAN_POINT ( 'NONE',  ( -7.300067000364999892, 1513.142795523620180, 216.3167343031170162 ) ) ;
#94823=CARTESIAN_POINT ( 'NONE',  ( 16.53955848059638356, 1513.001574290601184, 197.2393618145187020 ) ) ;
#94826=CARTESIAN_POINT ( 'NONE',  ( -1.709384611084999950, 1517.224900789629828, 216.4615953054470197 ) ) ;
#94834=CARTESIAN_POINT ( 'NONE',  ( -0.7578858299649979813, 1516.872851364150165, 206.6414186775969881 ) ) ;
#94845=CARTESIAN_POINT ( 'NONE',  ( -6.014475223502429913, 1511.645396655840159, 201.1712641573570011 ) ) ;
#94852=CARTESIAN_POINT ( 'NONE',  ( 0.01244693565920149993, 1516.939646076049939, 214.9034317483770167 ) ) ;
#94856=CARTESIAN_POINT ( 'NONE',  ( -4.026777524084999449, 1516.718889242609976, 211.4189316860469887 ) ) ;
#94874=CARTESIAN_POINT ( 'NONE',  ( 5.774609621945000271, 1516.777260590120022, 204.5018377250270021 ) ) ;
#94901=LINE ( 'NONE', #10904, #110296 ) ;
#94922=DIRECTION ( 'NONE',  ( -0.02616798426500965835, -0.9993150019883683122, -0.02616798426500960631 ) ) ;
#94925=CARTESIAN_POINT ( 'NONE',  ( -5.385523200472070116, 1511.435001055929888, 200.4690698413500058 ) ) ;
#94955=CARTESIAN_POINT ( 'NONE',  ( 7.334957356574999920, 1517.030858226499959, 213.7381182667970165 ) ) ;
#94956=CARTESIAN_POINT ( 'NONE',  ( 2.830985213604999995, 1512.320675624280057, 216.9025790381570289 ) ) ;
#94958=B_SPLINE_CURVE_WITH_KNOTS ( 'NONE', 3,
 ( #53097, #95633, #46364, #78276, #20020, #18902 ),
 .UNSPECIFIED., .F., .F.,
 ( 4, 2, 4 ),
 ( 0.000000000000000000, 0.5000000000000000000, 1.000000000000000000 ),
 .UNSPECIFIED. ) ;
#94963=CARTESIAN_POINT ( 'NONE',  ( 5.775236792744999903, 1516.804776704140068, 204.1142572851869943 ) ) ;
#94973=CARTESIAN_POINT ( 'NONE',  ( 8.325276386639346882, 1512.905891558394842, 201.7177514598866424 ) ) ;
#94978=CARTESIAN_POINT ( 'NONE',  ( -6.933879441005000643, 1516.560253536979872, 211.6083207129769903 ) ) ;
#94983=CARTESIAN_POINT ( 'NONE',  ( 2.477975315464999717, 1516.839862955080207, 207.9852983471170091 ) ) ;
#94984=ORIENTED_EDGE ( 'NONE', *, *, #92589, .F. ) ;
#94992=FACE_OUTER_BOUND ( 'NONE', #29149, .T. ) ;
#95000=CARTESIAN_POINT ( 'NONE',  ( -3.451033427095000050, 1517.025653221279981, 214.9083735325669977 ) ) ;
#95003=CARTESIAN_POINT ( 'NONE',  ( 7.717505752974999744, 1516.857914730730045, 216.8393517232070167 ) ) ;
#95025=FACE_OUTER_BOUND ( 'NONE', #83876, .T. ) ;
#95036=DIRECTION ( 'NONE',  ( 0.000000000000000000, -1.000000000000000000, -8.596382804469569442E-17 ) ) ;
#95040=ORIENTED_EDGE ( 'NONE', *, *, #2404, .T. ) ;
#95083=CARTESIAN_POINT ( 'NONE',  ( -6.944466780504999548, 1516.939530130779985, 209.1331108864249870 ) ) ;
#95084=CARTESIAN_POINT ( 'NONE',  ( -7.550503362055001055, 1510.480349266450048, 214.6730346442070072 ) ) ;
#95098=CARTESIAN_POINT ( 'NONE',  ( -2.881325412095000260, 1517.003078582959688, 208.0029426616869728 ) ) ;
#95105=CARTESIAN_POINT ( 'NONE',  ( 8.652776089875690246, 1511.435001055579960, 203.7363227723449768 ) ) ;
#95115=CARTESIAN_POINT ( 'NONE',  ( 6.935133380425000382, 1516.613881697390070, 205.8602099992770036 ) ) ;
#95116=EDGE_LOOP ( 'NONE', ( #28574, #20872, #48026, #92479, #109095 ) ) ;
#95135=DIRECTION ( 'NONE',  ( -0.02616798426453448637, 0.9993150019883495494, 0.02616798426619628554 ) ) ;
#95137=CARTESIAN_POINT ( 'NONE',  ( 3.459156578084999989, 1516.769879638719885, 213.7318425517769924 ) ) ;
#95167=CARTESIAN_POINT ( 'NONE',  ( -3.253462098795000035, 1516.874084700499907, 212.5832060635069922 ) ) ;
#95208=CARTESIAN_POINT ( 'NONE',  ( 2.476733476015000157, 1516.858326417339867, 206.6281461634669938 ) ) ;
#95221=CARTESIAN_POINT ( 'NONE',  ( 7.725372132234999967, 1517.158319634930194, 211.9946825927569876 ) ) ;
#95242=CARTESIAN_POINT ( 'NONE',  ( 6.827653005798030250, 1508.551704612109916, 202.6664205262289897 ) ) ;
#95248=CARTESIAN_POINT ( 'NONE',  ( 3.257220602695000355, 1517.040132827679827, 203.3350082531769942 ) ) ;
#95249=CARTESIAN_POINT ( 'NONE',  ( -5.006259886824999228, 1516.939723362869927, 209.1347437590049765 ) ) ;
#95254=CARTESIAN_POINT ( 'NONE',  ( 5.496430422650386838, 1510.805212306365547, 216.6808561322358173 ) ) ;
#95268=EDGE_CURVE ( 'NONE', #598, #11573, #4906, .T. ) ;
#95292=CARTESIAN_POINT ( 'NONE',  ( -16.01627750966499875, 1512.526319173689899, 222.7161941950670041 ) ) ;
#95297=CARTESIAN_POINT ( 'NONE',  ( 4.995725969715000048, 1516.651306816259876, 206.8263604310569690 ) ) ;
#95309=DIRECTION ( 'NONE',  ( -0.6742693640212139572, -4.300014380382889521E-13, -0.7384854939282339270 ) ) ;
#95313=CARTESIAN_POINT ( 'NONE',  ( -2.549111485395000098, 1512.332007210709889, 201.4919753869869794 ) ) ;
#95337=CARTESIAN_POINT ( 'NONE',  ( -6.032863554449749088, 1508.551565390740279, 216.2881064706280085 ) ) ;
#95347=CARTESIAN_POINT ( 'NONE',  ( -7.334328310795000583, 1517.005755693489846, 204.1179978101270081 ) ) ;
#95370=CARTESIAN_POINT ( 'NONE',  ( 6.949574947644999945, 1517.102359858469754, 212.3809477691169718 ) ) ;
#95373=CARTESIAN_POINT ( 'NONE',  ( 6.096095830864999954, 1514.881364185380107, 201.0808170114369773 ) ) ;
#95380=ORIENTED_EDGE ( 'NONE', *, *, #76897, .F. ) ;
#95381=CARTESIAN_POINT ( 'NONE',  ( -7.922128378965000550, 1512.637906871319728, 215.9665121834669890 ) ) ;
#95392=CARTESIAN_POINT ( 'NONE',  ( 6.933879402874999265, 1516.560253536979872, 206.6353711893569880 ) ) ;
#95398=CARTESIAN_POINT ( 'NONE',  ( -7.508705051315979873, 1508.884118747140064, 203.6086422076290035 ) ) ;
#95409=CARTESIAN_POINT ( 'NONE',  ( 4.038637462725000127, 1516.734985836460055, 214.8955147850770118 ) ) ;
#95412=CARTESIAN_POINT ( 'NONE',  ( 5.803572356819420186, 1510.929912129050081, 216.7181665413809810 ) ) ;
#95414=CARTESIAN_POINT ( 'NONE',  ( -2.477986770365000257, 1516.922519270759949, 212.3907053662870226 ) ) ;
#95432=CARTESIAN_POINT ( 'NONE',  ( 4.611879685325000366, 1516.858533673840157, 204.4999481076869756 ) ) ;
#95474=CARTESIAN_POINT ( 'NONE',  ( 4.616272296565000488, 1517.030858226499959, 201.7868885755270014 ) ) ;
#95486=CARTESIAN_POINT ( 'NONE',  ( -7.983219854955000194, 1511.369014903080142, 214.5214372678569816 ) ) ;
#95503=CARTESIAN_POINT ( 'NONE',  ( -2.867803664234999772, 1516.994127245590107, 213.7465828294170080 ) ) ;
#95504=CARTESIAN_POINT ( 'NONE',  ( 3.780286388835000011, 1510.542924508009946, 216.6739878845270084 ) ) ;
#95509=CARTESIAN_POINT ( 'NONE',  ( -2.875850132345000087, 1516.647618671360078, 203.3500485059169876 ) ) ;
#95513=CARTESIAN_POINT ( 'NONE',  ( -2.325731141814999958, 1511.751588929339960, 201.5380540260670159 ) ) ;
#95521=LINE ( 'NONE', #87691, #21023 ) ;
#95525=CARTESIAN_POINT ( 'NONE',  ( 5.011678838024999472, 1516.989560013210166, 212.3778133565769792 ) ) ;
#95531=CARTESIAN_POINT ( 'NONE',  ( 1.701850457105000158, 1516.908147884120126, 207.9845492812970065 ) ) ;
#95540=B_SPLINE_SURFACE_WITH_KNOTS ( 'NONE', 5, 5, ( 
 ( #43876, #28172, #70223, #78019, #26503, #45002, #104327, #103198, #95929 ),
 ( #782, #62932, #19189, #10260, #104882, #103779, #10830, #9709, #3003 ),
 ( #88098, #36572, #19763, #11385, #71324, #70771, #45557, #35467, #105438 ),
 ( #28726, #61265, #97044, #95381, #20307, #54510, #18645, #88647, #1326 ),
 ( #52844, #46103, #34912, #60699, #94822, #18099, #69657, #86970, #44437 ),
 ( #47730, #57256, #56683, #48291, #81311, #82434, #71880, #99758, #4627 ),
 ( #47184, #55050, #20855, #4092, #105996, #29272, #55601, #97583, #89178 ),
 ( #29817, #64552, #38762, #64005, #98672, #63464, #14661, #5730, #12470 ),
 ( #90819, #37675, #81863, #21391, #80233, #72936, #46653, #5164, #39322 ) ),
 .UNSPECIFIED., .F., .F., .F.,
 ( 6, 3, 6 ),
 ( 6, 3, 6 ),
 ( 3.580107477860000387, 6.558749095649999639, 9.700153431729999554 ),
 ( 0.000000000000000000, 0.5000000000000000000, 1.000000000000000000 ),
 .UNSPECIFIED. ) ;
#95546=CARTESIAN_POINT ( 'NONE',  ( 6.556651371285000529, 1516.858146885269889, 215.6747433371770057 ) ) ;
#95551=CARTESIAN_POINT ( 'NONE',  ( 2.485205649205000089, 1517.181921232829836, 201.3958557702769951 ) ) ;
#95586=CARTESIAN_POINT ( 'NONE',  ( -2.386618527720739902, 1516.532192033489991, 201.4128695281360137 ) ) ;
#95631=ORIENTED_EDGE ( 'NONE', *, *, #22009, .F. ) ;
#95632=CARTESIAN_POINT ( 'NONE',  ( -0.7374509209069979310, 1516.978425811520083, 210.2554991112269818 ) ) ;
#95633=CARTESIAN_POINT ( 'NONE',  ( -7.509380800793006294, 1508.909942010299346, 203.6084103740969908 ) ) ;
#95640=CARTESIAN_POINT ( 'NONE',  ( -15.10400618450110066, 1513.569700117909861, 223.6131665486809936 ) ) ;
#95649=CARTESIAN_POINT ( 'NONE',  ( -1.717139122245000094, 1516.949031626070109, 208.0040058453670042 ) ) ;
#95651=CARTESIAN_POINT ( 'NONE',  ( -6.742044282776496367, 1509.032357808383040, 216.2339691194059696 ) ) ;
#95666=CARTESIAN_POINT ( 'NONE',  ( -7.337153806245000354, 1517.119374999550018, 205.8621166342670108 ) ) ;
#95669=CARTESIAN_POINT ( 'NONE',  ( -3.724929251180815193, 1516.669760784821392, 202.6114878535433945 ) ) ;
#95677=CARTESIAN_POINT ( 'NONE',  ( 6.541070334811199594, 1517.051704644130041, 212.7912326336579838 ) ) ;
#95688=CARTESIAN_POINT ( 'NONE',  ( 2.489617538345000103, 1516.665179208830068, 214.1178407578070164 ) ) ;
#95715=CARTESIAN_POINT ( 'NONE',  ( -2.284526496774999860, 1516.956048353049937, 212.5847947667770086 ) ) ;
#95739=ORIENTED_EDGE ( 'NONE', *, *, #52786, .T. ) ;
#95752=CARTESIAN_POINT ( 'NONE',  ( -7.151171913976369865, 1516.544165615068778, 211.3944463322366687 ) ) ;
#95755=CARTESIAN_POINT ( 'NONE',  ( -8.788316527315000570, 1511.741868877540128, 215.3741124244170067 ) ) ;
#95757=CARTESIAN_POINT ( 'NONE',  ( -2.299983615734999987, 1516.861367446839949, 206.8392230197369770 ) ) ;
#95770=CARTESIAN_POINT ( 'NONE',  ( 2.879956924955000108, 1516.827328999679821, 212.3743765858270081 ) ) ;
#95790=CARTESIAN_POINT ( 'NONE',  ( 7.260542949781179978, 1508.878901734200099, 202.3557440548540285 ) ) ;
#95794=ORIENTED_EDGE ( 'NONE', *, *, #47144, .F. ) ;
#95795=CARTESIAN_POINT ( 'NONE',  ( -5.780861274184998955, 1516.783701990830195, 202.1826264492970324 ) ) ;
#95796=CARTESIAN_POINT ( 'NONE',  ( -3.449647478144999724, 1516.829948096479939, 209.8791439064560223 ) ) ;
#95808=CARTESIAN_POINT ( 'NONE',  ( -0.4346943098025670138, 1517.051704408590012, 216.8444262844809884 ) ) ;
#95817=CARTESIAN_POINT ( 'NONE',  ( -6.998420887974999616, 1512.696049264740168, 200.9299854953570161 ) ) ;
#95823=( BOUNDED_CURVE ( )  B_SPLINE_CURVE ( 3, ( #41498, #51001, #56, #92983 ),
 .UNSPECIFIED., .F., .F. ) 
 B_SPLINE_CURVE_WITH_KNOTS ( ( 4, 4 ),
 ( 2.356690338815510266, 3.926801539092879878 ),
 .UNSPECIFIED. ) 
 CURVE ( )  GEOMETRIC_REPRESENTATION_ITEM ( )  RATIONAL_B_SPLINE_CURVE ( ( 1.000000000000000000, 0.8048993123304821751, 0.8048993123304821751, 1.000000000000000000 ) ) 
 REPRESENTATION_ITEM ( '' )  );
#95839=CARTESIAN_POINT ( 'NONE',  ( 3.487592431604999987, 1508.551704408389924, 204.1347675156769981 ) ) ;
#95840=CARTESIAN_POINT ( 'NONE',  ( -4.043366258305000294, 1516.951766529250108, 206.2549880390970145 ) ) ;
#95859=CARTESIAN_POINT ( 'NONE',  ( 5.750872949060175543, 1510.549724832337461, 216.6642929926275087 ) ) ;
#95896=CARTESIAN_POINT ( 'NONE',  ( -5.784638357945000031, 1516.939574742129935, 204.5080835752170003 ) ) ;
#95917=CARTESIAN_POINT ( 'NONE',  ( -2.477986770365000257, 1516.922519270759949, 212.3907053662870226 ) ) ;
#95925=ORIENTED_EDGE ( 'NONE', *, *, #90442, .T. ) ;
#95929=CARTESIAN_POINT ( 'NONE',  ( -7.396545081264999766, 1511.069621805459974, 215.4940135707870184 ) ) ;
#95941=CARTESIAN_POINT ( 'NONE',  ( -6.951175166914999259, 1517.170721208160103, 206.8315896683770063 ) ) ;
#95946=CARTESIAN_POINT ( 'NONE',  ( -6.120078482172389478, 1508.729259781710198, 201.6787668352259857 ) ) ;
#95957=CARTESIAN_POINT ( 'NONE',  ( -2.482067898354999969, 1517.099836525840146, 214.9099431973869798 ) ) ;
#95960=CARTESIAN_POINT ( 'NONE',  ( 5.570674229300860425, 1511.275365984429982, 217.0209262882389964 ) ) ;
#95962=CARTESIAN_POINT ( 'NONE',  ( -4.609673279564999504, 1516.754149861460064, 212.3872530880769887 ) ) ;
#95970=CARTESIAN_POINT ( 'NONE',  ( -7.599227184291730275, 1512.341036968809931, 211.3567690145959830 ) ) ;
#95979=CARTESIAN_POINT ( 'NONE',  ( -1.132949114555000136, 1516.693851263360102, 204.1241276937270186 ) ) ;
#96009=EDGE_CURVE ( 'NONE', #68646, #55731, #94901, .T. ) ;
#96020=CARTESIAN_POINT ( 'NONE',  ( 5.004475574535000248, 1517.026025493960105, 201.3999380438669959 ) ) ;
#96025=CARTESIAN_POINT ( 'NONE',  ( 7.691516654014999510, 1512.326491219019999, 206.4237331406770011 ) ) ;
#96035=CARTESIAN_POINT ( 'NONE',  ( -7.559673342214999536, 1510.830536680500245, 212.2954481221070182 ) ) ;
#96057=CARTESIAN_POINT ( 'NONE',  ( 6.945490048805000427, 1516.932669162149978, 214.9002185338470099 ) ) ;
#96058=CARTESIAN_POINT ( 'NONE',  ( 3.558864023334999960, 1511.483345606789953, 217.0119653402770155 ) ) ;
#96063=CARTESIAN_POINT ( 'NONE',  ( -6.557909920764999789, 1516.908489800550115, 203.3441005368270282 ) ) ;
#96065=DIRECTION ( 'NONE',  ( 8.673617379884002932E-16, 0.02617694830786544691, -0.9996573249755575929 ) ) ;
#96066=CARTESIAN_POINT ( 'NONE',  ( 3.801734845580006183, 1509.034509900239755, 204.6344869756675848 ) ) ;
#96075=CARTESIAN_POINT ( 'NONE',  ( 6.562635822504999439, 1517.111322026010157, 211.9927976380170094 ) ) ;
#96080=CARTESIAN_POINT ( 'NONE',  ( -6.944466780504999548, 1516.939530130779985, 209.1331108864249870 ) ) ;
#96093=EDGE_CURVE ( 'NONE', #20112, #58764, #48369, .T. ) ;
#96094=CARTESIAN_POINT ( 'NONE',  ( 0.7543881828220019292, 1516.727502608469877, 215.6727161143369926 ) ) ;
#96106=CARTESIAN_POINT ( 'NONE',  ( 7.546131039266060547, 1510.764648358900104, 203.2669580094189996 ) ) ;
#96136=CARTESIAN_POINT ( 'NONE',  ( -1.677883752140799878, 1516.549122391340006, 201.4124261911130134 ) ) ;
#96144=ORIENTED_EDGE ( 'NONE', *, *, #50627, .T. ) ;
#96162=AXIS2_PLACEMENT_3D ( 'NONE', #53105, #87243, #20561 ) ;
#96186=CARTESIAN_POINT ( 'NONE',  ( -5.000330033664999618, 1516.770163853809890, 209.8779366980180328 ) ) ;
#96197=EDGE_CURVE ( 'NONE', #21616, #56695, #2708, .T. ) ;
#96202=ORIENTED_EDGE ( 'NONE', *, *, #35093, .T. ) ;
#96204=CARTESIAN_POINT ( 'NONE',  ( -1.135898823814999847, 1516.958737650239982, 208.0022537503870126 ) ) ;
#96220=CARTESIAN_POINT ( 'NONE',  ( 7.321193707744999557, 1516.534976163889951, 206.8301696586770220 ) ) ;
#96239=CARTESIAN_POINT ( 'NONE',  ( 0.7564342142240020328, 1516.783665406140017, 213.7345173100169973 ) ) ;
#96306=CARTESIAN_POINT ( 'NONE',  ( -6.073016847162494791, 1516.743606062366780, 213.5232657706371810 ) ) ;
#96310=CARTESIAN_POINT ( 'NONE',  ( -3.462948834675000143, 1516.956048353049937, 206.8373194734570006 ) ) ;
#96324=CARTESIAN_POINT ( 'NONE',  ( -2.476733514145000203, 1516.858326417339867, 211.6155457388669845 ) ) ;
#96332=VERTEX_POINT ( 'NONE', #35969 ) ;
#96334=CARTESIAN_POINT ( 'NONE',  ( 12.24386287430722575, 1513.118420038113072, 225.7974128742104369 ) ) ;
#96347=CARTESIAN_POINT ( 'NONE',  ( 7.203707678260440339, 1508.728101425929935, 202.3962581857610132 ) ) ;
#96352=CARTESIAN_POINT ( 'NONE',  ( 7.715625202974999652, 1516.786099423779888, 202.5670817708370066 ) ) ;
#96353=CARTESIAN_POINT ( 'NONE',  ( 4.626591867355000609, 1517.096587378560116, 210.8266407735670214 ) ) ;
#96358=CARTESIAN_POINT ( 'NONE',  ( -9.813597492012577916, 1516.551188145990182, 203.5583050039579973 ) ) ;
#96373=CARTESIAN_POINT ( 'NONE',  ( -7.587489932915000068, 1513.914017980330073, 202.7196074656669964 ) ) ;
#96376=CIRCLE ( 'NONE', #98199, 5.000000000000000888 ) ;
#96391=CARTESIAN_POINT ( 'NONE',  ( 15.21523570123499880, 1514.242353506929931, 224.0841638630670047 ) ) ;
#96400=CARTESIAN_POINT ( 'NONE',  ( 3.251888829344999898, 1516.793978928989873, 206.6294022811970024 ) ) ;
#96419=CARTESIAN_POINT ( 'NONE',  ( -2.930838077694999821, 1510.983859056260144, 201.5581577403170002 ) ) ;
#96453=CARTESIAN_POINT ( 'NONE',  ( 4.998515157294999511, 1516.787536375099990, 205.0819486540370065 ) ) ;
#96457=CIRCLE ( 'NONE', #46435, 0.9999999999999986677 ) ;
#96473=CARTESIAN_POINT ( 'NONE',  ( -4.997250192034999650, 1516.727068157269969, 212.3866247496169990 ) ) ;
#96495=CARTESIAN_POINT ( 'NONE',  ( 7.708745647785000266, 1516.523379810429788, 207.4137536659370085 ) ) ;
#96513=CARTESIAN_POINT ( 'NONE',  ( 7.330554133425000174, 1516.857992118400034, 216.4511490482170188 ) ) ;
#96515=CARTESIAN_POINT ( 'NONE',  ( 6.092700134410669932, 1510.714321716100130, 216.6162777139399793 ) ) ;
#96518=CARTESIAN_POINT ( 'NONE',  ( 3.267603515704999850, 1516.858171774179937, 212.3749871074670068 ) ) ;
#96538=CARTESIAN_POINT ( 'NONE',  ( 6.937338745574999521, 1516.706638732659940, 204.5037262658370025 ) ) ;
#96582=VECTOR ( 'NONE', #20086, 1000.000000000000000 ) ;
#96583=CARTESIAN_POINT ( 'NONE',  ( -6.554764199395000546, 1516.786099423779888, 201.4062207291269999 ) ) ;
#96587=CARTESIAN_POINT ( 'NONE',  ( 7.780733067925000412, 1512.320675624280057, 206.2908607184970151 ) ) ;
#96589=B_SPLINE_SURFACE_WITH_KNOTS ( 'NONE', 5, 5, ( 
 ( #22904, #64408, #13405, #81177, #90123, #30218 ),
 ( #100193, #14518, #73904, #82832, #72802, #99070 ),
 ( #6124, #4493, #15059, #21799, #97974, #108593 ),
 ( #90678, #73346, #40280, #22349, #74465, #91782 ),
 ( #39170, #31880, #57669, #81718, #31327, #56550 ),
 ( #13964, #98531, #108030, #55999, #106929, #82290 ) ),
 .UNSPECIFIED., .F., .F., .F.,
 ( 6, 6 ),
 ( 6, 6 ),
 ( 4.250940516431700011, 7.082035122218299783 ),
 ( -9.670478295150139691E-06, 0.5000000000000000000 ),
 .UNSPECIFIED. ) ;
#96597=CARTESIAN_POINT ( 'NONE',  ( -7.888956606115001158, 1511.220390575160081, 213.9483244531670039 ) ) ;
#96601=CARTESIAN_POINT ( 'NONE',  ( 8.181958942834999249, 1517.051704408389924, 212.1568108385370124 ) ) ;
#96618=CARTESIAN_POINT ( 'NONE',  ( 7.331812085974999782, 1516.906641539930206, 215.6759973964769870 ) ) ;
#96619=CARTESIAN_POINT ( 'NONE',  ( 4.495269857704999872, 1510.967342883699985, 216.7778746379670167 ) ) ;
#96624=CARTESIAN_POINT ( 'NONE',  ( 6.936398355645000180, 1516.667393516340098, 205.0850970932970085 ) ) ;
#96625=VECTOR ( 'NONE', #6085, 1000.000000000000000 ) ;
#96640=VECTOR ( 'NONE', #85995, 1000.000000000000000 ) ;
#96641=CARTESIAN_POINT ( 'NONE',  ( 4.042417777704999438, 1516.904492006980036, 212.5700528489170154 ) ) ;
#96646=EDGE_CURVE ( 'NONE', #44905, #20112, #72946, .T. ) ;
#96647=CARTESIAN_POINT ( 'NONE',  ( -6.556851034704999748, 1516.939568781210028, 209.1335575761840175 ) ) ;
#96655=DIRECTION ( 'NONE',  ( 0.7384854939285241393, 0.000000000000000000, -0.6742693640208961003 ) ) ;
#96662=CARTESIAN_POINT ( 'NONE',  ( 2.294209629405000062, 1516.603620185149794, 214.8927295341169952 ) ) ;
#96667=CARTESIAN_POINT ( 'NONE',  ( 5.779627054084999216, 1516.977993847330026, 201.4011957967969977 ) ) ;
#96725=AXIS2_PLACEMENT_3D ( 'NONE', #64972, #99087, #39758 ) ;
#96728=CARTESIAN_POINT ( 'NONE',  ( 7.722580314274999580, 1517.051704408389924, 210.6910072246569996 ) ) ;
#96732=EDGE_CURVE ( 'NONE', #47285, #60389, #94064, .T. ) ;
#96737=VECTOR ( 'NONE', #103488, 1000.000000000000114 ) ;
#96748=CARTESIAN_POINT ( 'NONE',  ( -4.610079871555000430, 1516.713079096360161, 210.2553629353369899 ) ) ;
#96754=CARTESIAN_POINT ( 'NONE',  ( 15.90990255763500016, 1515.867682058960099, 193.9190501556669801 ) ) ;
#96757=CARTESIAN_POINT ( 'NONE',  ( -2.291047527245000381, 1516.524310051880093, 201.4130759250869858 ) ) ;
#96764=CARTESIAN_POINT ( 'NONE',  ( 3.447128460625000113, 1516.778853242349896, 207.9866608880570027 ) ) ;
#96781=CARTESIAN_POINT ( 'NONE',  ( 6.546302742015000398, 1516.577434278289957, 206.6347425125669872 ) ) ;
#96791=CARTESIAN_POINT ( 'NONE',  ( 7.722580339391510229, 1517.051704402239920, 213.7119063846940037 ) ) ;
#96799=CARTESIAN_POINT ( 'NONE',  ( 0.01171160595180150039, 1516.939568781210028, 215.6786969668069958 ) ) ;
#96834=( BOUNDED_CURVE ( )  B_SPLINE_CURVE ( 3, ( #103963, #18837, #62563, #27260 ),
 .UNSPECIFIED., .F., .T. ) 
 B_SPLINE_CURVE_WITH_KNOTS ( ( 4, 4 ),
 ( 2.356690340185370047, 3.926801538374500300 ),
 .UNSPECIFIED. ) 
 CURVE ( )  GEOMETRIC_REPRESENTATION_ITEM ( )  RATIONAL_B_SPLINE_CURVE ( ( 1.000000000000000000, 0.8048993128225162552, 0.8048993128225162552, 1.000000000000000000 ) ) 
 REPRESENTATION_ITEM ( '' )  );
#96849=( LENGTH_UNIT ( ) NAMED_UNIT ( * ) SI_UNIT ( .MILLI., .METRE. ) );
#96871=CARTESIAN_POINT ( 'NONE',  ( 2.282915183265000092, 1516.876240617270014, 206.6278256496669883 ) ) ;
#96908=CARTESIAN_POINT ( 'NONE',  ( 6.937338745574999521, 1516.706638732659940, 204.5037262658370025 ) ) ;
#96927=DIRECTION ( 'NONE',  ( -3.659266894335750173E-33, 6.123233995736769734E-17, 1.000000000000000000 ) ) ;
#96932=CARTESIAN_POINT ( 'NONE',  ( -6.560424634844999936, 1512.053281741900037, 200.4573988352969707 ) ) ;
#96949=CARTESIAN_POINT ( 'NONE',  ( 13.06501229733500047, 1513.192861445620110, 226.0202954981670302 ) ) ;
#96953=CARTESIAN_POINT ( 'NONE',  ( -5.371346839175000554, 1517.051704408389924, 218.7599618298069970 ) ) ;
#96957=CARTESIAN_POINT ( 'NONE',  ( 4.026777485955000735, 1516.718889242609976, 206.8247602162870180 ) ) ;
#97013=CARTESIAN_POINT ( 'NONE',  ( 2.287084270065000258, 1517.068517094990057, 204.1085709707169826 ) ) ;
#97028=FACE_OUTER_BOUND ( 'NONE', #12982, .T. ) ;
#97034=CARTESIAN_POINT ( 'NONE',  ( -7.322709724964999722, 1516.596789218710001, 212.3828531017969965 ) ) ;
#97044=CARTESIAN_POINT ( 'NONE',  ( -8.061256588785001398, 1512.677556571460173, 216.0330363529270130 ) ) ;
#97045=CARTESIAN_POINT ( 'NONE',  ( 16.75056590446115479, 1513.749562441641729, 195.5293526489948874 ) ) ;
#97054=CARTESIAN_POINT ( 'NONE',  ( 4.026777485955000735, 1516.718889242609976, 206.8247602162870180 ) ) ;
#97059=CARTESIAN_POINT ( 'NONE',  ( -7.443079267411500055, 1508.729259695960081, 203.0017376064890016 ) ) ;
#97066=DIRECTION ( 'NONE',  ( -0.4770263929453589236, -0.7067418228232984490, -0.5224574779883445208 ) ) ;
#97071=CARTESIAN_POINT ( 'NONE',  ( 6.942973629204999497, 1516.833844030519913, 216.4505221401170161 ) ) ;
#97073=CARTESIAN_POINT ( 'NONE',  ( 5.863482170922579506, 1511.603576927810082, 217.5746331517350143 ) ) ;
#97076=CARTESIAN_POINT ( 'NONE',  ( 4.624736859184999993, 1516.994127245590107, 211.9896495963369887 ) ) ;
#97093=CARTESIAN_POINT ( 'NONE',  ( -3.460101890015000237, 1516.812923327049930, 205.0932153474469715 ) ) ;
#97126=CARTESIAN_POINT ( 'NONE',  ( -13.59755241946499993, 1512.525301340730039, 193.3332859498670189 ) ) ;
#97136=CARTESIAN_POINT ( 'NONE',  ( -17.10989647720995777, 1517.051704408390151, 195.2932400735099066 ) ) ;
#97142=CARTESIAN_POINT ( 'NONE',  ( -7.890119408174999904, 1511.483345606789953, 212.6807099935669783 ) ) ;
#97159=CARTESIAN_POINT ( 'NONE',  ( -1.705466448594999962, 1517.120861839400050, 214.1360410720469929 ) ) ;
#97160=CARTESIAN_POINT ( 'NONE',  ( 5.181410150655000990, 1510.418062979269962, 216.6707182703270291 ) ) ;
#97166=CARTESIAN_POINT ( 'NONE',  ( -6.947377821305000367, 1517.009964551830080, 204.5062011277169916 ) ) ;
#97177=CARTESIAN_POINT ( 'NONE',  ( -1.119717754394999876, 1517.038650117239968, 212.5846815975970117 ) ) ;
#97182=CARTESIAN_POINT ( 'NONE',  ( 5.011551368014999674, 1517.080322339569875, 209.8587501411369942 ) ) ;
#97187=EDGE_LOOP ( 'NONE', ( #92257, #87994, #44999 ) ) ;
#97195=CARTESIAN_POINT ( 'NONE',  ( 6.943602653455000606, 1516.858069504249897, 216.0629462479770098 ) ) ;
#97205=CARTESIAN_POINT ( 'NONE',  ( 8.629219820895000836, 1511.600194708689969, 203.2115927965309936 ) ) ;
#97207=UNCERTAINTY_MEASURE_WITH_UNIT (LENGTH_MEASURE( 1.000000000000000082E-05 ), #106100, 'distance_accuracy_value', 'NONE');
#97223=CARTESIAN_POINT ( 'NONE',  ( 15.90990255763500016, 1516.551704408390151, 198.1616908427670296 ) ) ;
#97225=CYLINDRICAL_SURFACE ( 'NONE', #14467, 0.9999999999999988898 ) ;
#97236=CARTESIAN_POINT ( 'NONE',  ( -0.5542586829518019176, 1516.774419107840004, 201.4065265889630041 ) ) ;
#97240=CARTESIAN_POINT ( 'NONE',  ( 13.40617544342749845, 1512.633419863019981, 224.4245124526530049 ) ) ;
#97283=CARTESIAN_POINT ( 'NONE',  ( 6.951175128784999657, 1517.170721208160103, 211.4121022339570004 ) ) ;
#97290=VERTEX_POINT ( 'NONE', #11605 ) ;
#97293=CARTESIAN_POINT ( 'NONE',  ( -1.129386240404999908, 1516.613712827999962, 201.7984555248870038 ) ) ;
#97315=CARTESIAN_POINT ( 'NONE',  ( -6.562635860634999929, 1517.111322026010157, 206.2508942643169974 ) ) ;
#97331=CARTESIAN_POINT ( 'NONE',  ( -2.288357445734999995, 1517.116049120239950, 214.9102823043970147 ) ) ;
#97334=CARTESIAN_POINT ( 'NONE',  ( 7.722580314274999580, 1517.051704408389924, 210.6910072246569996 ) ) ;
#97350=DIRECTION ( 'NONE',  ( -1.000000000000000000, 0.000000000000000000, 0.000000000000000000 ) ) ;
#97351=VECTOR ( 'NONE', #30666, 999.9999999999998863 ) ;
#97393=CARTESIAN_POINT ( 'NONE',  ( -7.203707716490680646, 1508.728101425919931, 215.8474337165719987 ) ) ;
#97405=EDGE_CURVE ( 'NONE', #17368, #8750, #42856, .T. ) ;
#97406=CARTESIAN_POINT ( 'NONE',  ( -5.014195139944999546, 1517.120861839400050, 207.4163795216369977 ) ) ;
#97423=B_SPLINE_CURVE_WITH_KNOTS ( 'NONE', 3,
 ( #98709, #46142, #30953, #47217, #89214, #90856, #4658, #38797, #21969, #47764, #99241, #22517, #91959, #33695, #102544, #15236, #76822, #33150, #25837, #49970, #41571, #92501, #6843, #60038, #24727, #68441, #14698, #23651, #67338, #34259, #85204, #24186, #75182, #110415, #74629, #66246, #50528, #83015, #101437, #41004 ),
 .UNSPECIFIED., .F., .F.,
 ( 4, 1, 1, 1, 1, 2, 2, 1, 1, 1, 2, 2, 1, 1, 2, 2, 1, 1, 1, 1, 2, 2, 1, 1, 1, 2, 2, 4 ),
 ( 0.000000000000000000, 0.06249999999983144039, 0.09374999999974716058, 0.1093749999997047639, 0.1171874999996835309, 0.1210937499996792149, 0.1249999999996748989, 0.1874999999995648203, 0.2187499999995081157, 0.2343749999994797772, 0.2421874999994653443, 0.2499999999994509392, 0.3749999999992617572, 0.4374999999991670552, 0.4687499999991197042, 0.4999999999990722976, 0.5624999999990122346, 0.5937499999989822586, 0.6093749999989873656, 0.6171874999989899191, 0.6210937499989912514, 0.6249999999989925836, 0.6874999999992860156, 0.7187499999994573230, 0.7343749999995197175, 0.7421874999995508038, 0.7499999999995818900, 1.000000000000000000 ),
 .UNSPECIFIED. ) ;
#97430=CARTESIAN_POINT ( 'NONE',  ( 13.24077306275803068, 1513.560745840759637, 225.9062032717914974 ) ) ;
#97446=ORIENTED_EDGE ( 'NONE', *, *, #39098, .F. ) ;
#97451=CARTESIAN_POINT ( 'NONE',  ( -7.721907926364999675, 1517.026025493960105, 204.1173703575669833 ) ) ;
#97471=CARTESIAN_POINT ( 'NONE',  ( -7.942827010805000754, 1514.298059036109862, 202.2691041254170159 ) ) ;
#97476=CARTESIAN_POINT ( 'NONE',  ( -7.167383222404231979, 1508.551704408387423, 214.6352815287315252 ) ) ;
#97487=CARTESIAN_POINT ( 'NONE',  ( 15.20279853403500070, 1514.921193539169963, 225.0317509809670184 ) ) ;
#97496=CARTESIAN_POINT ( 'NONE',  ( -0.01265822594359850006, 1516.959716008189844, 207.4120794380770292 ) ) ;
#97515=CARTESIAN_POINT ( 'NONE',  ( 6.054581389202323471, 1510.727597956443788, 216.6161816537009486 ) ) ;
#97524=CARTESIAN_POINT ( 'NONE',  ( 7.983219802273961996, 1511.369014876796655, 203.7222547165445690 ) ) ;
#97530=DIRECTION ( 'NONE',  ( 0.7071067811865492381, 0.000000000000000000, -0.7071067811865457964 ) ) ;
#97548=EDGE_CURVE ( 'NONE', #28577, #65542, #91802, .T. ) ;
#97552=CARTESIAN_POINT ( 'NONE',  ( -1.132949114555000136, 1516.693851263360102, 204.1241276937270186 ) ) ;
#97573=CARTESIAN_POINT ( 'NONE',  ( 2.298369469825000344, 1516.779243033999819, 212.3734572960470075 ) ) ;
#97583=CARTESIAN_POINT ( 'NONE',  ( -6.242053784335000799, 1513.743447518359972, 216.6918286318270077 ) ) ;
#97584=CARTESIAN_POINT ( 'NONE',  ( 16.23489788457936811, 1514.585431650382588, 194.3036092076362991 ) ) ;
#97597=CARTESIAN_POINT ( 'NONE',  ( -3.269984819434999856, 1516.999105586269934, 207.4194399470370058 ) ) ;
#97609=CARTESIAN_POINT ( 'NONE',  ( -5.705922872222989994, 1511.346048414110101, 201.2009718814310020 ) ) ;
#97615=CARTESIAN_POINT ( 'NONE',  ( 6.943602653455000606, 1516.858069504249897, 216.0629462479770098 ) ) ;
#97617=CARTESIAN_POINT ( 'NONE',  ( 0.4346943641293429805, 1517.051704428850144, 201.3992661435559910 ) ) ;
#97620=CARTESIAN_POINT ( 'NONE',  ( 6.949574947644999945, 1517.102359858469754, 212.3809477691169718 ) ) ;
#97637=CARTESIAN_POINT ( 'NONE',  ( -3.459156616214999591, 1516.769879638719885, 204.5118493505569859 ) ) ;
#97656=CARTESIAN_POINT ( 'NONE',  ( -12.01221612688690676, 1513.042033678214011, 192.5302509902024610 ) ) ;
#97671=CARTESIAN_POINT ( 'NONE',  ( -13.56546627376500069, 1512.571022561229938, 193.5522729196669900 ) ) ;
#97688=CARTESIAN_POINT ( 'NONE',  ( -7.622960524865000309, 1511.191277613550028, 212.5075598512569854 ) ) ;
#97695=SURFACE_SIDE_STYLE ('',( #89296 ) ) ;
#97701=VERTEX_POINT ( 'NONE', #104269 ) ;
#97708=CARTESIAN_POINT ( 'NONE',  ( 7.720650135305000994, 1516.977993847330026, 214.9014730243169993 ) ) ;
#97717=CARTESIAN_POINT ( 'NONE',  ( -6.560742263465000335, 1517.028034847769959, 205.0881926677770082 ) ) ;
#97729=CARTESIAN_POINT ( 'NONE',  ( -1.702754409475000008, 1517.014196759610059, 212.5856132281170119 ) ) ;
#97735=CARTESIAN_POINT ( 'NONE',  ( -7.708878413334149471, 1516.528448466100144, 211.3872135947860045 ) ) ;
#97736=CARTESIAN_POINT ( 'NONE',  ( -3.255809902135000211, 1516.837969789639828, 209.8792719553279937 ) ) ;
#97737=ORIENTED_EDGE ( 'NONE', *, *, #28818, .T. ) ;
#97748=CARTESIAN_POINT ( 'NONE',  ( -6.941100315875000426, 1516.858069504249897, 216.0654486236869900 ) ) ;
#97752=ORIENTED_EDGE ( 'NONE', *, *, #97548, .T. ) ;
#97753=CARTESIAN_POINT ( 'NONE',  ( -6.554764199395000546, 1516.786099423779888, 201.4062207291269999 ) ) ;
#97787=CARTESIAN_POINT ( 'NONE',  ( 12.33871145880999975, 1512.142158944850053, 223.9832163156410161 ) ) ;
#97822=ORIENTED_EDGE ( 'NONE', *, *, #104881, .T. ) ;
#97826=CARTESIAN_POINT ( 'NONE',  ( 5.789394662204999875, 1517.164987839469859, 210.8286437561770299 ) ) ;
#97833=CARTESIAN_POINT ( 'NONE',  ( -0.7526715882979990724, 1516.710624944440042, 201.4081970979170251 ) ) ;
#97845=B_SPLINE_CURVE_WITH_KNOTS ( 'NONE', 3,
 ( #94143, #17414, #51611, #667, #1217, #95808 ),
 .UNSPECIFIED., .F., .F.,
 ( 4, 2, 4 ),
 ( 1.219745808755950105E-06, 0.01184124321884439703, 0.02355706456992970321 ),
 .UNSPECIFIED. ) ;
#97855=CARTESIAN_POINT ( 'NONE',  ( 1.118903270415000151, 1517.003078582959688, 206.2405205581369785 ) ) ;
#97858=CARTESIAN_POINT ( 'NONE',  ( 0.4403324358131759930, 1517.051704035390003, 201.6347831756999938 ) ) ;
#97871=CARTESIAN_POINT ( 'NONE',  ( -1.123101616545000070, 1517.157901477309906, 214.9105372957470195 ) ) ;
#97873=CARTESIAN_POINT ( 'NONE',  ( 7.708979774182910027, 1516.532320736849897, 206.7210651042560130 ) ) ;
#97880=EDGE_CURVE ( 'NONE', #107968, #42578, #41340, .T. ) ;
#97905=DIRECTION ( 'NONE',  ( 0.7044160264027579110, -0.08715574274766998975, 0.7044160264027579110 ) ) ;
#97944=CARTESIAN_POINT ( 'NONE',  ( -6.952166420425000659, 1517.213554313520035, 207.4130983078469797 ) ) ;
#97965=CARTESIAN_POINT ( 'NONE',  ( 13.22750721609810398, 1513.553906385406208, 225.9068792231137195 ) ) ;
#97967=ORIENTED_EDGE ( 'NONE', *, *, #75513, .T. ) ;
#97974=CARTESIAN_POINT ( 'NONE',  ( 4.668127331444700268, 1508.551704406479985, 204.7884844211849895 ) ) ;
#97976=AXIS2_PLACEMENT_3D ( 'NONE', #83584, #24224, #58411 ) ;
#97985=CARTESIAN_POINT ( 'NONE',  ( -5.007588685045000432, 1516.804776704140068, 203.3466091393569855 ) ) ;
#98001=DIRECTION ( 'NONE',  ( -0.7071067811865490160, 0.000000000000000000, 0.7071067811865460184 ) ) ;
#98007=CARTESIAN_POINT ( 'NONE',  ( -7.304088287825000414, 1513.265135866609853, 201.5893727638369910 ) ) ;
#98022=CARTESIAN_POINT ( 'NONE',  ( 13.59434822483500049, 1512.526319173689899, 225.1381234417670214 ) ) ;
#98030=CARTESIAN_POINT ( 'NONE',  ( -1.717432486395000124, 1516.836638729160086, 206.8395443540670158 ) ) ;
#98054=B_SPLINE_CURVE_WITH_KNOTS ( 'NONE', 5,
 ( #108883, #48450, #30517, #40574, #82015, #82588 ),
 .UNSPECIFIED., .F., .F.,
 ( 6, 6 ),
 ( 0.000000000000000000, 1.000000000000000000 ),
 .UNSPECIFIED. ) ;
#98080=CARTESIAN_POINT ( 'NONE',  ( -5.513435588854999736, 1508.551704408389924, 216.1347675159770176 ) ) ;
#98088=CARTESIAN_POINT ( 'NONE',  ( 3.254401403604999743, 1516.919782530640077, 205.0791161293069820 ) ) ;
#98102=CARTESIAN_POINT ( 'NONE',  ( -1.701850495234999983, 1516.908147884120126, 210.2591426210370003 ) ) ;
#98129=CARTESIAN_POINT ( 'NONE',  ( -4.625693903144999730, 1517.042661899400173, 206.8353996064669786 ) ) ;
#98130=ORIENTED_EDGE ( 'NONE', *, *, #31043, .F. ) ;
#98148=CARTESIAN_POINT ( 'NONE',  ( -5.777745433405000242, 1516.908489800550115, 215.6797558528670038 ) ) ;
#98150=B_SPLINE_CURVE_WITH_KNOTS ( 'NONE', 3,
 ( #90611, #6063, #99554, #64338, #98461, #106855 ),
 .UNSPECIFIED., .F., .F.,
 ( 4, 2, 4 ),
 ( 0.000000000000000000, 0.5000000000000000000, 1.000000000000000000 ),
 .UNSPECIFIED. ) ;
#98155=CARTESIAN_POINT ( 'NONE',  ( -7.710610441124999603, 1516.594591938570147, 212.5759658869370128 ) ) ;
#98175=CARTESIAN_POINT ( 'NONE',  ( 1.120543697654999837, 1517.073005577650065, 205.0775260448770041 ) ) ;
#98180=CARTESIAN_POINT ( 'NONE',  ( -6.372167638625000130, 1511.069621805459974, 201.7253008890070021 ) ) ;
#98199=AXIS2_PLACEMENT_3D ( 'NONE', #54656, #62515, #104473 ) ;
#98208=VECTOR ( 'NONE', #73027, 1000.000000000000000 ) ;
#98215=CARTESIAN_POINT ( 'NONE',  ( -12.93225142166500063, 1513.362623229679912, 192.2350631226669861 ) ) ;
#98218=CARTESIAN_POINT ( 'NONE',  ( 3.452917022905000355, 1517.089216728169959, 202.1725802860869976 ) ) ;
#98225=CARTESIAN_POINT ( 'NONE',  ( 4.987078422726499483, 1508.551704408389924, 205.6342535031670025 ) ) ;
#98234=CARTESIAN_POINT ( 'NONE',  ( -7.594039287445000674, 1512.142919181319940, 211.3515775794370199 ) ) ;
#98241=( NAMED_UNIT ( * ) SI_UNIT ( $, .STERADIAN. ) SOLID_ANGLE_UNIT ( ) );
#98256=CARTESIAN_POINT ( 'NONE',  ( -1.121950782074999875, 1517.123342927159911, 214.1352753262870010 ) ) ;
#98263=CARTESIAN_POINT ( 'NONE',  ( 2.867803626105000170, 1516.994127245590107, 204.4971090729170271 ) ) ;
#98268=CARTESIAN_POINT ( 'NONE',  ( 6.329634364484999942, 1512.038636172079805, 217.3289309248769996 ) ) ;
#98276=CARTESIAN_POINT ( 'NONE',  ( -7.322709724964999722, 1516.596789218710001, 212.3828531017969965 ) ) ;
#98281=CARTESIAN_POINT ( 'NONE',  ( -7.719450415276570610, 1516.932212683830130, 209.1299851226509929 ) ) ;
#98282=CARTESIAN_POINT ( 'NONE',  ( 1.127928333405000094, 1516.989863902050047, 209.1117210464550169 ) ) ;
#98289=VECTOR ( 'NONE', #36532, 1000.000000000000114 ) ;
#98297=CARTESIAN_POINT ( 'NONE',  ( 0.7538707352880020807, 1516.719999691880048, 216.0603247549969979 ) ) ;
#98302=CARTESIAN_POINT ( 'NONE',  ( 5.003848121975000396, 1517.005755693489846, 201.7875176594370146 ) ) ;
#98319=ORIENTED_EDGE ( 'NONE', *, *, #93291, .T. ) ;
#98322=CARTESIAN_POINT ( 'NONE',  ( 5.513435558552499671, 1509.038615934029849, 201.6090957240569992 ) ) ;
#98337=EDGE_CURVE ( 'NONE', #108462, #5353, #27157, .T. ) ;
#98342=CARTESIAN_POINT ( 'NONE',  ( 12.67335156995190104, 1512.240709848930010, 224.2037181255240057 ) ) ;
#98371=VECTOR ( 'NONE', #66332, 1000.000000000000000 ) ;
#98379=VERTEX_POINT ( 'NONE', #77982 ) ;
#98383=CARTESIAN_POINT ( 'NONE',  ( -0.7350232362959980836, 1516.970035769810011, 211.4194755912870107 ) ) ;
#98385=CARTESIAN_POINT ( 'NONE',  ( -2.864326125434999870, 1516.826109302209943, 211.6149197999869784 ) ) ;
#98390=VERTEX_POINT ( 'NONE', #102062 ) ;
#98392=CARTESIAN_POINT ( 'NONE',  ( -7.330554171554999776, 1516.857992118400034, 201.7925428541169879 ) ) ;
#98396=CARTESIAN_POINT ( 'NONE',  ( -3.487592467065220081, 1508.551704408389924, 204.1347675093749956 ) ) ;
#98407=CARTESIAN_POINT ( 'NONE',  ( 3.269984781304999810, 1516.999105586269934, 210.8242519552970009 ) ) ;
#98412=CARTESIAN_POINT ( 'NONE',  ( 7.563688191785000292, 1510.983859056260144, 206.1910078925270113 ) ) ;
#98413=CARTESIAN_POINT ( 'NONE',  ( -2.881222795715000284, 1516.891731298979948, 206.6444723262370076 ) ) ;
#98415=CARTESIAN_POINT ( 'NONE',  ( -7.709151609294999652, 1516.538881398679905, 211.6739720840869836 ) ) ;
#98416=CARTESIAN_POINT ( 'NONE',  ( -2.935376417616495370, 1516.592453102976606, 202.2105020858446096 ) ) ;
#98430=CARTESIAN_POINT ( 'NONE',  ( -1.706797824074999914, 1517.164987839469859, 214.9112406324369999 ) ) ;
#98432=CARTESIAN_POINT ( 'NONE',  ( 7.711638320313230821, 1516.633846517499933, 208.0028055230160078 ) ) ;
#98450=VERTEX_POINT ( 'NONE', #69615 ) ;
#98461=CARTESIAN_POINT ( 'NONE',  ( -6.141424781052139181, 1511.655929346179391, 200.3276031877419427 ) ) ;
#98495=CARTESIAN_POINT ( 'NONE',  ( 7.722580314247720068, 1517.051704408590012, 209.5565402419049974 ) ) ;
#98501=CARTESIAN_POINT ( 'NONE',  ( 2.476170596904999854, 1516.819260244609950, 207.4047612206870213 ) ) ;
#98524=CARTESIAN_POINT ( 'NONE',  ( 12.03834750937141607, 1513.050501378461377, 225.7232701713909933 ) ) ;
#98531=CARTESIAN_POINT ( 'NONE',  ( 3.487587042568910167, 1508.884219106000046, 204.6305577925189993 ) ) ;
#98539=CARTESIAN_POINT ( 'NONE',  ( -2.488360667435000284, 1516.616791731099966, 203.3506968572170308 ) ) ;
#98548=CARTESIAN_POINT ( 'NONE',  ( -12.77505765355909872, 1512.281672892730057, 193.9892705280500138 ) ) ;
#98570=VECTOR ( 'NONE', #56859, 1000.000000000000114 ) ;
#98575=CARTESIAN_POINT ( 'NONE',  ( 14.66019551493499939, 1513.841826332629807, 225.4222558759669823 ) ) ;
#98583=CARTESIAN_POINT ( 'NONE',  ( -4.625693903144999730, 1517.042661899400173, 206.8353996064669786 ) ) ;
#98637=AXIS2_PLACEMENT_3D ( 'NONE', #10921, #2545, #66574 ) ;
#98638=CARTESIAN_POINT ( 'NONE',  ( -2.492130661305000050, 1516.778761582560037, 205.6761608547170113 ) ) ;
#98654=CARTESIAN_POINT ( 'NONE',  ( 3.462835627365000057, 1517.038650117239968, 210.2415636864969883 ) ) ;
#98672=CARTESIAN_POINT ( 'NONE',  ( -6.259133024435000081, 1514.370494773850169, 216.8656120519870001 ) ) ;
#98682=EDGE_CURVE ( 'NONE', #107607, #51438, #48997, .T. ) ;
#98687=CARTESIAN_POINT ( 'NONE',  ( -4.044319925355000400, 1517.073005577650065, 208.0013022344469960 ) ) ;
#98695=EDGE_CURVE ( 'NONE', #63015, #71163, #95823, .T. ) ;
#98698=CARTESIAN_POINT ( 'NONE',  ( -5.854887960802339641, 1510.764648358910108, 201.5757148928349807 ) ) ;
#98701=CARTESIAN_POINT ( 'NONE',  ( -5.650234538444452781, 1510.510563500882199, 201.5728936304679451 ) ) ;
#98705=CARTESIAN_POINT ( 'NONE',  ( -6.941100315875000426, 1516.858069504249897, 216.0654486236869900 ) ) ;
#98709=CARTESIAN_POINT ( 'NONE',  ( 2.759768239755020058, 1516.551696783219995, 216.8313331240459831 ) ) ;
#98710=CARTESIAN_POINT ( 'NONE',  ( 2.878693249144999466, 1516.766397346390022, 213.1495431961470217 ) ) ;
#98727=CARTESIAN_POINT ( 'NONE',  ( -2.878693287274999957, 1516.766397346390022, 205.0941487061870134 ) ) ;
#98756=CARTESIAN_POINT ( 'NONE',  ( 8.510893208398943699, 1511.398734635591836, 204.1579629377903302 ) ) ;
#98763=CARTESIAN_POINT ( 'NONE',  ( -7.477233281890912409, 1510.784366248438573, 215.2449024152596166 ) ) ;
#98766=CARTESIAN_POINT ( 'NONE',  ( -14.12475447096500147, 1513.169116394660023, 193.8258293473670051 ) ) ;
#98770=CARTESIAN_POINT ( 'NONE',  ( 2.290886266485000267, 1517.184383877180153, 201.7830921018669983 ) ) ;
#98773=CARTESIAN_POINT ( 'NONE',  ( 14.84895960063500020, 1511.957228877180114, 197.0446257365670135 ) ) ;
#98786=CARTESIAN_POINT ( 'NONE',  ( -7.621419158765000645, 1512.021995456199875, 211.6878531360469822 ) ) ;
#98796=CARTESIAN_POINT ( 'NONE',  ( 7.475494255215000550, 1511.623805160490065, 202.7254354214969965 ) ) ;
#98807=CARTESIAN_POINT ( 'NONE',  ( 5.005071008295000290, 1516.710692850270107, 216.4473877573669824 ) ) ;
#98815=CARTESIAN_POINT ( 'NONE',  ( 2.286446325635000054, 1517.042661899400173, 204.4961520670869959 ) ) ;
#98817=CARTESIAN_POINT ( 'NONE',  ( -0.7402208985179988820, 1516.992029636990083, 209.8751463226419958 ) ) ;
#98820=CARTESIAN_POINT ( 'NONE',  ( 6.338109897684999439, 1511.735270473999890, 216.7196367433270154 ) ) ;
#98831=CARTESIAN_POINT ( 'NONE',  ( 1.714334247185000049, 1516.699825673279975, 213.1484604498870112 ) ) ;
#98836=CARTESIAN_POINT ( 'NONE',  ( -7.709419779119449423, 1516.549122391340006, 210.7997296842460173 ) ) ;
#98837=CARTESIAN_POINT ( 'NONE',  ( -4.026614517785000125, 1516.699825673279975, 210.8361802174170236 ) ) ;
#98846=CARTESIAN_POINT ( 'NONE',  ( 7.559673304084999934, 1510.830536680500245, 205.9482437802269885 ) ) ;
#98849=CARTESIAN_POINT ( 'NONE',  ( 0.7533001353030019942, 1516.714320817460020, 216.4479181143769893 ) ) ;
#98854=CARTESIAN_POINT ( 'NONE',  ( -2.485217232065000115, 1516.534320418310244, 201.4128137944169907 ) ) ;
#98889=CARTESIAN_POINT ( 'NONE',  ( 13.64573737686789912, 1512.804203059180054, 224.4338647574110155 ) ) ;
#98893=CARTESIAN_POINT ( 'NONE',  ( 6.198157297588786641, 1516.723276579750518, 204.8982196523435846 ) ) ;
#98929=CARTESIAN_POINT ( 'NONE',  ( 2.881548424445000034, 1516.909589401870107, 211.4054166033970148 ) ) ;
#98931=CARTESIAN_POINT ( 'NONE',  ( -5.771797464315000070, 1516.647618671360078, 211.9976960644470125 ) ) ;
#98937=CARTESIAN_POINT ( 'NONE',  ( 2.290886266485000267, 1517.184383877180153, 201.7830921018669983 ) ) ;
#98952=CARTESIAN_POINT ( 'NONE',  ( 1.717139084115000047, 1516.949031626070109, 210.2396860569670025 ) ) ;
#98958=CARTESIAN_POINT ( 'NONE',  ( -3.462948834675000143, 1516.956048353049937, 206.8373194734570006 ) ) ;
#98974=CARTESIAN_POINT ( 'NONE',  ( 3.262264650305000124, 1516.633288330999903, 215.6694029015669969 ) ) ;
#98976=CARTESIAN_POINT ( 'NONE',  ( 7.709204607498650219, 1516.540906774789846, 207.3459979817129977 ) ) ;
#98984=LINE ( 'NONE', #4933, #70089 ) ;
#98994=CARTESIAN_POINT ( 'NONE',  ( -3.415238448984999842, 1511.775527460079957, 212.5370843810869985 ) ) ;
#98999=CARTESIAN_POINT ( 'NONE',  ( -5.139225489064998875, 1511.037966505499980, 201.4363886582769965 ) ) ;
#99004=LINE ( 'NONE', #29072, #8566 ) ;
#99030=ORIENTED_EDGE ( 'NONE', *, *, #108128, .T. ) ;
#99038=CARTESIAN_POINT ( 'NONE',  ( -7.580298022105069755, 1511.034527886640262, 215.0658449916730035 ) ) ;
#99042=CARTESIAN_POINT ( 'NONE',  ( 1.119592181715000079, 1516.958737650239982, 207.9859471464170326 ) ) ;
#99054=CARTESIAN_POINT ( 'NONE',  ( -15.21196350663329966, 1512.378201925209851, 222.0999656735410213 ) ) ;
#99055=CARTESIAN_POINT ( 'NONE',  ( -5.513435595168334480, 1508.783371651738207, 216.5758637223831329 ) ) ;
#99070=CARTESIAN_POINT ( 'NONE',  ( 4.987081042841619904, 1508.551704408389924, 205.1632167381339968 ) ) ;
#99079=CARTESIAN_POINT ( 'NONE',  ( 4.611879685325000366, 1516.858533673840157, 204.4999481076869756 ) ) ;
#99087=DIRECTION ( 'NONE',  ( -1.238073365138532047E-30, 1.000000000000000000, -6.123233995736639079E-17 ) ) ;
#99168=CARTESIAN_POINT ( 'NONE',  ( 9.638115859575000499, 1517.051704408389924, 214.4931927712770232 ) ) ;
#99175=CARTESIAN_POINT ( 'NONE',  ( -3.460101890015000237, 1516.812923327049930, 205.0932153474469715 ) ) ;
#99181=AXIS2_PLACEMENT_3D ( 'NONE', #98994, #48633, #66545 ) ;
#99191=CARTESIAN_POINT ( 'NONE',  ( -7.713648872314999849, 1516.710624944440042, 209.8745175203999906 ) ) ;
#99198=LINE ( 'NONE', #49925, #64156 ) ;
#99205=CARTESIAN_POINT ( 'NONE',  ( 16.30010422171099904, 1514.508970265533890, 194.3992361457187599 ) ) ;
#99217=CARTESIAN_POINT ( 'NONE',  ( 3.260357128764999946, 1517.133889586189980, 201.3971135232069969 ) ) ;
#99218=CARTESIAN_POINT ( 'NONE',  ( 4.610079833424999940, 1516.713079096360161, 207.9883289669969884 ) ) ;
#99230=CARTESIAN_POINT ( 'NONE',  ( -6.288919133997779021, 1510.947107049704073, 201.6929532012474340 ) ) ;
#99238=CARTESIAN_POINT ( 'NONE',  ( 3.261007131564999995, 1516.596789218710001, 216.4445556570670135 ) ) ;
#99241=CARTESIAN_POINT ( 'NONE',  ( 2.255244433210603638, 1516.528169492436291, 216.8307170402573831 ) ) ;
#99242=CARTESIAN_POINT ( 'NONE',  ( 1.134357970594999987, 1516.744381837270112, 213.1504571913470159 ) ) ;
#99245=CARTESIAN_POINT ( 'NONE',  ( 3.487587102937319994, 1509.038630944639863, 213.6090953401219963 ) ) ;
#99260=CARTESIAN_POINT ( 'NONE',  ( -6.560742263465000335, 1517.028034847769959, 205.0881926677770082 ) ) ;
#99278=CARTESIAN_POINT ( 'NONE',  ( 3.330134165755000097, 1515.051704408389924, 204.7920544413669859 ) ) ;
#99289=CARTESIAN_POINT ( 'NONE',  ( 7.943217798846315958, 1511.827406192408489, 205.9421500790769528 ) ) ;
#99295=ORIENTED_EDGE ( 'NONE', *, *, #88439, .F. ) ;
#99297=CARTESIAN_POINT ( 'NONE',  ( -7.550704986171106192, 1510.491946833609973, 214.7158011863163836 ) ) ;
#99298=EDGE_CURVE ( 'NONE', #47608, #3729, #42470, .T. ) ;
#99305=CARTESIAN_POINT ( 'NONE',  ( 2.483949940595000516, 1517.156142772249950, 202.1710124019969896 ) ) ;
#99308=CARTESIAN_POINT ( 'NONE',  ( 16.48353617723500264, 1512.679339245399888, 197.4676877011670229 ) ) ;
#99341=CARTESIAN_POINT ( 'NONE',  ( -4.615017365965000451, 1516.987478262539980, 215.6816440265270103 ) ) ;
#99347=VECTOR ( 'NONE', #90373, 1000.000000000000114 ) ;
#99349=CARTESIAN_POINT ( 'NONE',  ( 3.447264348965000558, 1516.858765657450249, 205.6607986404769974 ) ) ;
#99351=CARTESIAN_POINT ( 'NONE',  ( 2.297629621054999571, 1516.970035769810011, 209.8568691683980205 ) ) ;
#99355=CARTESIAN_POINT ( 'NONE',  ( 6.252266454184999489, 1511.741868877540128, 217.9101624594169948 ) ) ;
#99365=CARTESIAN_POINT ( 'NONE',  ( 2.877744946244999991, 1516.723920667490120, 213.7309102736070088 ) ) ;
#99371=CARTESIAN_POINT ( 'NONE',  ( -7.709465792554129671, 1516.550879573519751, 210.7818539985390203 ) ) ;
#99372=CARTESIAN_POINT ( 'NONE',  ( -2.863787893864999656, 1516.788317650260069, 210.8382387120070121 ) ) ;
#99383=DIRECTION ( 'NONE',  ( 0.000000000000000000, -1.000000000000000000, 6.123233995736769734E-17 ) ) ;
#99387=CARTESIAN_POINT ( 'NONE',  ( -3.259729335964999919, 1517.119374999550018, 216.4589997383470177 ) ) ;
#99392=CARTESIAN_POINT ( 'NONE',  ( -2.291676311554999845, 1516.534976163889951, 201.8006522243570089 ) ) ;
#99399=CARTESIAN_POINT ( 'NONE',  ( 8.652278223286959502, 1511.434805660039956, 203.7377894773300113 ) ) ;
#99411=PLANE ( 'NONE',  #63943 ) ;
#99412=ADVANCED_FACE ( 'NONE', ( #28997 ), #11100, .F. ) ;
#99469=CARTESIAN_POINT ( 'NONE',  ( 4.626591867355000609, 1517.096587378560116, 210.8266407735670214 ) ) ;
#99472=CARTESIAN_POINT ( 'NONE',  ( -4.997573825325000385, 1516.742629295279812, 212.5803724681170195 ) ) ;
#99477=CARTESIAN_POINT ( 'NONE',  ( -5.005700239535000762, 1516.732530461250008, 202.1838802717869896 ) ) ;
#99492=CARTESIAN_POINT ( 'NONE',  ( -1.117840124865000062, 1516.949031626070109, 210.8389850543470061 ) ) ;
#99498=CARTESIAN_POINT ( 'NONE',  ( 7.703229018584999643, 1511.126521646420088, 203.6801735634869885 ) ) ;
#99499=CARTESIAN_POINT ( 'NONE',  ( 3.445201488374999954, 1516.743010792419909, 207.4064848398570291 ) ) ;
#99505=CARTESIAN_POINT ( 'NONE',  ( 7.012921545474999796, 1508.551704408389924, 209.1218459511669892 ) ) ;
#99517=CARTESIAN_POINT ( 'NONE',  ( 7.718763505904999711, 1516.905946377369901, 216.0642002436470079 ) ) ;
#99519=CARTESIAN_POINT ( 'NONE',  ( 7.713327774496799627, 1516.698364169800016, 208.2833887839009890 ) ) ;
#99551=CARTESIAN_POINT ( 'NONE',  ( -4.824495029074999941, 1511.382391139620040, 200.6581036276869838 ) ) ;
#99554=CARTESIAN_POINT ( 'NONE',  ( -5.716900218388740740, 1511.491070486171338, 200.3735384854518315 ) ) ;
#99588=CARTESIAN_POINT ( 'NONE',  ( -8.771942286537230515, 1511.501325589009866, 214.9071201462460010 ) ) ;
#99593=CARTESIAN_POINT ( 'NONE',  ( -3.269984819434999856, 1516.999105586269934, 207.4194399470370058 ) ) ;
#99603=CARTESIAN_POINT ( 'NONE',  ( -14.92433373228269922, 1512.160613316490071, 221.5430094126030269 ) ) ;
#99609=EDGE_LOOP ( 'NONE', ( #27631, #75940, #82565, #60990 ) ) ;
#99627=CARTESIAN_POINT ( 'NONE',  ( 5.773668814845000163, 1516.734985836460055, 205.0832084693769843 ) ) ;
#99645=VECTOR ( 'NONE', #3879, 1000.000000000000000 ) ;
#99649=CARTESIAN_POINT ( 'NONE',  ( -7.692900486654999703, 1514.487275757750012, 203.3032714771670157 ) ) ;
#99721=CARTESIAN_POINT ( 'NONE',  ( -3.112702537996912433, 1511.889608914253358, 201.1973302697319070 ) ) ;
#99729=CARTESIAN_POINT ( 'NONE',  ( -7.724423432224999608, 1517.122088787240045, 205.6676733166769964 ) ) ;
#99736=ORIENTED_EDGE ( 'NONE', *, *, #86544, .T. ) ;
#99745=CARTESIAN_POINT ( 'NONE',  ( 7.727327114725000001, 1517.232977404109988, 210.8318586907270173 ) ) ;
#99758=CARTESIAN_POINT ( 'NONE',  ( -6.470331913555000369, 1513.423632355040127, 216.5900188188570041 ) ) ;
#99772=CARTESIAN_POINT ( 'NONE',  ( 0.7391219670640019057, 1517.130100026000036, 202.1721425974470208 ) ) ;
#99773=CARTESIAN_POINT ( 'NONE',  ( -2.881325412095000260, 1517.003078582959688, 208.0029426616869728 ) ) ;
#99783=CARTESIAN_POINT ( 'NONE',  ( 10.96015508933500016, 1514.690994518219895, 225.0317485278669949 ) ) ;
#99786=CARTESIAN_POINT ( 'NONE',  ( -5.773315255633579390, 1510.559702728003685, 201.5815081783346727 ) ) ;
#99792=CARTESIAN_POINT ( 'NONE',  ( -7.329930051325000306, 1516.881930554049859, 216.8399805996670011 ) ) ;
#99795=CARTESIAN_POINT ( 'NONE',  ( 5.213129316145000303, 1514.517422889960017, 200.4652853224170030 ) ) ;
#99797=CARTESIAN_POINT ( 'NONE',  ( -1.119717754394999876, 1517.038650117239968, 212.5846815975970117 ) ) ;
#99800=CARTESIAN_POINT ( 'NONE',  ( 4.429741920660830168, 1508.551704408389924, 213.9240898912200066 ) ) ;
#99815=CARTESIAN_POINT ( 'NONE',  ( 3.446329775655000205, 1516.812046502680005, 206.2422037788969931 ) ) ;
#99846=CARTESIAN_POINT ( 'NONE',  ( 8.184191755800993562, 1511.478973222094055, 205.1565754550810254 ) ) ;
#99859=CARTESIAN_POINT ( 'NONE',  ( 4.615017327834999961, 1516.987478262539980, 202.5620478758069964 ) ) ;
#99862=CARTESIAN_POINT ( 'NONE',  ( 15.85140261003499873, 1511.863761374039996, 197.3804798592670124 ) ) ;
#99895=CARTESIAN_POINT ( 'NONE',  ( 0.01171160595180150039, 1516.939568781210028, 215.6786969668069958 ) ) ;
#99897=AXIS2_PLACEMENT_3D ( 'NONE', #34628, #78860, #53108 ) ;
#99905=CARTESIAN_POINT ( 'NONE',  ( -3.267603553834999897, 1516.858171774179937, 205.8687047948669999 ) ) ;
#99907=CARTESIAN_POINT ( 'NONE',  ( 3.455495833855000143, 1516.939877939420057, 209.1085718841020196 ) ) ;
#99912=CARTESIAN_POINT ( 'NONE',  ( 6.262845557134999908, 1511.198876514819858, 216.5713750547470227 ) ) ;
#99921=CARTESIAN_POINT ( 'NONE',  ( -2.479246885834999858, 1516.983612918759945, 213.1658362778269691 ) ) ;
#99925=CARTESIAN_POINT ( 'NONE',  ( -7.709535243742100086, 1516.553531807379841, 210.7548730175080038 ) ) ;
#99926=CARTESIAN_POINT ( 'NONE',  ( -6.548200625775000283, 1516.632821972880038, 210.2524534341069966 ) ) ;
#99942=CARTESIAN_POINT ( 'NONE',  ( -5.003848160104999998, 1517.005755693489846, 216.4561742428970206 ) ) ;
#99947=CARTESIAN_POINT ( 'NONE',  ( 2.871580388595000422, 1517.129577905929864, 202.1716309988170224 ) ) ;
#99948=CARTESIAN_POINT ( 'NONE',  ( -16.28235098596499952, 1514.570049710740022, 223.9522021028669769 ) ) ;
#99953=CARTESIAN_POINT ( 'NONE',  ( 7.591975344036550055, 1510.802068165409992, 203.6262312139739947 ) ) ;
#99993=B_SPLINE_CURVE_WITH_KNOTS ( 'NONE', 3,
 ( #39190, #66639, #57131, #30238, #91258, #91800, #14538, #100740, #64973, #23494, #24024, #31899, #65529, #58224, #98548, #22366, #48727, #6142, #108049, #92347, #82309, #48171, #81194, #5607, #40853, #32464, #40300, #21817, #74483, #15620, #107505, #90696, #108610, #100212, #57686, #15079, #13983, #31345, #39760, #49273, #83401, #6698, #75028, #4512, #47613, #109179, #38644, #13423, #81737, #5045, #85595, #67733, #94007, #50381, #9460 ),
 .UNSPECIFIED., .F., .F.,
 ( 4, 3, 3, 3, 3, 3, 3, 3, 3, 3, 3, 3, 3, 3, 3, 3, 3, 3, 4 ),
 ( 9.902195898180000455, 10.17210527305359946, 10.45530577770680125, 10.70141353110000004, 11.00396970308290001, 11.32322756685609910, 11.52456852350000105, 11.84989040654409997, 12.16242387770059885, 12.38020728900000123, 12.74551463658920092, 13.12275145097450135, 13.53252099856520019, 13.95359103768650044, 14.40783883234479923, 14.91487510226109947, 15.44821056776079971, 15.94145638524880049, 16.40090783169999966 ),
 .UNSPECIFIED. ) ;
#100009=VERTEX_POINT ( 'NONE', #77391 ) ;
#100028=CARTESIAN_POINT ( 'NONE',  ( 3.268235720634999897, 1516.890356958860139, 211.9874346545169885 ) ) ;
#100032=CARTESIAN_POINT ( 'NONE',  ( 7.724423394095000894, 1517.122088787240045, 212.5760185856570104 ) ) ;
#100042=CARTESIAN_POINT ( 'NONE',  ( 1.708747624254999931, 1517.213554313520035, 202.1696795498070003 ) ) ;
#100055=LINE ( 'NONE', #73780, #20562 ) ;
#100061=CARTESIAN_POINT ( 'NONE',  ( 0.7579843820170020230, 1516.883361325900069, 211.4083188566570186 ) ) ;
#100069=CARTESIAN_POINT ( 'NONE',  ( -0.7579263249019989601, 1516.927039499179955, 207.4176752179770347 ) ) ;
#100073=EDGE_CURVE ( 'NONE', #71004, #97290, #19613, .T. ) ;
#100076=DIRECTION ( 'NONE',  ( 0.000000000000000000, -6.123233995736769734E-17, -1.000000000000000000 ) ) ;
#100085=CARTESIAN_POINT ( 'NONE',  ( 7.512750208045280154, 1509.038615934079871, 214.6352815289239970 ) ) ;
#100090=CARTESIAN_POINT ( 'NONE',  ( -3.452917061035000401, 1517.089216728169959, 216.0711116162470091 ) ) ;
#100093=CARTESIAN_POINT ( 'NONE',  ( -8.181958980964999739, 1517.051704408389924, 206.0868810637969943 ) ) ;
#100157=CARTESIAN_POINT ( 'NONE',  ( -8.275210849650859402, 1511.570327478370018, 214.9577656342009959 ) ) ;
#100163=CARTESIAN_POINT ( 'NONE',  ( 2.286472886424999906, 1516.883361325900069, 208.3638615500849767 ) ) ;
#100193=CARTESIAN_POINT ( 'NONE',  ( 4.487358438102120317, 1509.034524880150002, 205.3201215594939981 ) ) ;
#100199=CARTESIAN_POINT ( 'NONE',  ( -4.987078454533489413, 1508.551704408389924, 205.6342615457560044 ) ) ;
#100201=CARTESIAN_POINT ( 'NONE',  ( -3.460101890015000237, 1516.812923327049930, 205.0932153474469715 ) ) ;
#100204=CARTESIAN_POINT ( 'NONE',  ( 15.13257540405220070, 1512.281672892730057, 196.3467883166729848 ) ) ;
#100205=VECTOR ( 'NONE', #87835, 1000.000000000000114 ) ;
#100212=CARTESIAN_POINT ( 'NONE',  ( -13.70533116771989945, 1512.850289815999986, 193.8128379569050139 ) ) ;
#100216=EDGE_CURVE ( 'NONE', #42670, #76843, #13703, .T. ) ;
#100267=ORIENTED_EDGE ( 'NONE', *, *, #23852, .T. ) ;
#100280=ORIENTED_EDGE ( 'NONE', *, *, #92850, .F. ) ;
#100293=CARTESIAN_POINT ( 'NONE',  ( -4.330155983108352480, 1511.419855273161829, 200.8197880651785852 ) ) ;
#100298=CARTESIAN_POINT ( 'NONE',  ( 7.710610402995000001, 1516.594591938570147, 205.6677260153969939 ) ) ;
#100312=CARTESIAN_POINT ( 'NONE',  ( -6.548200625775000283, 1516.632821972880038, 210.2524534341069966 ) ) ;
#100324=VERTEX_POINT ( 'NONE', #86478 ) ;
#100340=CARTESIAN_POINT ( 'NONE',  ( -4.617490504904999682, 1516.685667699390024, 201.7969310139470167 ) ) ;
#100341=CARTESIAN_POINT ( 'NONE',  ( -2.879318455905000018, 1516.995911393979895, 208.3865093923290033 ) ) ;
#100360=CARTESIAN_POINT ( 'NONE',  ( -4.035536263215000474, 1517.086065052259983, 216.8453260496270047 ) ) ;
#100362=AXIS2_PLACEMENT_3D ( 'NONE', #66419, #64772, #107288 ) ;
#100366=CARTESIAN_POINT ( 'NONE',  ( 6.560742225334999844, 1517.028034847769959, 213.1554992345569701 ) ) ;
#100370=CARTESIAN_POINT ( 'NONE',  ( 3.910140106688379635, 1508.551704408389924, 213.9552835937910231 ) ) ;
#100384=CARTESIAN_POINT ( 'NONE',  ( -7.336844680545000053, 1517.106845464700200, 205.6683011064770312 ) ) ;
#100404=CARTESIAN_POINT ( 'NONE',  ( -13.22747438852011292, 1513.553889449568032, 192.3368110773319586 ) ) ;
#100411=CARTESIAN_POINT ( 'NONE',  ( 7.910095025013141878, 1511.948749218533067, 206.0626124326618651 ) ) ;
#100414=B_SPLINE_CURVE_WITH_KNOTS ( 'NONE', 5,
 ( #64340, #106858, #72732, #3890, #37468, #4428 ),
 .UNSPECIFIED., .F., .F.,
 ( 6, 6 ),
 ( 0.000000000000000000, 1.000000000000000000 ),
 .UNSPECIFIED. ) ;
#100418=EDGE_LOOP ( 'NONE', ( #27333, #4302, #24916, #76491, #17101, #23610, #4091, #98319 ) ) ;
#100427=CARTESIAN_POINT ( 'NONE',  ( 7.328049280255000575, 1516.809497469189864, 202.5664528150769854 ) ) ;
#100430=CARTESIAN_POINT ( 'NONE',  ( 15.71561344153500350, 1514.030803186779849, 194.0252525622669850 ) ) ;
#100444=CARTESIAN_POINT ( 'NONE',  ( -7.883416877324999739, 1512.215430505229961, 212.0555133921270112 ) ) ;
#100456=ORIENTED_EDGE ( 'NONE', *, *, #60045, .T. ) ;
#100461=CARTESIAN_POINT ( 'NONE',  ( 1.709358663124999955, 1516.542957540330008, 216.0554336257470140 ) ) ;
#100462=CARTESIAN_POINT ( 'NONE',  ( -8.389626007570329946, 1511.399590460235004, 213.7199506810841569 ) ) ;
#100470=CARTESIAN_POINT ( 'NONE',  ( -4.042417815834999928, 1516.904492006980036, 205.6736390534169914 ) ) ;
#100471=ORIENTED_EDGE ( 'NONE', *, *, #39179, .F. ) ;
#100472=CARTESIAN_POINT ( 'NONE',  ( 4.623892060624999800, 1517.066898074209803, 209.8584071487349831 ) ) ;
#100476=CARTESIAN_POINT ( 'NONE',  ( 6.911190382705000523, 1512.677556571470177, 217.1831025208769859 ) ) ;
#100485=CARTESIAN_POINT ( 'NONE',  ( 5.784638319815000429, 1516.939574742129935, 213.7356083271170064 ) ) ;
#100489=CARTESIAN_POINT ( 'NONE',  ( 6.032864527508810859, 1508.551565390810083, 216.2881064761960204 ) ) ;
#100490=CARTESIAN_POINT ( 'NONE',  ( -3.253301419385000504, 1516.790374942449944, 210.2573062871869922 ) ) ;
#100505=CARTESIAN_POINT ( 'NONE',  ( -2.872836660654999985, 1517.158319634930194, 216.8472181024670249 ) ) ;
#100509=EDGE_LOOP ( 'NONE', ( #22822, #77844, #25495, #104123 ) ) ;
#100510=CARTESIAN_POINT ( 'NONE',  ( 7.328049280255000575, 1516.809497469189864, 202.5664528150769854 ) ) ;
#100511=CARTESIAN_POINT ( 'NONE',  ( -16.62677417856500028, 1512.592133792520144, 221.2813269351669874 ) ) ;
#100529=CARTESIAN_POINT ( 'NONE',  ( -4.333389548141039604, 1508.551704407329908, 213.7899627404379999 ) ) ;
#100547=CARTESIAN_POINT ( 'NONE',  ( 6.224497175254511738, 1516.718921113260649, 204.9371257324691555 ) ) ;
#100579=CARTESIAN_POINT ( 'NONE',  ( -0.7353365779029981120, 1516.995911393979895, 212.0011643880069698 ) ) ;
#100582=CARTESIAN_POINT ( 'NONE',  ( -2.478306858074999841, 1516.938330505699923, 212.5844667883370107 ) ) ;
#100589=CARTESIAN_POINT ( 'NONE',  ( -6.556651409415000131, 1516.858146885269889, 202.5689485651570010 ) ) ;
#100604=CARTESIAN_POINT ( 'NONE',  ( 2.299656316094999653, 1516.843453247299749, 211.5982966343670171 ) ) ;
#100608=CARTESIAN_POINT ( 'NONE',  ( -2.494020320564999782, 1516.876240617270014, 206.8389307488369866 ) ) ;
#100626=CARTESIAN_POINT ( 'NONE',  ( -4.615644842514999624, 1517.009964551830080, 216.0692237534070159 ) ) ;
#100701=CARTESIAN_POINT ( 'NONE',  ( 2.486220101774999858, 1516.939658295650133, 209.1086089184300079 ) ) ;
#100732=CARTESIAN_POINT ( 'NONE',  ( 1.703779605225000049, 1517.057265928030120, 205.0766634521770015 ) ) ;
#100740=CARTESIAN_POINT ( 'NONE',  ( -12.45742386984340122, 1512.169469372310004, 194.1709192302429869 ) ) ;
#100775=VECTOR ( 'NONE', #47751, 1000.000000000000000 ) ;
#100780=EDGE_CURVE ( 'NONE', #96332, #94274, #80712, .T. ) ;
#100819=LINE ( 'NONE', #34183, #92941 ) ;
#100820=CARTESIAN_POINT ( 'NONE',  ( 15.91746618545751524, 1512.594959757391052, 198.1541272149443671 ) ) ;
#100822=CARTESIAN_POINT ( 'NONE',  ( -3.141753572004903461, 1511.860476876181110, 201.1893397601683944 ) ) ;
#100827=CARTESIAN_POINT ( 'NONE',  ( -0.7574260232259989456, 1516.837969789639828, 205.8660360680970030 ) ) ;
#100837=FACE_OUTER_BOUND ( 'NONE', #66752, .T. ) ;
#100841=CARTESIAN_POINT ( 'NONE',  ( 7.725990161824999980, 1517.181921232829836, 211.6070516194370157 ) ) ;
#100867=ORIENTED_EDGE ( 'NONE', *, *, #31531, .T. ) ;
#100868=CARTESIAN_POINT ( 'NONE',  ( -5.779603138255000161, 1516.738222552470233, 201.4074744291170020 ) ) ;
#100869=CARTESIAN_POINT ( 'NONE',  ( -6.563915562015000482, 1517.184063036290127, 207.9975562766469750 ) ) ;
#100872=CARTESIAN_POINT ( 'NONE',  ( 2.957482190928379495, 1512.146734775097912, 217.0093202360658609 ) ) ;
#100887=CARTESIAN_POINT ( 'NONE',  ( 3.454119916704999849, 1516.594591938570147, 216.8324563732270178 ) ) ;
#100892=CARTESIAN_POINT ( 'NONE',  ( 5.009478067315000338, 1516.886345593249871, 213.7343532441369973 ) ) ;
#100910=CARTESIAN_POINT ( 'NONE',  ( -5.011367984924999242, 1516.974592746400049, 205.6720686163770324 ) ) ;
#100958=CARTESIAN_POINT ( 'NONE',  ( -15.01814803086499950, 1514.214451716350140, 194.3960746180669901 ) ) ;
#100961=CARTESIAN_POINT ( 'NONE',  ( -13.78858225216500166, 1513.492015765619954, 222.2033214031669957 ) ) ;
#100963=CARTESIAN_POINT ( 'NONE',  ( -2.487103457664999961, 1516.577434278289957, 202.5755431900869894 ) ) ;
#100966=CARTESIAN_POINT ( 'NONE',  ( 16.44145556193499758, 1512.902436350919970, 197.5299575732669837 ) ) ;
#100973=VERTEX_POINT ( 'NONE', #94053 ) ;
#100991=CARTESIAN_POINT ( 'NONE',  ( 8.473068888075001581, 1511.778199792620171, 203.0330132217169989 ) ) ;
#100999=CARTESIAN_POINT ( 'NONE',  ( -2.483949978725000118, 1517.156142772249950, 216.0726795003369887 ) ) ;
#101000=CARTESIAN_POINT ( 'NONE',  ( -8.480656650225677495, 1511.395875706868765, 213.9949865275974616 ) ) ;
#101004=LINE ( 'NONE', #51177, #76070 ) ;
#101006=CARTESIAN_POINT ( 'NONE',  ( 3.446942071715000111, 1516.842852731759876, 205.8545543269370057 ) ) ;
#101008=CARTESIAN_POINT ( 'NONE',  ( 0.7468175155120010400, 1517.006509894990131, 209.1147170949500094 ) ) ;
#101021=CARTESIAN_POINT ( 'NONE',  ( -3.449149233875000053, 1516.947419719950176, 213.7456339395970133 ) ) ;
#101025=CARTESIAN_POINT ( 'NONE',  ( 5.513199787613100256, 1509.038617475950105, 216.6345962046710270 ) ) ;
#101026=CARTESIAN_POINT ( 'NONE',  ( 2.882325979385000014, 1516.969638403840008, 210.8235757905769674 ) ) ;
#101031=ORIENTED_EDGE ( 'NONE', *, *, #37375, .F. ) ;
#101045=CARTESIAN_POINT ( 'NONE',  ( -1.710004586925000236, 1516.557392317769882, 202.5758445815369839 ) ) ;
#101123=CARTESIAN_POINT ( 'NONE',  ( -2.865911554774999814, 1516.906233342200039, 212.5838411289170153 ) ) ;
#101125=CARTESIAN_POINT ( 'NONE',  ( 7.495834450094876367, 1517.015741767610280, 209.4130272268053261 ) ) ;
#101131=CARTESIAN_POINT ( 'NONE',  ( -0.01126495432349849946, 1516.939530130779985, 202.1773791897269916 ) ) ;
#101146=CARTESIAN_POINT ( 'NONE',  ( 1.717432448265000078, 1516.836638729160086, 211.4041475482669910 ) ) ;
#101151=CARTESIAN_POINT ( 'NONE',  ( -1.717432486395000124, 1516.836638729160086, 206.8395443540670158 ) ) ;
#101165=CARTESIAN_POINT ( 'NONE',  ( -2.287084308194999860, 1517.068517094990057, 214.1351209316169957 ) ) ;
#101168=CARTESIAN_POINT ( 'NONE',  ( 3.455377977254999955, 1516.627618683580067, 216.0573038954169931 ) ) ;
#101204=LINE ( 'NONE', #32909, #32486 ) ;
#101237=CARTESIAN_POINT ( 'NONE',  ( 4.037050997585000189, 1516.939819969850078, 209.1086255745840106 ) ) ;
#101243=ORIENTED_EDGE ( 'NONE', *, *, #4240, .T. ) ;
#101271=CARTESIAN_POINT ( 'NONE',  ( -2.297085753945000253, 1516.718889242609976, 205.0950684461469962 ) ) ;
#101365=CARTESIAN_POINT ( 'NONE',  ( -6.950214971414999887, 1517.129577905929864, 206.2502655435069983 ) ) ;
#101375=CARTESIAN_POINT ( 'NONE',  ( -1.906498070525230022E-08, 1509.051704408389924, 202.1089243866269953 ) ) ;
#101379=CARTESIAN_POINT ( 'NONE',  ( 0.01323701367210150005, 1516.939658295650133, 211.6080660720070341 ) ) ;
#101404=CARTESIAN_POINT ( 'NONE',  ( 5.761714419953206878, 1516.919864955462117, 213.9826803693840986 ) ) ;
#101410=CARTESIAN_POINT ( 'NONE',  ( 4.034280915654999689, 1517.049325831759916, 202.1735242262370207 ) ) ;
#101411=CARTESIAN_POINT ( 'NONE',  ( -3.455495871984999745, 1516.939877939420057, 209.1351200182310208 ) ) ;
#101433=CARTESIAN_POINT ( 'NONE',  ( 0.01010282929720150019, 1516.939452820819952, 216.8414868732370167 ) ) ;
#101436=CARTESIAN_POINT ( 'NONE',  ( 17.05938516367379876, 1517.051704408300111, 223.0487112149370148 ) ) ;
#101437=CARTESIAN_POINT ( 'NONE',  ( -0.1447896363496347094, 1516.980486180143544, 216.8425613695660275 ) ) ;
#101438=CARTESIAN_POINT ( 'NONE',  ( 5.784008635194999748, 1516.911981270829983, 214.1231845985469988 ) ) ;
#101441=CARTESIAN_POINT ( 'NONE',  ( 4.832613776139130124, 1508.551704408389924, 212.6094311844759943 ) ) ;
#101446=CARTESIAN_POINT ( 'NONE',  ( -4.329791528864999961, 1515.051704408389924, 205.7917117663469924 ) ) ;
#101456=CARTESIAN_POINT ( 'NONE',  ( 6.935133380425000382, 1516.613881697390070, 205.8602099992770036 ) ) ;
#101480=CARTESIAN_POINT ( 'NONE',  ( -14.16484771644310925, 1514.105042352133523, 192.5349129913882393 ) ) ;
#101500=CARTESIAN_POINT ( 'NONE',  ( -14.96248399886500202, 1513.868118914750085, 193.8718938829669867 ) ) ;
#101506=CARTESIAN_POINT ( 'NONE',  ( 0.7386049046750020608, 1517.122674412569950, 202.5597518628069906 ) ) ;
#101510=CARTESIAN_POINT ( 'NONE',  ( 14.92003712803500015, 1512.136030808819896, 196.7378588390670018 ) ) ;
#101533=CARTESIAN_POINT ( 'NONE',  ( 5.924854864274999855, 1514.639648807489948, 201.3510662795570170 ) ) ;
#101539=DIRECTION ( 'NONE',  ( 0.7071067811865474617, -5.176495448588656087E-16, 0.7071067811865474617 ) ) ;
#101543=CARTESIAN_POINT ( 'NONE',  ( 6.554764161265000055, 1516.786099423779888, 216.8374711732070068 ) ) ;
#101549=CARTESIAN_POINT ( 'NONE',  ( 6.935457925184999262, 1516.627618683580067, 205.6664679548470076 ) ) ;
#101555=CARTESIAN_POINT ( 'NONE',  ( 7.908505681124999853, 1514.005261957200219, 216.3707927467769991 ) ) ;
#101566=AXIS2_PLACEMENT_3D ( 'NONE', #81816, #5118, #39274 ) ;
#101567=CARTESIAN_POINT ( 'NONE',  ( -3.448206916814999801, 1516.904492006980036, 213.1642637479369853 ) ) ;
#101568=EDGE_CURVE ( 'NONE', #64503, #13404, #94488, .T. ) ;
#101572=CARTESIAN_POINT ( 'NONE',  ( 6.827653871725639867, 1508.551704612109916, 215.5772939192580111 ) ) ;
#101573=CARTESIAN_POINT ( 'NONE',  ( 4.625693865015000128, 1517.042661899400173, 211.4082922958669997 ) ) ;
#101586=CARTESIAN_POINT ( 'NONE',  ( 12.30406194763500061, 1511.972232048389969, 224.1970232450669869 ) ) ;
#101587=CARTESIAN_POINT ( 'NONE',  ( -7.329930051325000306, 1516.881930554049859, 216.8399805996670011 ) ) ;
#101593=CARTESIAN_POINT ( 'NONE',  ( -2.292307268505000106, 1516.548716157039962, 202.1882291110970300 ) ) ;
#101616=LINE ( 'NONE', #24903, #30634 ) ;
#101649=CARTESIAN_POINT ( 'NONE',  ( 7.458082240553069120, 1510.848430439774347, 202.9305636724023429 ) ) ;
#101670=CARTESIAN_POINT ( 'NONE',  ( 2.297085715815000206, 1516.718889242609976, 213.1486234561869821 ) ) ;
#101671=CARTESIAN_POINT ( 'NONE',  ( 5.496430521294999316, 1510.805212328559946, 216.6808561328170128 ) ) ;
#101677=CARTESIAN_POINT ( 'NONE',  ( 7.326795523374999952, 1516.760434454289907, 203.3416138547669902 ) ) ;
#101691=CARTESIAN_POINT ( 'NONE',  ( -13.96015163203214549, 1516.660421270692041, 191.9693043941119299 ) ) ;
#101693=CARTESIAN_POINT ( 'NONE',  ( 3.462620818104999998, 1516.938330505699923, 211.6001527901769919 ) ) ;
#101699=CARTESIAN_POINT ( 'NONE',  ( -1.715109485185000171, 1516.963431999339946, 208.3866188148990091 ) ) ;
#101716=CARTESIAN_POINT ( 'NONE',  ( 6.559168636745000391, 1516.960844870249957, 214.1244393295569921 ) ) ;
#101720=CARTESIAN_POINT ( 'NONE',  ( 6.556022194504999234, 1516.833525648419936, 216.0623193043769845 ) ) ;
#101776=CARTESIAN_POINT ( 'NONE',  ( -8.126234285584999384, 1514.923664147150021, 202.9950997886369635 ) ) ;
#101800=CARTESIAN_POINT ( 'NONE',  ( 3.455495833855000143, 1516.939877939420057, 209.1085718841020196 ) ) ;
#101809=CARTESIAN_POINT ( 'NONE',  ( -15.29936285970580023, 1512.951873711589997, 222.9557858335909941 ) ) ;
#101832=CARTESIAN_POINT ( 'NONE',  ( 4.997250153905000047, 1516.727068157269969, 205.8570671527170077 ) ) ;
#101835=CARTESIAN_POINT ( 'NONE',  ( 14.98757060048970047, 1513.799047785590119, 194.4265915126370032 ) ) ;
#101873=FACE_OUTER_BOUND ( 'NONE', #61281, .T. ) ;
#101883=CARTESIAN_POINT ( 'NONE',  ( 2.492130623175000448, 1516.778761582560037, 212.5675310476169955 ) ) ;
#101901=CARTESIAN_POINT ( 'NONE',  ( 15.90990255763500016, 1516.814170398969964, 193.9190501556669801 ) ) ;
#101930=CARTESIAN_POINT ( 'NONE',  ( -3.268235758764999943, 1516.890356958860139, 206.2562572478169898 ) ) ;
#101938=CARTESIAN_POINT ( 'NONE',  ( -16.35769669196890419, 1514.438069590152509, 223.7531373634772649 ) ) ;
#101942=CARTESIAN_POINT ( 'NONE',  ( -7.321193745875000047, 1516.534976163889951, 211.4135222436570132 ) ) ;
#101973=CARTESIAN_POINT ( 'NONE',  ( 3.452917022905000355, 1517.089216728169959, 202.1725802860869976 ) ) ;
#101974=CARTESIAN_POINT ( 'NONE',  ( 3.261652286895000419, 1516.939580991450157, 209.1085619926769823 ) ) ;
#101978=CARTESIAN_POINT ( 'NONE',  ( 3.196833426707265335, 1511.813436676099627, 217.0699578229602196 ) ) ;
#102010=LINE ( 'NONE', #52746, #60967 ) ;
#102017=CARTESIAN_POINT ( 'NONE',  ( -4.624099329465000352, 1516.962555622980062, 205.8665050058069994 ) ) ;
#102023=( BOUNDED_CURVE ( )  B_SPLINE_CURVE ( 3, ( #81111, #6616, #110177, #40769 ),
 .UNSPECIFIED., .F., .F. ) 
 B_SPLINE_CURVE_WITH_KNOTS ( ( 4, 4 ),
 ( 1.144746442793614261, 1.570758305569332380 ),
 .UNSPECIFIED. ) 
 CURVE ( )  GEOMETRIC_REPRESENTATION_ITEM ( )  RATIONAL_B_SPLINE_CURVE ( ( 1.000000000000000000, 0.9849332539703330447, 0.9849332539703330447, 1.000000000000000000 ) ) 
 REPRESENTATION_ITEM ( '' )  );
#102060=CARTESIAN_POINT ( 'NONE',  ( -5.513200305162849979, 1508.884117426709963, 216.6305509556679851 ) ) ;
#102062=CARTESIAN_POINT ( 'NONE',  ( 5.513435558014999849, 1508.551704408389924, 216.1347675157070114 ) ) ;
#102071=CARTESIAN_POINT ( 'NONE',  ( -2.488360667435000284, 1516.616791731099966, 203.3506968572170308 ) ) ;
#102100=CARTESIAN_POINT ( 'NONE',  ( 6.787530778265000286, 1514.254015528269974, 201.2664419476070066 ) ) ;
#102109=CARTESIAN_POINT ( 'NONE',  ( 3.454119916704999849, 1516.594591938570147, 216.8324563732270178 ) ) ;
#102110=CARTESIAN_POINT ( 'NONE',  ( -8.384987537200094820, 1511.400228778148630, 213.7058500936460632 ) ) ;
#102113=CARTESIAN_POINT ( 'NONE',  ( 7.396545043095000160, 1511.069621805459974, 202.7496783316070150 ) ) ;
#102116=CARTESIAN_POINT ( 'NONE',  ( -0.01323705180209850014, 1516.939658295650133, 206.6356258303270010 ) ) ;
#102121=CARTESIAN_POINT ( 'NONE',  ( 7.651189237105000096, 1514.325389163589989, 214.8282438176370022 ) ) ;
#102129=CARTESIAN_POINT ( 'NONE',  ( -0.7369042090349989804, 1517.080322339569875, 214.1333973382469935 ) ) ;
#102133=CARTESIAN_POINT ( 'NONE',  ( 7.166260500400270850, 1508.551565390750284, 215.1547094865549923 ) ) ;
#102134=CARTESIAN_POINT ( 'NONE',  ( 0.7578857918350010436, 1516.872851364150165, 211.6022732247369902 ) ) ;
#102154=CARTESIAN_POINT ( 'NONE',  ( 5.776491095245000373, 1516.858301627840092, 203.3390965304970166 ) ) ;
#102177=CARTESIAN_POINT ( 'NONE',  ( -3.801734761035370447, 1509.034524749680031, 213.6092044152910034 ) ) ;
#102190=EDGE_CURVE ( 'NONE', #21931, #71163, #15519, .T. ) ;
#102209=CARTESIAN_POINT ( 'NONE',  ( -5.381311933963230487, 1511.468585895311890, 200.7968825339673913 ) ) ;
#102238=CARTESIAN_POINT ( 'NONE',  ( 7.709253415549203403, 1516.542698387791233, 206.5079181198552760 ) ) ;
#102241=CARTESIAN_POINT ( 'NONE',  ( 6.559168636745000391, 1516.960844870249957, 214.1244393295569921 ) ) ;
#102242=FACE_OUTER_BOUND ( 'NONE', #49527, .T. ) ;
#102246=CARTESIAN_POINT ( 'NONE',  ( 3.449777315724999571, 1516.974592746400049, 204.1104779853070283 ) ) ;
#102260=CARTESIAN_POINT ( 'NONE',  ( 4.625693865015000128, 1517.042661899400173, 211.4082922958669997 ) ) ;
#102264=CARTESIAN_POINT ( 'NONE',  ( -6.951517170504999399, 1517.194816588360027, 207.9969518818670053 ) ) ;
#102280=CARTESIAN_POINT ( 'NONE',  ( 2.877113070465000089, 1516.697242742309982, 214.1184881303969973 ) ) ;
#102283=CARTESIAN_POINT ( 'NONE',  ( -7.717505791104999346, 1516.857914730730045, 216.8393517232070167 ) ) ;
#102308=CARTESIAN_POINT ( 'NONE',  ( -4.487249792034999629, 1509.038615934169911, 205.6342535031670025 ) ) ;
#102363=CARTESIAN_POINT ( 'NONE',  ( -2.879318455905000018, 1516.995911393979895, 208.3865093923290033 ) ) ;
#102373=CARTESIAN_POINT ( 'NONE',  ( -15.30997868661039973, 1512.715996828740117, 222.6464017490669960 ) ) ;
#102396=CARTESIAN_POINT ( 'NONE',  ( 0.7356989345870019736, 1517.020847257979995, 205.6609797614169963 ) ) ;
#102442=CARTESIAN_POINT ( 'NONE',  ( 6.948321705865000197, 1517.049325831759916, 213.1561268858870051 ) ) ;
#102484=CARTESIAN_POINT ( 'NONE',  ( -6.949574985774999547, 1517.102359858469754, 205.8627441332170065 ) ) ;
#102492=CARTESIAN_POINT ( 'NONE',  ( -15.90990259576500065, 1512.830284628050094, 220.0820010595669771 ) ) ;
#102496=CARTESIAN_POINT ( 'NONE',  ( 5.788097227154999302, 1517.099836525840146, 211.6039138304569747 ) ) ;
#102512=DIRECTION ( 'NONE',  ( -0.4999999999998399058, 0.7071067811867739472, 0.4999999999998399058 ) ) ;
#102520=ORIENTED_EDGE ( 'NONE', *, *, #37776, .T. ) ;
#102521=CARTESIAN_POINT ( 'NONE',  ( 5.001338628314999646, 1516.911981270829983, 203.3378372969070256 ) ) ;
#102522=CARTESIAN_POINT ( 'NONE',  ( 1.715109447055000125, 1516.963431999339946, 209.8570730874349977 ) ) ;
#102544=CARTESIAN_POINT ( 'NONE',  ( 2.073027880074009399, 1516.528002108337205, 216.8307126571504284 ) ) ;
#102563=CARTESIAN_POINT ( 'NONE',  ( -3.462620856235000044, 1516.938330505699923, 206.6435391121569864 ) ) ;
#102583=CARTESIAN_POINT ( 'NONE',  ( -14.75867395745958000, 1514.537581216768785, 192.8458395396856986 ) ) ;
#102607=CARTESIAN_POINT ( 'NONE',  ( 7.325541787135000149, 1516.710692850270107, 204.1167749238070144 ) ) ;
#102630=CARTESIAN_POINT ( 'NONE',  ( -1.701027861004999808, 1516.937508036699910, 211.6166039682370013 ) ) ;
#102634=CARTESIAN_POINT ( 'NONE',  ( 8.191860436744999419, 1512.696049264740168, 202.1234250822469960 ) ) ;
#102639=EDGE_CURVE ( 'NONE', #17126, #33889, #5110, .T. ) ;
#102643=CARTESIAN_POINT ( 'NONE',  ( 0.7526715501680020237, 1516.710624944440042, 216.8354948044169817 ) ) ;
#102644=CARTESIAN_POINT ( 'NONE',  ( -8.115358832489173224, 1511.538143004863514, 212.8694838649076928 ) ) ;
#102650=CARTESIAN_POINT ( 'NONE',  ( 3.445685077385000294, 1516.778761582560037, 206.6297153089269898 ) ) ;
#102656=CARTESIAN_POINT ( 'NONE',  ( 7.468172848634999639, 1513.423632355050131, 215.5921778456470008 ) ) ;
#102665=CARTESIAN_POINT ( 'NONE',  ( -4.613762395014999740, 1516.939574742129935, 214.9064842900469898 ) ) ;
#102670=CARTESIAN_POINT ( 'NONE',  ( -7.321455911854999776, 1516.545806094630279, 211.6076919691270177 ) ) ;
#102680=ADVANCED_FACE ( 'NONE', ( #43043 ), #66877, .F. ) ;
#102686=CARTESIAN_POINT ( 'NONE',  ( 0.7526715501680020237, 1516.710624944440042, 216.8354948044169817 ) ) ;
#102691=CARTESIAN_POINT ( 'NONE',  ( 1.123101578415000024, 1517.157901477309906, 203.3331546065870157 ) ) ;
#102712=CARTESIAN_POINT ( 'NONE',  ( -3.910153998790829810, 1508.551704408439946, 213.9552835279250189 ) ) ;
#102743=B_SPLINE_SURFACE_WITH_KNOTS ( 'NONE', 5, 5, ( 
 ( #28031, #1760, #44303, #62220, #45415, #27475 ),
 ( #43196, #61129, #9570, #35898, #79558, #61666 ),
 ( #2856, #17957, #60565, #103069, #19624, #26940 ),
 ( #95242, #104742, #77892, #96347, #95790, #36979 ),
 ( #105295, #28586, #78446, #36430, #34781, #18506 ),
 ( #52704, #77348, #26370, #86838, #87401, #94685 ) ),
 .UNSPECIFIED., .F., .F., .F.,
 ( 6, 6 ),
 ( 6, 6 ),
 ( 5.893388896116969811, 9.819930328983028645 ),
 ( -0.0002947352030313690231, 0.5000000000000000000 ),
 .UNSPECIFIED. ) ;
#102745=PRODUCT_DEFINITION ( 'UNKNOWN', '', #33320, #2079 ) ;
#102774=CARTESIAN_POINT ( 'NONE',  ( 0.01306000193830150063, 1516.939762005280045, 213.7404293621069939 ) ) ;
#102775=CARTESIAN_POINT ( 'NONE',  ( 7.500384403881742656, 1516.975677308576451, 209.2665120174619631 ) ) ;
#102781=CARTESIAN_POINT ( 'NONE',  ( -5.782749439735000330, 1516.858301627840092, 203.3453548368569841 ) ) ;
#102782=ADVANCED_FACE ( 'NONE', ( #35362 ), #41824, .F. ) ;
#102788=CARTESIAN_POINT ( 'NONE',  ( -5.649719788644999241, 1514.243099272629934, 216.7708803706970002 ) ) ;
#102795=CARTESIAN_POINT ( 'NONE',  ( 2.493073829755000137, 1516.826109302209943, 211.9861720575370043 ) ) ;
#102801=CARTESIAN_POINT ( 'NONE',  ( 5.000329995535000016, 1516.770163853809890, 208.3657552043160024 ) ) ;
#102816=CARTESIAN_POINT ( 'NONE',  ( 0.4363688355183920065, 1517.051704408389924, 201.4773664372389987 ) ) ;
#102819=CARTESIAN_POINT ( 'NONE',  ( 5.008848199894999631, 1516.858456333729919, 214.1219297979669989 ) ) ;
#102822=CARTESIAN_POINT ( 'NONE',  ( -6.554151464375000735, 1516.906641539930206, 216.4536580562070185 ) ) ;
#102831=UNCERTAINTY_MEASURE_WITH_UNIT (LENGTH_MEASURE( 1.000000000000000082E-05 ), #80354, 'distance_accuracy_value', 'NONE');
#102833=DIRECTION ( 'NONE',  ( -0.5224574779879248565, 0.7067418228238977473, 0.4770263929449307105 ) ) ;
#102856=CIRCLE ( 'NONE', #68943, 1.000000000039231285 ) ;
#102859=CARTESIAN_POINT ( 'NONE',  ( -2.521927849235349850, 1516.537893464249919, 201.4127202309169888 ) ) ;
#102883=ORIENTED_EDGE ( 'NONE', *, *, #91241, .T. ) ;
#102901=CARTESIAN_POINT ( 'NONE',  ( 7.012921545474999796, 1508.551704408389924, 203.6084103740869864 ) ) ;
#102903=CARTESIAN_POINT ( 'NONE',  ( 2.879318417774999972, 1516.995911393979895, 209.8571825100049750 ) ) ;
#102920=CARTESIAN_POINT ( 'NONE',  ( 6.550870144104999682, 1516.727502608469877, 208.3674577492799926 ) ) ;
#102936=CARTESIAN_POINT ( 'NONE',  ( 3.446942071715000111, 1516.842852731759876, 205.8545543269370057 ) ) ;
#102982=EDGE_CURVE ( 'NONE', #4206, #74270, #85669, .T. ) ;
#102991=CARTESIAN_POINT ( 'NONE',  ( -7.711550716115000093, 1516.630499592039996, 213.1573366827869904 ) ) ;
#103032=CARTESIAN_POINT ( 'NONE',  ( 4.609673241434999902, 1516.754149861460064, 205.8564388142570181 ) ) ;
#103039=DIRECTION ( 'NONE',  ( 1.794299266459999922E-16, 1.000000000000000000, 1.181975866886321963E-16 ) ) ;
#103041=CARTESIAN_POINT ( 'NONE',  ( -16.27599028281260019, 1514.537600263860895, 223.8805438227635989 ) ) ;
#103045=CARTESIAN_POINT ( 'NONE',  ( 2.299656316094999653, 1516.843453247299749, 211.5982966343670171 ) ) ;
#103065=LINE ( 'NONE', #94680, #72483 ) ;
#103069=CARTESIAN_POINT ( 'NONE',  ( 6.725623893241880147, 1508.728101229370168, 201.9181371664530218 ) ) ;
#103074=CARTESIAN_POINT ( 'NONE',  ( -7.331183129075000693, 1516.882217593000178, 202.1801186797769674 ) ) ;
#103075=CARTESIAN_POINT ( 'NONE',  ( -2.486220139904999904, 1516.939658295650133, 209.1350829839039989 ) ) ;
#103078=CARTESIAN_POINT ( 'NONE',  ( 3.000838584243140428, 1512.040964529592429, 217.0177385286994820 ) ) ;
#103079=VERTEX_POINT ( 'NONE', #2211 ) ;
#103098=CARTESIAN_POINT ( 'NONE',  ( -3.487592469391230132, 1509.038615938009798, 204.6345961782960217 ) ) ;
#103100=ADVANCED_FACE ( 'NONE', ( #88663 ), #83825, .F. ) ;
#103114=CARTESIAN_POINT ( 'NONE',  ( -15.71561347966500222, 1514.030803186779849, 224.2184393400669933 ) ) ;
#103119=CARTESIAN_POINT ( 'NONE',  ( 7.321193707744999557, 1516.534976163889951, 206.8301696586770220 ) ) ;
#103135=CARTESIAN_POINT ( 'NONE',  ( -3.077691755255000050, 1511.730395268069969, 201.3186441269170075 ) ) ;
#103167=CARTESIAN_POINT ( 'NONE',  ( -5.781490582474999584, 1516.807958722750072, 202.5702025453269925 ) ) ;
#103189=CARTESIAN_POINT ( 'NONE',  ( 3.461995158685000185, 1516.906233342200039, 211.9877574868770012 ) ) ;
#103192=CARTESIAN_POINT ( 'NONE',  ( 6.490306520025000303, 1514.605246816799763, 201.0943966606369884 ) ) ;
#103198=CARTESIAN_POINT ( 'NONE',  ( -7.449529122645000001, 1511.198876514819858, 215.3846915273670106 ) ) ;
#103202=CARTESIAN_POINT ( 'NONE',  ( -0.7403206051589980019, 1517.139320148880188, 216.8467205834170102 ) ) ;
#103209=CARTESIAN_POINT ( 'NONE',  ( 7.709032137684999952, 1516.534320418310244, 206.6366287381669906 ) ) ;
#103215=CARTESIAN_POINT ( 'NONE',  ( 6.867779371605000627, 1512.132770473900109, 216.2848484671970084 ) ) ;
#103225=CARTESIAN_POINT ( 'NONE',  ( 5.007588646914999941, 1516.804776704140068, 214.8970827629769644 ) ) ;
#103230=CARTESIAN_POINT ( 'NONE',  ( -4.995994825704999975, 1516.665179208830068, 211.6114635085770033 ) ) ;
#103247=CARTESIAN_POINT ( 'NONE',  ( -5.782749439735000330, 1516.858301627840092, 203.3453548368569841 ) ) ;
#103270=DIRECTION ( 'NONE',  ( -1.000000000000000000, 0.000000000000000000, 0.000000000000000000 ) ) ;
#103292=AXIS2_PLACEMENT_3D ( 'NONE', #44625, #102833, #2081 ) ;
#103328=CARTESIAN_POINT ( 'NONE',  ( -4.998515195425000002, 1516.787536375099990, 213.1617432482970003 ) ) ;
#103337=CARTESIAN_POINT ( 'NONE',  ( 0.7376675027960020170, 1517.104497701820037, 203.3349981924270082 ) ) ;
#103339=CARTESIAN_POINT ( 'NONE',  ( -2.714430944004193158, 1517.051704408389696, 217.0111434691034731 ) ) ;
#103352=CARTESIAN_POINT ( 'NONE',  ( 2.879956924955000108, 1516.827328999679821, 212.3743765858270081 ) ) ;
#103356=CARTESIAN_POINT ( 'NONE',  ( -2.297629659184999618, 1516.970035769810011, 208.3868227339359862 ) ) ;
#103371=CARTESIAN_POINT ( 'NONE',  ( -6.550389470255000290, 1516.755758396839838, 214.1281755516169767 ) ) ;
#103374=CARTESIAN_POINT ( 'NONE',  ( 1.708092266164999984, 1516.523379810429788, 216.8305916180169959 ) ) ;
#103376=ORIENTED_EDGE ( 'NONE', *, *, #105503, .T. ) ;
#103379=ORIENTED_EDGE ( 'NONE', *, *, #17874, .T. ) ;
#103382=CARTESIAN_POINT ( 'NONE',  ( 8.274182124064189736, 1511.569910118449798, 203.2859663394350207 ) ) ;
#103399=DIRECTION ( 'NONE',  ( 0.7384854939282339270, -4.128709092058508552E-17, -0.6742693640212139572 ) ) ;
#103413=CARTESIAN_POINT ( 'NONE',  ( -1.013215592032840062, 1516.657104395810165, 201.4095985828120092 ) ) ;
#103419=ORIENTED_EDGE ( 'NONE', *, *, #60946, .F. ) ;
#103432=EDGE_CURVE ( 'NONE', #54193, #98450, #1771, .T. ) ;
#103450=CARTESIAN_POINT ( 'NONE',  ( -4.364199663720353506, 1509.032014613822184, 213.2377092680158341 ) ) ;
#103453=EDGE_CURVE ( 'NONE', #107968, #47285, #40723, .T. ) ;
#103462=CARTESIAN_POINT ( 'NONE',  ( 6.563915523884999992, 1517.184063036290127, 210.2461356256870033 ) ) ;
#103471=CARTESIAN_POINT ( 'NONE',  ( -15.19269324566649892, 1513.356256558869973, 223.4054110361780090 ) ) ;
#103480=CARTESIAN_POINT ( 'NONE',  ( -2.879318455905000018, 1516.995911393979895, 208.3865093923290033 ) ) ;
#103482=CARTESIAN_POINT ( 'NONE',  ( -6.520293482274176711, 1509.032998982614345, 216.3821516759590509 ) ) ;
#103485=ORIENTED_EDGE ( 'NONE', *, *, #33693, .F. ) ;
#103488=DIRECTION ( 'NONE',  ( -0.02616798426359480748, 0.9993150019884422530, -0.02616798426359490809 ) ) ;
#103500=CARTESIAN_POINT ( 'NONE',  ( -7.724423432224999608, 1517.122088787240045, 205.6676733166769964 ) ) ;
#103503=CARTESIAN_POINT ( 'NONE',  ( -3.956111812109641690, 1516.693880335214544, 202.7485082001233820 ) ) ;
#103518=DIRECTION ( 'NONE',  ( -1.000000000000000000, 0.000000000000000000, 0.000000000000000000 ) ) ;
#103521=CARTESIAN_POINT ( 'NONE',  ( -4.031142389804999837, 1516.929569650079884, 214.1322689334670031 ) ) ;
#103553=CARTESIAN_POINT ( 'NONE',  ( -0.7360974767499980365, 1517.045004075700035, 213.1642344714070134 ) ) ;
#103564=ORIENTED_EDGE ( 'NONE', *, *, #35346, .T. ) ;
#103595=DIRECTION ( 'NONE',  ( 0.5224574779878928821, 0.7067418228236548305, -0.4770263929453257834 ) ) ;
#103598=CARTESIAN_POINT ( 'NONE',  ( -6.477828314561669742, 1516.676423271974500, 212.9199659827493463 ) ) ;
#103604=CARTESIAN_POINT ( 'NONE',  ( 6.933879402874999265, 1516.560253536979872, 206.6353711893569880 ) ) ;
#103612=DIRECTION ( 'NONE',  ( -0.7071067811865490160, 0.000000000000000000, 0.7071067811865461294 ) ) ;
#103618=CARTESIAN_POINT ( 'NONE',  ( 6.950214933285000285, 1517.129577905929864, 211.9934263588270085 ) ) ;
#103630=EDGE_CURVE ( 'NONE', #19958, #47285, #19278, .T. ) ;
#103647=CARTESIAN_POINT ( 'NONE',  ( 5.002593359325000044, 1516.960844870249957, 202.5626772953570196 ) ) ;
#103648=CARTESIAN_POINT ( 'NONE',  ( 7.337297311985000015, 1517.135701590510052, 209.8615382079770200 ) ) ;
#103654=CARTESIAN_POINT ( 'NONE',  ( 4.115863297784077446, 1509.032014613820820, 213.4860455958220768 ) ) ;
#103669=CARTESIAN_POINT ( 'NONE',  ( -6.160280215534999826, 1511.773927532309926, 200.4817730439669958 ) ) ;
#103686=CARTESIAN_POINT ( 'NONE',  ( -15.38132089836499894, 1512.167884426309911, 221.9700943965670206 ) ) ;
#103691=CARTESIAN_POINT ( 'NONE',  ( 6.546039395294999785, 1516.565291103010168, 206.8289057630870218 ) ) ;
#103744=CARTESIAN_POINT ( 'NONE',  ( -1.712644754285000070, 1516.636036526019780, 204.1262224792070015 ) ) ;
#103769=CARTESIAN_POINT ( 'NONE',  ( 5.012938863775000087, 1517.051603658920158, 211.6026598552170128 ) ) ;
#103772=CARTESIAN_POINT ( 'NONE',  ( 7.100264587344999434, 1513.939092156090055, 201.4023203369069961 ) ) ;
#103779=CARTESIAN_POINT ( 'NONE',  ( -7.597790811225000773, 1511.735270473989885, 215.4599558679070128 ) ) ;
#103783=CARTESIAN_POINT ( 'NONE',  ( -6.942354311545000378, 1516.905946377369901, 216.8406094761369900 ) ) ;
#103792=CARTESIAN_POINT ( 'NONE',  ( -3.268859434184999913, 1516.922519270759949, 206.6438591998669949 ) ) ;
#103798=CARTESIAN_POINT ( 'NONE',  ( -5.513203518415759952, 1509.038617455540134, 201.6090956557640084 ) ) ;
#103808=CARTESIAN_POINT ( 'NONE',  ( 7.333070134885000257, 1516.955859323880077, 214.9008457440070003 ) ) ;
#103810=CARTESIAN_POINT ( 'NONE',  ( 5.556441548075099490, 1511.478393686179970, 217.5010704010999802 ) ) ;
#103812=CARTESIAN_POINT ( 'NONE',  ( 5.012317068235000228, 1517.020727862619879, 211.9902797687369969 ) ) ;
#103819=DIRECTION ( 'NONE',  ( 0.9996573249755574819, 0.02617694830786557875, 0.000000000000000000 ) ) ;
#103828=CARTESIAN_POINT ( 'NONE',  ( -4.621267922064999922, 1516.830644417779922, 204.1223895416970038 ) ) ;
#103842=VECTOR ( 'NONE', #37084, 1000.000000000000114 ) ;
#103856=CARTESIAN_POINT ( 'NONE',  ( 7.886115920484915165, 1512.218044538973345, 206.1805372229848956 ) ) ;
#103858=ORIENTED_EDGE ( 'NONE', *, *, #100216, .T. ) ;
#103865=CARTESIAN_POINT ( 'NONE',  ( 7.501993457708461044, 1516.814304245379844, 208.6975970486373626 ) ) ;
#103887=EDGE_CURVE ( 'NONE', #36271, #74608, #72158, .T. ) ;
#103889=CARTESIAN_POINT ( 'NONE',  ( -1.906499846882070084E-08, 1515.051704408389924, 209.1218459511669892 ) ) ;
#103902=CARTESIAN_POINT ( 'NONE',  ( -2.866857931135000204, 1516.951766529250108, 213.1652121904069759 ) ) ;
#103903=CARTESIAN_POINT ( 'NONE',  ( 4.059671795525000348, 1511.437978678640093, 217.3350408236069882 ) ) ;
#103909=CARTESIAN_POINT ( 'NONE',  ( 6.550389432124999800, 1516.755758396839838, 204.1155163507169732 ) ) ;
#103911=CARTESIAN_POINT ( 'NONE',  ( -3.173602190014999991, 1510.830536680500245, 201.5621726280170094 ) ) ;
#103916=CARTESIAN_POINT ( 'NONE',  ( -7.396545081224999763, 1511.069621805459974, 215.4940135707269917 ) ) ;
#103924=CARTESIAN_POINT ( 'NONE',  ( -1.701027861004999808, 1516.937508036699910, 211.6166039682370013 ) ) ;
#103929=CARTESIAN_POINT ( 'NONE',  ( 0.7402208603880020554, 1516.992029636990083, 208.3685455796920110 ) ) ;
#103940=CARTESIAN_POINT ( 'NONE',  ( -6.774723970312340526, 1511.035127054690065, 200.8105558358980147 ) ) ;
#103944=CARTESIAN_POINT ( 'NONE',  ( -3.257220640824999958, 1517.040132827679827, 214.9086836491569841 ) ) ;
#103947=CARTESIAN_POINT ( 'NONE',  ( -1.126138146715000010, 1517.208444099459939, 216.8485306577670144 ) ) ;
#103955=CARTESIAN_POINT ( 'NONE',  ( 5.513435553965000402, 1508.551704408389924, 202.1089243864769855 ) ) ;
#103963=CARTESIAN_POINT ( 'NONE',  ( 5.513435558014999849, 1508.551704408389924, 216.1347675157070114 ) ) ;
#104005=DIRECTION ( 'NONE',  ( -1.000000000000000000, 0.000000000000000000, 0.000000000000000000 ) ) ;
#104017=CARTESIAN_POINT ( 'NONE',  ( -2.804945344961504716, 1516.554483488290998, 201.4122858543795189 ) ) ;
#104026=CARTESIAN_POINT ( 'NONE',  ( 2.493697040924999886, 1516.977201124959947, 210.2401991861970032 ) ) ;
#104029=CARTESIAN_POINT ( 'NONE',  ( -4.487249792034999629, 1509.038615934239942, 212.6094383991670043 ) ) ;
#104035=CARTESIAN_POINT ( 'NONE',  ( -15.06905043960169976, 1513.645442089240078, 223.6837085688980267 ) ) ;
#104043=CARTESIAN_POINT ( 'NONE',  ( 0.7374508827770021036, 1516.978425811520083, 207.9881927911069965 ) ) ;
#104059=CARTESIAN_POINT ( 'NONE',  ( 6.934528529765000116, 1516.588006113850042, 206.2478870805069846 ) ) ;
#104061=DIRECTION ( 'NONE',  ( 0.02616798426359480748, 0.9993150019884422530, -0.02616798426359490809 ) ) ;
#104077=FACE_OUTER_BOUND ( 'NONE', #7235, .T. ) ;
#104079=CARTESIAN_POINT ( 'NONE',  ( 7.721907888235000073, 1517.026025493960105, 214.1263215447669950 ) ) ;
#104111=CARTESIAN_POINT ( 'NONE',  ( 5.784638319815000429, 1516.939574742129935, 213.7356083271170064 ) ) ;
#104112=ADVANCED_FACE ( 'NONE', ( #42370 ), #107923, .T. ) ;
#104123=ORIENTED_EDGE ( 'NONE', *, *, #96009, .T. ) ;
#104156=CARTESIAN_POINT ( 'NONE',  ( 1.701027822874999984, 1516.937508036699910, 206.6270879340970055 ) ) ;
#104169=CARTESIAN_POINT ( 'NONE',  ( 7.724732408895000013, 1517.133889586189980, 212.3822030989969960 ) ) ;
#104183=EDGE_LOOP ( 'NONE', ( #110129, #15132, #20146, #22708 ) ) ;
#104198=CARTESIAN_POINT ( 'NONE',  ( 5.777745395274999751, 1516.908489800550115, 202.5639360494670029 ) ) ;
#104199=CARTESIAN_POINT ( 'NONE',  ( 3.462835627365000057, 1517.038650117239968, 210.2415636864969883 ) ) ;
#104236=CARTESIAN_POINT ( 'NONE',  ( 11.75640697503499865, 1511.791180387469922, 224.3022927925669876 ) ) ;
#104245=CARTESIAN_POINT ( 'NONE',  ( -5.787477032644999575, 1517.070197312179971, 206.2521524731670013 ) ) ;
#104262=ORIENTED_EDGE ( 'NONE', *, *, #44206, .T. ) ;
#104263=CARTESIAN_POINT ( 'NONE',  ( 5.650234563753527617, 1510.510563522158918, 216.6707982693055499 ) ) ;
#104269=CARTESIAN_POINT ( 'NONE',  ( -4.987078454554999318, 1508.551704408389924, 205.6342535004969818 ) ) ;
#104288=CARTESIAN_POINT ( 'NONE',  ( -7.260542987912549151, 1508.878901734200099, 215.8879478474800067 ) ) ;
#104298=CARTESIAN_POINT ( 'NONE',  ( -5.008848238024999233, 1516.858456333729919, 204.1217621043670079 ) ) ;
#104313=DIRECTION ( 'NONE',  ( -0.7384854939282339270, 0.000000000000000000, 0.6742693640212139572 ) ) ;
#104317=CARTESIAN_POINT ( 'NONE',  ( 2.492443650904999863, 1516.793978928989873, 212.3737347995770222 ) ) ;
#104325=ORIENTED_EDGE ( 'NONE', *, *, #108950, .F. ) ;
#104327=CARTESIAN_POINT ( 'NONE',  ( -7.538480533405000017, 1511.326779185850000, 215.2911934950269881 ) ) ;
#104339=CARTESIAN_POINT ( 'NONE',  ( -7.724732447025000504, 1517.133889586189980, 205.8614888033369823 ) ) ;
#104345=CARTESIAN_POINT ( 'NONE',  ( -7.266089503534879590, 1509.032013814719903, 202.3522253410079941 ) ) ;
#104355=CARTESIAN_POINT ( 'NONE',  ( -6.937965698444999774, 1516.732530461250008, 214.1275461716370216 ) ) ;
#104357=CARTESIAN_POINT ( 'NONE',  ( 6.127742252161359815, 1511.645100227929788, 217.9168819886610038 ) ) ;
#104359=CARTESIAN_POINT ( 'NONE',  ( -3.446942109845000157, 1516.842852731759876, 212.3891375753969726 ) ) ;
#104378=CARTESIAN_POINT ( 'NONE',  ( 1.705466410464999916, 1517.120861839400050, 204.1076508302870138 ) ) ;
#104421=LINE ( 'NONE', #27714, #34297 ) ;
#104428=CARTESIAN_POINT ( 'NONE',  ( 7.883543492515000750, 1512.115618635729788, 206.1708866102069919 ) ) ;
#104437=FACE_OUTER_BOUND ( 'NONE', #94799, .T. ) ;
#104454=CARTESIAN_POINT ( 'NONE',  ( 2.489617538345000103, 1516.665179208830068, 214.1178407578070164 ) ) ;
#104455=CARTESIAN_POINT ( 'NONE',  ( 3.279658019245000222, 1511.011611623900080, 216.6862599316969806 ) ) ;
#104460=CARTESIAN_POINT ( 'NONE',  ( 1.121950743945000051, 1517.123342927159911, 204.1084165760470057 ) ) ;
#104465=CARTESIAN_POINT ( 'NONE',  ( -0.7526715882979990724, 1516.710624944440042, 201.4081970979170251 ) ) ;
#104467=CARTESIAN_POINT ( 'NONE',  ( -11.92849872888365681, 1511.839858410421130, 194.1166199672483970 ) ) ;
#104473=DIRECTION ( 'NONE',  ( -1.000000000000000000, 0.000000000000000000, 0.000000000000000000 ) ) ;
#104475=CARTESIAN_POINT ( 'NONE',  ( -6.934528567894999718, 1516.588006113850042, 211.9958048218269937 ) ) ;
#104483=CARTESIAN_POINT ( 'NONE',  ( -4.612671377915000370, 1516.783665406140017, 209.8782801844560026 ) ) ;
#104497=CARTESIAN_POINT ( 'NONE',  ( 4.987078416414999715, 1508.551704408389924, 212.6094384009469707 ) ) ;
#104499=CARTESIAN_POINT ( 'NONE',  ( -2.483322492024999661, 1517.139039350860003, 215.6851008610869940 ) ) ;
#104511=CARTESIAN_POINT ( 'NONE',  ( 7.683752556684630086, 1511.083508941950186, 203.3594437696220041 ) ) ;
#104523=CARTESIAN_POINT ( 'NONE',  ( -9.220992939474999872, 1511.932705841380084, 197.3648029957670076 ) ) ;
#104525=CARTESIAN_POINT ( 'NONE',  ( 8.613178118295000019, 1512.860712383139798, 206.8726288444870249 ) ) ;
#104585=CARTESIAN_POINT ( 'NONE',  ( -2.865636847234999784, 1516.815173273089840, 210.2578502442970318 ) ) ;
#104602=CARTESIAN_POINT ( 'NONE',  ( 5.775625077365000415, 1516.745833913490060, 208.3665194962490261 ) ) ;
#104607=ORIENTED_EDGE ( 'NONE', *, *, #92850, .T. ) ;
#104617=CARTESIAN_POINT ( 'NONE',  ( -6.563254928984999736, 1517.139039350860003, 206.6385234782069915 ) ) ;
#104626=FACE_OUTER_BOUND ( 'NONE', #100418, .T. ) ;
#104634=CARTESIAN_POINT ( 'NONE',  ( 0.01289778877310149806, 1516.939723362869927, 214.1281058189269970 ) ) ;
#104641=DIRECTION ( 'NONE',  ( -0.5224574779878928821, 0.7067418228236548305, 0.4770263929453257834 ) ) ;
#104653=DIRECTION ( 'NONE',  ( -1.000000000000000000, 0.000000000000000000, 0.000000000000000000 ) ) ;
#104679=CARTESIAN_POINT ( 'NONE',  ( 8.311290096204249522, 1511.035127054690065, 202.3471219999200059 ) ) ;
#104704=CARTESIAN_POINT ( 'NONE',  ( -2.494020320564999782, 1516.876240617270014, 206.8389307488369866 ) ) ;
#104718=CARTESIAN_POINT ( 'NONE',  ( -2.864972154145000172, 1516.859514182039902, 212.0024388992169975 ) ) ;
#104723=EDGE_CURVE ( 'NONE', #8750, #85013, #107387, .T. ) ;
#104733=ORIENTED_EDGE ( 'NONE', *, *, #27359, .F. ) ;
#104742=CARTESIAN_POINT ( 'NONE',  ( 6.961841748697260357, 1508.551566289579796, 202.5699741863490146 ) ) ;
#104749=CARTESIAN_POINT ( 'NONE',  ( -5.005700239535000762, 1516.732530461250008, 202.1838802717869896 ) ) ;
#104750=CARTESIAN_POINT ( 'NONE',  ( -6.938478822895000064, 1516.719999691880048, 209.8757167055200057 ) ) ;
#104773=CARTESIAN_POINT ( 'NONE',  ( -6.946514214915000096, 1512.024017243120170, 202.0369668883770089 ) ) ;
#104774=VERTEX_POINT ( 'NONE', #27802 ) ;
#104788=CARTESIAN_POINT ( 'NONE',  ( 14.92730988393499914, 1514.452905717119847, 225.3342559640670117 ) ) ;
#104796=CARTESIAN_POINT ( 'NONE',  ( -6.950833568235000648, 1517.156142772249950, 206.6378959915070084 ) ) ;
#104850=CARTESIAN_POINT ( 'NONE',  ( 6.548821941055000373, 1516.688761843659904, 205.0844676760469838 ) ) ;
#104871=CARTESIAN_POINT ( 'NONE',  ( 4.624099291334999862, 1516.962555622980062, 212.3771868965270073 ) ) ;
#104881=EDGE_CURVE ( 'NONE', #38027, #81968, #41908, .T. ) ;
#104882=CARTESIAN_POINT ( 'NONE',  ( -7.881533630355000319, 1511.927085655870087, 215.3995285225870191 ) ) ;
#104883=CARTESIAN_POINT ( 'NONE',  ( 16.78028216998529132, 1513.363094769292047, 196.2862811899955204 ) ) ;
#104894=CARTESIAN_POINT ( 'NONE',  ( -2.299983615734999987, 1516.861367446839949, 206.8392230197369770 ) ) ;
#104912=CARTESIAN_POINT ( 'NONE',  ( 0.7543881828220019292, 1516.727502608469877, 215.6727161143369926 ) ) ;
#104916=AXIS2_PLACEMENT_3D ( 'NONE', #34336, #35440, #68514 ) ;
#104920=CARTESIAN_POINT ( 'NONE',  ( 7.337153768115000751, 1517.119374999550018, 212.3815752680669959 ) ) ;
#104936=CARTESIAN_POINT ( 'NONE',  ( 2.868433798504999910, 1517.020727862619879, 204.1095288638669842 ) ) ;
#104977=CARTESIAN_POINT ( 'NONE',  ( 2.872836622524999939, 1517.158319634930194, 201.3964737998670103 ) ) ;
#104982=CARTESIAN_POINT ( 'NONE',  ( 7.618904756804999678, 1511.873873588870083, 206.4967791623069786 ) ) ;
#105003=EDGE_CURVE ( 'NONE', #110691, #52986, #74058, .T. ) ;
#105005=ORIENTED_EDGE ( 'NONE', *, *, #1154, .T. ) ;
#105014=CARTESIAN_POINT ( 'NONE',  ( -6.550389470255000290, 1516.755758396839838, 214.1281755516169767 ) ) ;
#105015=CARTESIAN_POINT ( 'NONE',  ( 2.701540375215000012, 1511.422242621320265, 216.6970128893269987 ) ) ;
#105021=CARTESIAN_POINT ( 'NONE',  ( 4.999456390405000228, 1516.830644417779922, 204.5005780481670001 ) ) ;
#105024=CARTESIAN_POINT ( 'NONE',  ( -2.291047527245000381, 1516.524310051880093, 201.4130759250869858 ) ) ;
#105037=CARTESIAN_POINT ( 'NONE',  ( -7.709681306425000713, 1516.559109716219837, 211.9945464874270158 ) ) ;
#105043=CARTESIAN_POINT ( 'NONE',  ( -1.906501101195560124E-08, 1517.020990152690047, 209.1218459511669892 ) ) ;
#105052=DIRECTION ( 'NONE',  ( 0.4025563316115431389, 0.03449475076686812219, 0.9147450530333514074 ) ) ;
#105056=CARTESIAN_POINT ( 'NONE',  ( -3.452289220704999551, 1517.069378699710114, 215.6835323934670328 ) ) ;
#105067=CARTESIAN_POINT ( 'NONE',  ( 7.596320571148669210, 1510.929912129050081, 203.3182735752830013 ) ) ;
#105079=ORIENTED_EDGE ( 'NONE', *, *, #44206, .F. ) ;
#105089=CARTESIAN_POINT ( 'NONE',  ( -7.559010200133819524, 1510.805212306365547, 214.6182763928821657 ) ) ;
#105121=B_SPLINE_CURVE_WITH_KNOTS ( 'NONE', 5,
 ( #95970, #44477, #110558, #34405, #68578, #87011, #59618, #25978, #9750, #78623, #60177, #52883 ),
 .UNSPECIFIED., .F., .F.,
 ( 6, 3, 3, 6 ),
 ( -8.912489289850000773, -7.801458206509999549, -6.062162762939999894, -3.672001930560000460 ),
 .UNSPECIFIED. ) ;
#105141=CARTESIAN_POINT ( 'NONE',  ( 2.881325373965000214, 1517.003078582959688, 210.2407492406470055 ) ) ;
#105151=CARTESIAN_POINT ( 'NONE',  ( 1.126138108584999964, 1517.208444099459939, 201.3951612445669923 ) ) ;
#105157=CARTESIAN_POINT ( 'NONE',  ( 7.326072144144999854, 1516.714320817460020, 208.3685457967989976 ) ) ;
#105175=CARTESIAN_POINT ( 'NONE',  ( 4.026777485955000735, 1516.718889242609976, 206.8247602162870180 ) ) ;
#105194=CARTESIAN_POINT ( 'NONE',  ( -5.775236830874999505, 1516.804776704140068, 214.1294346171470124 ) ) ;
#105248=CARTESIAN_POINT ( 'NONE',  ( -1.906563618092599921E-08, 1509.051704408389924, 214.1089243866270238 ) ) ;
#105260=CARTESIAN_POINT ( 'NONE',  ( 4.027051405805000428, 1516.733363207009916, 206.6306575737070261 ) ) ;
#105265=VECTOR ( 'NONE', #67121, 1000.000000000000114 ) ;
#105283=CARTESIAN_POINT ( 'NONE',  ( 14.69200427761992600, 1514.485057820107158, 225.4415873000313297 ) ) ;
#105286=ORIENTED_EDGE ( 'NONE', *, *, #97880, .T. ) ;
#105295=CARTESIAN_POINT ( 'NONE',  ( 7.012524228414029892, 1508.551704613440052, 203.1374999936529946 ) ) ;
#105302=CARTESIAN_POINT ( 'NONE',  ( -6.945490086935000029, 1516.932669162149978, 203.3434733684869968 ) ) ;
#105323=CARTESIAN_POINT ( 'NONE',  ( -7.943523479595000047, 1514.557408760799945, 202.6827084971669990 ) ) ;
#105342=CARTESIAN_POINT ( 'NONE',  ( 12.84824842633499919, 1512.167884426309911, 224.5031668304669950 ) ) ;
#105350=CARTESIAN_POINT ( 'NONE',  ( -7.726331963605000297, 1517.194972660189933, 206.8303316343270239 ) ) ;
#105371=CARTESIAN_POINT ( 'NONE',  ( 5.768664107876966263, 1510.557600717794685, 216.6626378734150933 ) ) ;
#105405=CARTESIAN_POINT ( 'NONE',  ( -0.7564342523539989704, 1516.783665406140017, 204.5091745923169810 ) ) ;
#105427=CARTESIAN_POINT ( 'NONE',  ( 4.623787969365000805, 1516.947419719950176, 212.5709951659769956 ) ) ;
#105438=CARTESIAN_POINT ( 'NONE',  ( -7.211759849075000339, 1511.702066573629963, 215.8939835620469978 ) ) ;
#105439=CARTESIAN_POINT ( 'NONE',  ( 16.25466701628457500, 1514.562529182973549, 194.3320297101351741 ) ) ;
#105447=CARTESIAN_POINT ( 'NONE',  ( -3.424720339024999838, 1517.051704408389924, 217.6596685689069943 ) ) ;
#105449=CARTESIAN_POINT ( 'NONE',  ( 3.251611325815000342, 1516.779243033999819, 206.8234764622770001 ) ) ;
#105461=DIRECTION ( 'NONE',  ( 0.4999999999998399614, -0.7071067811867740582, 0.4999999999998399614 ) ) ;
#105469=CARTESIAN_POINT ( 'NONE',  ( -0.7386049428049979992, 1517.122674412569950, 215.6839400395269877 ) ) ;
#105471=CARTESIAN_POINT ( 'NONE',  ( 5.704331096967670156, 1511.494703458840149, 217.3688750472999800 ) ) ;
#105473=CARTESIAN_POINT ( 'NONE',  ( 2.879956924955000108, 1516.827328999679821, 212.3743765858270081 ) ) ;
#105483=CARTESIAN_POINT ( 'NONE',  ( 2.344512035239230130, 1516.526058368810027, 216.8306617777329848 ) ) ;
#105490=CARTESIAN_POINT ( 'NONE',  ( -1.133517003235000153, 1516.713079096360161, 204.5117660986770147 ) ) ;
#105498=EDGE_CURVE ( 'NONE', #52986, #36271, #65921, .T. ) ;
#105503=EDGE_CURVE ( 'NONE', #37961, #31839, #16893, .T. ) ;
#105534=CARTESIAN_POINT ( 'NONE',  ( -12.13495040386500001, 1511.961073825299991, 193.0130861717670143 ) ) ;
#105539=CARTESIAN_POINT ( 'NONE',  ( 7.329930013194999816, 1516.881930554049859, 201.4037113026670056 ) ) ;
#105543=CARTESIAN_POINT ( 'NONE',  ( 7.893411082094998754, 1512.020737142380085, 206.1250608998970222 ) ) ;
#105554=CARTESIAN_POINT ( 'NONE',  ( -7.685457311955000925, 1511.037966505499980, 214.2610714211569984 ) ) ;
#105574=CARTESIAN_POINT ( 'NONE',  ( -3.257220640824999958, 1517.040132827679827, 214.9086836491569841 ) ) ;
#105575=CARTESIAN_POINT ( 'NONE',  ( 2.564633783425000146, 1511.308638870219966, 216.6940388207569868 ) ) ;
#105583=CARTESIAN_POINT ( 'NONE',  ( -2.877744984375000037, 1516.723920667490120, 204.5127816287269980 ) ) ;
#105599=CARTESIAN_POINT ( 'NONE',  ( 6.949265646015000186, 1517.089216728169959, 212.5747629931370000 ) ) ;
#105604=CARTESIAN_POINT ( 'NONE',  ( -1.127928371535000140, 1516.989863902050047, 209.1319708558790182 ) ) ;
#105615=CARTESIAN_POINT ( 'NONE',  ( 7.548872300095000654, 1510.418062979259958, 203.9404357814470075 ) ) ;
#105619=CARTESIAN_POINT ( 'NONE',  ( -1.123101616545000070, 1517.157901477309906, 214.9105372957470195 ) ) ;
#105624=CARTESIAN_POINT ( 'NONE',  ( -0.7526715882979990724, 1516.710624944440042, 201.4081970979170251 ) ) ;
#105630=CARTESIAN_POINT ( 'NONE',  ( 8.423122042745829319, 1511.533951550999973, 203.4036934630460109 ) ) ;
#105644=CARTESIAN_POINT ( 'NONE',  ( 7.821732060355000016, 1516.863303996349941, 216.8564630578470087 ) ) ;
#105685=AXIS2_PLACEMENT_3D ( 'NONE', #2589, #20990, #96065 ) ;
#105694=CARTESIAN_POINT ( 'NONE',  ( -9.638115897704999213, 1517.051704408389924, 203.7504991310570119 ) ) ;
#105707=CARTESIAN_POINT ( 'NONE',  ( -2.476170635034999901, 1516.819260244609950, 210.8389306816469855 ) ) ;
#105716=CARTESIAN_POINT ( 'NONE',  ( 1.709384572955000126, 1517.224900789629828, 201.7820965968870155 ) ) ;
#105722=CARTESIAN_POINT ( 'NONE',  ( 0.7533003524100010395, 1516.992029636990083, 209.8620668306199946 ) ) ;
#105738=CARTESIAN_POINT ( 'NONE',  ( 0.7353365397730019515, 1516.995911393979895, 206.2425275143270085 ) ) ;
#105744=ADVANCED_FACE ( 'NONE', ( #11574 ), #70406, .F. ) ;
#105755=CARTESIAN_POINT ( 'NONE',  ( -3.258474617075000079, 1517.083030555940013, 215.6838419306269827 ) ) ;
#105771=CARTESIAN_POINT ( 'NONE',  ( 5.371346801045000063, 1520.551704408390151, 199.4837300725270097 ) ) ;
#105773=ORIENTED_EDGE ( 'NONE', *, *, #22093, .T. ) ;
#105774=EDGE_CURVE ( 'NONE', #39998, #89473, #30279, .T. ) ;
#105776=CARTESIAN_POINT ( 'NONE',  ( -6.391938905018056616, 1508.551704408390151, 202.1089245808659882 ) ) ;
#105780=CARTESIAN_POINT ( 'NONE',  ( -6.742045582256606551, 1509.032357776622348, 202.0097237844711344 ) ) ;
#105802=CARTESIAN_POINT ( 'NONE',  ( 7.708815788408339920, 1516.526058372639909, 206.7773338513199803 ) ) ;
#105827=CARTESIAN_POINT ( 'NONE',  ( 6.933616821004999764, 1516.548716157039962, 206.8295387017270173 ) ) ;
#105846=CARTESIAN_POINT ( 'NONE',  ( 13.06910704241984966, 1513.473960729436385, 225.9112088208277953 ) ) ;
#105864=CARTESIAN_POINT ( 'NONE',  ( -1.131796848745000084, 1516.659138130710289, 203.3488676535569937 ) ) ;
#105884=CARTESIAN_POINT ( 'NONE',  ( -7.266995445965000577, 1512.686126173209914, 202.3407130533369980 ) ) ;
#105902=CARTESIAN_POINT ( 'NONE',  ( 15.01814799273499901, 1514.214451716350140, 223.8476172842669882 ) ) ;
#105910=CARTESIAN_POINT ( 'NONE',  ( -1.136814071995000175, 1516.854133554269993, 206.8377924607469822 ) ) ;
#105923=FACE_OUTER_BOUND ( 'NONE', #92148, .T. ) ;
#105931=CARTESIAN_POINT ( 'NONE',  ( 6.372167600494999640, 1511.069621805459974, 216.5183910133270047 ) ) ;
#105947=CARTESIAN_POINT ( 'NONE',  ( -8.568313719024999386, 1512.631076693560090, 197.0179983452670172 ) ) ;
#105951=EDGE_CURVE ( 'NONE', #17368, #68158, #55532, .T. ) ;
#105966=CARTESIAN_POINT ( 'NONE',  ( -7.722536802824999214, 1517.050041317280147, 204.5049460973469877 ) ) ;
#105987=CARTESIAN_POINT ( 'NONE',  ( 4.042729802795000715, 1516.919782530640077, 212.3762473738369749 ) ) ;
#105996=CARTESIAN_POINT ( 'NONE',  ( -6.563811449735000636, 1514.071098020780028, 216.7756948377870003 ) ) ;
#105997=CARTESIAN_POINT ( 'NONE',  ( 16.51878312702331186, 1514.214507863231120, 194.7969773782033656 ) ) ;
#106007=CARTESIAN_POINT ( 'NONE',  ( -7.726331963605000297, 1517.194972660189933, 206.8303316343270239 ) ) ;
#106024=CARTESIAN_POINT ( 'NONE',  ( 1.709358663124999955, 1516.542957540330008, 216.0554336257470140 ) ) ;
#106025=CARTESIAN_POINT ( 'NONE',  ( -3.330134203884999700, 1515.051704408389924, 213.4516374609670208 ) ) ;
#106026=CARTESIAN_POINT ( 'NONE',  ( 5.912727970548059986, 1510.598356033829987, 216.6556934984580209 ) ) ;
#106028=CARTESIAN_POINT ( 'NONE',  ( 5.787476994515000861, 1517.070197312179971, 211.9915394291670054 ) ) ;
#106033=CARTESIAN_POINT ( 'NONE',  ( 8.598884471655001249, 1512.314860040240092, 206.8869224911269953 ) ) ;
#106044=CARTESIAN_POINT ( 'NONE',  ( 4.998515157294999511, 1516.787536375099990, 205.0819486540370065 ) ) ;
#106075=CARTESIAN_POINT ( 'NONE',  ( -12.18811182046500008, 1511.857118786289902, 193.8586218496669744 ) ) ;
#106080=CARTESIAN_POINT ( 'NONE',  ( -0.7526715882979990724, 1516.710624944440042, 201.4081970979170251 ) ) ;
#106084=CARTESIAN_POINT ( 'NONE',  ( 7.774021405044999611, 1512.205735116489905, 206.2993818420169987 ) ) ;
#106089=EDGE_LOOP ( 'NONE', ( #101243, #37368, #41937, #87969 ) ) ;
#106094=CARTESIAN_POINT ( 'NONE',  ( -8.100204470725000050, 1511.336728379370243, 213.6607147150270123 ) ) ;
#106100=( LENGTH_UNIT ( ) NAMED_UNIT ( * ) SI_UNIT ( .MILLI., .METRE. ) );
#106109=ORIENTED_EDGE ( 'NONE', *, *, #38482, .T. ) ;
#106113=CARTESIAN_POINT ( 'NONE',  ( -2.288357445734999995, 1517.116049120239950, 214.9102823043970147 ) ) ;
#106114=CARTESIAN_POINT ( 'NONE',  ( 4.826478482935000258, 1511.220390575160081, 217.0108025382170069 ) ) ;
#106123=CARTESIAN_POINT ( 'NONE',  ( -4.622842882315000068, 1516.901952101700090, 205.0913314195169903 ) ) ;
#106136=CARTESIAN_POINT ( 'NONE',  ( 2.878693249144999466, 1516.766397346390022, 213.1495431961470217 ) ) ;
#106142=CARTESIAN_POINT ( 'NONE',  ( -1.122033430074999893, 1516.972341476009888, 209.8777854684929878 ) ) ;
#106158=CARTESIAN_POINT ( 'NONE',  ( 1.709358663124999955, 1516.542957540330008, 216.0554336257470140 ) ) ;
#106163=CARTESIAN_POINT ( 'NONE',  ( 1.709384572955000126, 1517.224900789629828, 201.7820965968870155 ) ) ;
#106181=CARTESIAN_POINT ( 'NONE',  ( 14.49568591477500057, 1514.921196705999819, 224.3246435558060057 ) ) ;
#106240=CARTESIAN_POINT ( 'NONE',  ( 5.013274961385000061, 1517.068517094990057, 211.4089302402969963 ) ) ;
#106248=EDGE_CURVE ( 'NONE', #47608, #103079, #75232, .T. ) ;
#106250=CARTESIAN_POINT ( 'NONE',  ( -3.260378293205000055, 1516.582197289609894, 201.4115600944169842 ) ) ;
#106261=EDGE_CURVE ( 'NONE', #52986, #42748, #106334, .T. ) ;
#106271=CARTESIAN_POINT ( 'NONE',  ( 1.701027822874999984, 1516.937508036699910, 206.6270879340970055 ) ) ;
#106275=ORIENTED_EDGE ( 'NONE', *, *, #42966, .F. ) ;
#106282=CARTESIAN_POINT ( 'NONE',  ( 7.150360480941603036, 1512.239113741272149, 216.2200089361317339 ) ) ;
#106287=CARTESIAN_POINT ( 'NONE',  ( -6.937965698444999774, 1516.732530461250008, 214.1275461716370216 ) ) ;
#106289=ORIENTED_EDGE ( 'NONE', *, *, #28798, .T. ) ;
#106290=CARTESIAN_POINT ( 'NONE',  ( 7.714278200979600264, 1516.734659492849914, 208.4225296901069839 ) ) ;
#106334=LINE ( 'NONE', #29620, #89444 ) ;
#106360=CARTESIAN_POINT ( 'NONE',  ( -4.045182518055000287, 1517.057265928030120, 207.4180663268770104 ) ) ;
#106367=DIRECTION ( 'NONE',  ( -0.7384854939282345931, 0.000000000000000000, 0.6742693640212131800 ) ) ;
#106385=ORIENTED_EDGE ( 'NONE', *, *, #32444, .F. ) ;
#106402=CARTESIAN_POINT ( 'NONE',  ( -3.457266643525000127, 1516.691414181030041, 203.3491180233569935 ) ) ;
#106417=CARTESIAN_POINT ( 'NONE',  ( -2.249664798384999997, 1512.877808311729950, 200.5082201411669871 ) ) ;
#106423=CARTESIAN_POINT ( 'NONE',  ( -6.844666251345000063, 1512.637906871299947, 201.1997175912570128 ) ) ;
#106435=DIRECTION ( 'NONE',  ( -0.4999999999998399614, -0.7071067811867740582, 0.4999999999998399614 ) ) ;
#106438=CARTESIAN_POINT ( 'NONE',  ( 15.00364256283500097, 1514.335759350750095, 225.2363441599670182 ) ) ;
#106446=CARTESIAN_POINT ( 'NONE',  ( 1.700706776364999895, 1516.923170579120097, 206.8211163054370161 ) ) ;
#106485=DIRECTION ( 'NONE',  ( 0.9980844203940678616, -0.06184550950381709211, 0.001619481661242269796 ) ) ;
#106500=CARTESIAN_POINT ( 'NONE',  ( -0.01327408612949850138, 1516.939877939420057, 205.6663500982469941 ) ) ;
#106514=CARTESIAN_POINT ( 'NONE',  ( -7.710967015764999211, 1516.608208975040043, 210.2506035313070072 ) ) ;
#106531=CARTESIAN_POINT ( 'NONE',  ( 16.78772369872005754, 1513.520094853501405, 195.9605301170960843 ) ) ;
#106542=CARTESIAN_POINT ( 'NONE',  ( 6.933616821004999764, 1516.548716157039962, 206.8295387017270173 ) ) ;
#106556=CARTESIAN_POINT ( 'NONE',  ( -6.164039445902147030, 1510.821818207758270, 201.6558465868637313 ) ) ;
#106557=DIRECTION ( 'NONE',  ( -1.387778780781598557E-14, -1.000000000000000000, 0.000000000000000000 ) ) ;
#106560=EDGE_CURVE ( 'NONE', #44996, #78702, #100819, .T. ) ;
#106561=CARTESIAN_POINT ( 'NONE',  ( 7.331183090945000203, 1516.882217593000178, 216.0635732225570109 ) ) ;
#106564=CARTESIAN_POINT ( 'NONE',  ( 3.461047291624999911, 1516.858765657450249, 212.5691103191969944 ) ) ;
#106582=CARTESIAN_POINT ( 'NONE',  ( 6.548821941055000373, 1516.688761843659904, 205.0844676760469838 ) ) ;
#106615=CARTESIAN_POINT ( 'NONE',  ( -13.99234591236500158, 1513.736060322949925, 192.3918525003670084 ) ) ;
#106616=DIRECTION ( 'NONE',  ( -0.7071067811865474617, 4.329780281177460882E-17, 0.7071067811865474617 ) ) ;
#106618=CARTESIAN_POINT ( 'NONE',  ( -3.261007169695000041, 1516.596789218710001, 201.7991362452670216 ) ) ;
#106622=CARTESIAN_POINT ( 'NONE',  ( 7.404094472206104172, 1512.905891558378698, 217.4471223568880021 ) ) ;
#106630=CARTESIAN_POINT ( 'NONE',  ( -7.329925260613682880, 1516.833976298084281, 201.4049670776166749 ) ) ;
#106633=CARTESIAN_POINT ( 'NONE',  ( -7.937216491484998748, 1511.802450769970164, 212.2876873266469886 ) ) ;
#106652=CARTESIAN_POINT ( 'NONE',  ( 5.006329581384999727, 1516.755758396839838, 215.6722354023569892 ) ) ;
#106661=CARTESIAN_POINT ( 'NONE',  ( 5.773668814845000163, 1516.734985836460055, 205.0832084693769843 ) ) ;
#106675=CARTESIAN_POINT ( 'NONE',  ( -1.702406023195000007, 1516.999105586269934, 212.3918307515370145 ) ) ;
#106680=CARTESIAN_POINT ( 'NONE',  ( -7.718845898157540297, 1516.909122020879977, 209.2104016507690005 ) ) ;
#106681=CARTESIAN_POINT ( 'NONE',  ( 6.951517132375000685, 1517.194816588360027, 210.2467400204669730 ) ) ;
#106685=ORIENTED_EDGE ( 'NONE', *, *, #68675, .T. ) ;
#106693=CARTESIAN_POINT ( 'NONE',  ( -1.708747662384999977, 1517.213554313520035, 216.0740123525270064 ) ) ;
#106698=CARTESIAN_POINT ( 'NONE',  ( 7.716252052974999387, 1516.810037859429940, 202.1795012402670011 ) ) ;
#106699=CARTESIAN_POINT ( 'NONE',  ( -16.20130421256499886, 1512.842772631639946, 220.3734026763669931 ) ) ;
#106717=DIRECTION ( 'NONE',  ( 0.06162841671618448508, -0.9961946980917499861, -0.06162841671618445039 ) ) ;
#106737=CARTESIAN_POINT ( 'NONE',  ( 14.86941678424950020, 1514.013728164709846, 223.9821045949209974 ) ) ;
#106739=VERTEX_POINT ( 'NONE', #48673 ) ;
#106750=AXIS2_PLACEMENT_3D ( 'NONE', #109735, #34678, #50945 ) ;
#106778=CARTESIAN_POINT ( 'NONE',  ( -3.251611363945000388, 1516.779243033999819, 211.4202154400570066 ) ) ;
#106780=CARTESIAN_POINT ( 'NONE',  ( -5.771149113014999443, 1516.616791731099966, 211.6102065995370083 ) ) ;
#106787=CARTESIAN_POINT ( 'NONE',  ( -4.617490504904999682, 1516.685667699390024, 201.7969310139470167 ) ) ;
#106802=CARTESIAN_POINT ( 'NONE',  ( -3.255809902135000211, 1516.837969789639828, 209.8792719553279937 ) ) ;
#106807=CARTESIAN_POINT ( 'NONE',  ( 7.985842358304999777, 1511.355055856599847, 205.0854651845669991 ) ) ;
#106808=CARTESIAN_POINT ( 'NONE',  ( 3.445685077385000294, 1516.778761582560037, 206.6297153089269898 ) ) ;
#106811=CARTESIAN_POINT ( 'NONE',  ( -2.446740418831741870, 1516.554415856173591, 202.0292846036045944 ) ) ;
#106826=CARTESIAN_POINT ( 'NONE',  ( -6.550389470255000290, 1516.755758396839838, 214.1281755516169767 ) ) ;
#106828=CARTESIAN_POINT ( 'NONE',  ( 7.710405941315919165, 1516.586783862359880, 207.7425835133209944 ) ) ;
#106855=CARTESIAN_POINT ( 'NONE',  ( -6.252266492314999979, 1511.741868877540128, 200.3335294429169835 ) ) ;
#106858=CARTESIAN_POINT ( 'NONE',  ( -4.832616828004995924, 1508.551704408610021, 212.6094309338623418 ) ) ;
#106868=EDGE_CURVE ( 'NONE', #11573, #37685, #40798, .T. ) ;
#106871=CARTESIAN_POINT ( 'NONE',  ( 3.487592431261229642, 1509.038615938009798, 213.6090957240379851 ) ) ;
#106879=DIRECTION ( 'NONE',  ( -1.577721810442025012E-32, -1.000000000000000000, 6.123233995736769734E-17 ) ) ;
#106895=CARTESIAN_POINT ( 'NONE',  ( -7.670153693721269761, 1511.304111283970087, 215.1254345037010012 ) ) ;
#106900=CARTESIAN_POINT ( 'NONE',  ( -1.137296688934999800, 1516.908147884120126, 207.4199954749970232 ) ) ;
#106929=CARTESIAN_POINT ( 'NONE',  ( 3.487585214244389942, 1508.551704408389924, 204.2892321559630204 ) ) ;
#106943=CARTESIAN_POINT ( 'NONE',  ( -7.333070173014999860, 1516.955859323880077, 203.3428461583270064 ) ) ;
#106966=CARTESIAN_POINT ( 'NONE',  ( -7.809063951335000198, 1513.978875661330221, 201.9427188508670099 ) ) ;
#106980=CARTESIAN_POINT ( 'NONE',  ( 14.58906255643499961, 1513.961173499609913, 225.5460952577670071 ) ) ;
#106981=CARTESIAN_POINT ( 'NONE',  ( -17.15254157612201880, 1516.660421270687038, 223.0819975641380495 ) ) ;
#106987=CARTESIAN_POINT ( 'NONE',  ( 2.476450664134999702, 1516.843453247299749, 206.8221896160070230 ) ) ;
#107019=B_SPLINE_SURFACE_WITH_KNOTS ( 'NONE', 5, 5, ( 
 ( #13089, #4175, #55696, #5264, #89817, #107724, #79789, #81957, #47274 ),
 ( #22028, #89269, #106075, #37774, #29901, #56225, #29355, #37222, #12565 ),
 ( #3094, #71419, #81397, #31009, #105534, #64093, #20943, #65189, #4709 ),
 ( #73031, #21483, #63556, #38852, #63020, #13634, #47822, #107169, #80877 ),
 ( #46195, #97671, #97126, #71965, #28823, #38305, #30461, #64646, #98215 ),
 ( #98766, #20395, #54599, #11474, #72486, #88732, #12015, #106615, #73595 ),
 ( #39417, #90356, #55148, #19851, #54055, #80329, #45649, #3645, #88182 ),
 ( #75781, #14757, #101500, #109394, #32670, #41066, #24787, #66305, #39966 ),
 ( #100958, #57890, #15832, #83612, #50036, #90917, #84712, #65736, #6910 ) ),
 .UNSPECIFIED., .F., .F., .F.,
 ( 6, 3, 6 ),
 ( 6, 3, 6 ),
 ( 9.902195898180000455, 12.38020728900000123, 16.40090783169999966 ),
 ( 0.000000000000000000, 0.5000000000000000000, 1.000000000000000000 ),
 .UNSPECIFIED. ) ;
#107039=CARTESIAN_POINT ( 'NONE',  ( -3.836805930384536545, 1511.512554418210811, 200.9783825810452527 ) ) ;
#107047=CARTESIAN_POINT ( 'NONE',  ( -1.135185082175000026, 1516.778853242349896, 205.6747174714770097 ) ) ;
#107049=VERTEX_POINT ( 'NONE', #96601 ) ;
#107058=ORIENTED_EDGE ( 'NONE', *, *, #93291, .F. ) ;
#107063=CARTESIAN_POINT ( 'NONE',  ( -7.326072182274999456, 1516.714320817460020, 209.8751461055349807 ) ) ;
#107082=CARTESIAN_POINT ( 'NONE',  ( 10.96015508933500016, 1516.551704408390151, 225.0317485278669949 ) ) ;
#107088=CARTESIAN_POINT ( 'NONE',  ( -1.717139122245000094, 1516.949031626070109, 208.0040058453670042 ) ) ;
#107100=CARTESIAN_POINT ( 'NONE',  ( -5.523053292569629846, 1510.639750819970004, 201.5677449951700169 ) ) ;
#107106=CARTESIAN_POINT ( 'NONE',  ( -2.871580426725000024, 1517.129577905929864, 216.0720609035170128 ) ) ;
#107109=CARTESIAN_POINT ( 'NONE',  ( -10.96015512746500065, 1516.551704408390151, 193.2119433744669834 ) ) ;
#107112=CARTESIAN_POINT ( 'NONE',  ( -3.447264387095000160, 1516.858765657450249, 212.5828932618570093 ) ) ;
#107130=CARTESIAN_POINT ( 'NONE',  ( 1.121383591734999907, 1517.104192383289956, 204.4960559556369901 ) ) ;
#107137=CARTESIAN_POINT ( 'NONE',  ( 4.151444298953053114, 1516.720891557477444, 200.3679918764218826 ) ) ;
#107159=CARTESIAN_POINT ( 'NONE',  ( 7.321844823074391329, 1508.611350403034521, 203.6084103738731130 ) ) ;
#107169=CARTESIAN_POINT ( 'NONE',  ( -12.04783380916500057, 1512.799725290120023, 192.4725698663669959 ) ) ;
#107173=CARTESIAN_POINT ( 'NONE',  ( 0.7391219670640019057, 1517.130100026000036, 202.1721425974470208 ) ) ;
#107188=CARTESIAN_POINT ( 'NONE',  ( -7.717505791104999346, 1516.857914730730045, 201.4043401791270185 ) ) ;
#107198=B_SPLINE_CURVE_WITH_KNOTS ( 'NONE', 5,
 ( #40422, #66214, #64558, #6813, #49391, #5171 ),
 .UNSPECIFIED., .F., .F.,
 ( 6, 6 ),
 ( 0.000000000000000000, 1.000000000000000000 ),
 .UNSPECIFIED. ) ;
#107212=CARTESIAN_POINT ( 'NONE',  ( -3.452917061035000401, 1517.089216728169959, 216.0711116162470091 ) ) ;
#107219=CARTESIAN_POINT ( 'NONE',  ( -4.621897862544999569, 1516.858533673840157, 204.5099662467769974 ) ) ;
#107224=CARTESIAN_POINT ( 'NONE',  ( 6.044020038074999768, 1511.752511073100095, 217.4188488492769977 ) ) ;
#107232=CARTESIAN_POINT ( 'NONE',  ( 5.010422963235000360, 1516.929569650079884, 213.1529883219070030 ) ) ;
#107237=CARTESIAN_POINT ( 'NONE',  ( -7.709610715716689988, 1516.556413965810179, 210.7279121869730147 ) ) ;
#107238=CARTESIAN_POINT ( 'NONE',  ( 0.01265818781360149997, 1516.959716008189844, 210.8316124642570060 ) ) ;
#107252=CARTESIAN_POINT ( 'NONE',  ( -2.871580426725000024, 1517.129577905929864, 216.0720609035170128 ) ) ;
#107256=CARTESIAN_POINT ( 'NONE',  ( -7.717505791104999346, 1516.857914730730045, 201.4043401791270185 ) ) ;
#107258=ORIENTED_EDGE ( 'NONE', *, *, #40920, .F. ) ;
#107277=DIRECTION ( 'NONE',  ( 0.4999997527789440399, 0.7071067730516870098, -0.5000002587253580266 ) ) ;
#107286=CARTESIAN_POINT ( 'NONE',  ( -7.500000019064997581, 1516.976251993718961, 208.9751496355367806 ) ) ;
#107288=DIRECTION ( 'NONE',  ( -1.000000000000000000, 0.000000000000000000, 0.000000000000000000 ) ) ;
#107297=CARTESIAN_POINT ( 'NONE',  ( 12.18971934853500194, 1512.123542805230272, 223.8476153537669973 ) ) ;
#107299=ORIENTED_EDGE ( 'NONE', *, *, #34365, .F. ) ;
#107338=CARTESIAN_POINT ( 'NONE',  ( -6.546001388695000145, 1516.557392317769882, 210.8318505190270002 ) ) ;
#107340=CARTESIAN_POINT ( 'NONE',  ( 1.135460316954999938, 1516.790374942449944, 212.3751473514870156 ) ) ;
#107347=CARTESIAN_POINT ( 'NONE',  ( -2.291676311554999845, 1516.534976163889951, 201.8006522243570089 ) ) ;
#107362=CARTESIAN_POINT ( 'NONE',  ( 6.563915523884999992, 1517.184063036290127, 210.2461356256870033 ) ) ;
#107367=FACE_OUTER_BOUND ( 'NONE', #99609, .T. ) ;
#107368=CARTESIAN_POINT ( 'NONE',  ( -5.014195139944999546, 1517.120861839400050, 207.4163795216369977 ) ) ;
#107383=CARTESIAN_POINT ( 'NONE',  ( -7.325541825264999751, 1516.710692850270107, 214.1269169785269924 ) ) ;
#107385=CARTESIAN_POINT ( 'NONE',  ( 7.712015721893069831, 1516.648258902369889, 208.0703445135380036 ) ) ;
#107387=LINE ( 'NONE', #30683, #10640 ) ;
#107410=CARTESIAN_POINT ( 'NONE',  ( -3.279658057385000269, 1511.011611623890076, 201.5574319706369977 ) ) ;
#107426=CARTESIAN_POINT ( 'NONE',  ( 3.487586588097512319, 1508.731359868794925, 213.6768079589742513 ) ) ;
#107448=CARTESIAN_POINT ( 'NONE',  ( -7.937147302369870872, 1511.433279536600139, 214.9445374233650057 ) ) ;
#107452=EDGE_CURVE ( 'NONE', #44905, #104774, #79398, .T. ) ;
#107453=CARTESIAN_POINT ( 'NONE',  ( -0.01012492377659850000, 1516.989863902050047, 207.9939175986969815 ) ) ;
#107464=CARTESIAN_POINT ( 'NONE',  ( -15.08187219341120056, 1512.240709848920005, 221.7951975401620075 ) ) ;
#107485=ORIENTED_EDGE ( 'NONE', *, *, #61646, .T. ) ;
#107491=CARTESIAN_POINT ( 'NONE',  ( 2.868433798504999910, 1517.020727862619879, 204.1095288638669842 ) ) ;
#107492=VECTOR ( 'NONE', #13828, 1000.000000000000114 ) ;
#107502=CARTESIAN_POINT ( 'NONE',  ( 4.832616789874995433, 1508.551704408610021, 205.6342609684716933 ) ) ;
#107505=CARTESIAN_POINT ( 'NONE',  ( -13.52455581696280085, 1512.715996828740117, 193.8118672836219787 ) ) ;
#107545=DIRECTION ( 'NONE',  ( -1.000000000000000000, 0.000000000000000000, 0.000000000000000000 ) ) ;
#107559=ORIENTED_EDGE ( 'NONE', *, *, #101568, .F. ) ;
#107589=CARTESIAN_POINT ( 'NONE',  ( -3.747637931291374347, 1511.538143005324173, 201.0064871382184890 ) ) ;
#107598=CARTESIAN_POINT ( 'NONE',  ( -5.011367984924999242, 1516.974592746400049, 205.6720686163770324 ) ) ;
#107607=VERTEX_POINT ( 'NONE', #83245 ) ;
#107612=CARTESIAN_POINT ( 'NONE',  ( -2.476170635034999901, 1516.819260244609950, 210.8389306816469855 ) ) ;
#107630=CARTESIAN_POINT ( 'NONE',  ( 16.77415063058788292, 1513.652806712936126, 195.7035532396738517 ) ) ;
#107634=CIRCLE ( 'NONE', #28911, 1.000000000039231285 ) ;
#107645=CARTESIAN_POINT ( 'NONE',  ( -4.626591905484999323, 1517.096587378560116, 207.4170511287669854 ) ) ;
#107651=DIRECTION ( 'NONE',  ( -0.02616798426500965835, 0.9993150019883683122, 0.02616798426500955774 ) ) ;
#107657=CARTESIAN_POINT ( 'NONE',  ( -6.191282293671606318, 1510.848430435494720, 201.6637636903093949 ) ) ;
#107663=CARTESIAN_POINT ( 'NONE',  ( -2.872208748294999836, 1517.145312756229941, 216.4596396827270155 ) ) ;
#107665=FACE_OUTER_BOUND ( 'NONE', #2712, .T. ) ;
#107668=CARTESIAN_POINT ( 'NONE',  ( -4.029572678834999699, 1516.858649670339901, 213.1633184439769764 ) ) ;
#107673=ORIENTED_EDGE ( 'NONE', *, *, #2359, .T. ) ;
#107687=CARTESIAN_POINT ( 'NONE',  ( -6.947377821305000367, 1517.009964551830080, 204.5062011277169916 ) ) ;
#107724=CARTESIAN_POINT ( 'NONE',  ( -11.12931925036500047, 1512.151624459629829, 193.3374815694669735 ) ) ;
#107728=CARTESIAN_POINT ( 'NONE',  ( -5.005071046424999892, 1516.710692850270107, 201.7963041449669959 ) ) ;
#107731=CARTESIAN_POINT ( 'NONE',  ( 15.48184689783500012, 1513.486273623730085, 194.4742589842670100 ) ) ;
#107764=CARTESIAN_POINT ( 'NONE',  ( 3.261635932824999973, 1516.613881697390070, 216.0569793506570022 ) ) ;
#107766=ORIENTED_EDGE ( 'NONE', *, *, #63840, .T. ) ;
#107771=CARTESIAN_POINT ( 'NONE',  ( 2.284199363404999961, 1516.940296199220029, 205.8526610237369994 ) ) ;
#107773=CARTESIAN_POINT ( 'NONE',  ( 5.011551368014999674, 1517.080322339569875, 209.8587501411369942 ) ) ;
#107787=CARTESIAN_POINT ( 'NONE',  ( -4.028307778284999863, 1516.797038924770050, 212.3881954442970255 ) ) ;
#107789=EDGE_CURVE ( 'NONE', #29868, #8432, #86655, .T. ) ;
#107793=CARTESIAN_POINT ( 'NONE',  ( -7.711161960695579687, 1516.615653621549882, 210.3347488552499840 ) ) ;
#107794=CARTESIAN_POINT ( 'NONE',  ( 5.014195101815000832, 1517.120861839400050, 210.8273123806970091 ) ) ;
#107806=CARTESIAN_POINT ( 'NONE',  ( -5.778999811904999895, 1516.955859323880077, 216.4549161051170074 ) ) ;
#107811=CARTESIAN_POINT ( 'NONE',  ( 3.259729297834999873, 1517.119374999550018, 201.7846921639870175 ) ) ;
#107813=CARTESIAN_POINT ( 'NONE',  ( -15.78436440076499991, 1512.151624459629829, 220.2511651824670196 ) ) ;
#107819=CARTESIAN_POINT ( 'NONE',  ( 7.663889412338700247, 1510.954290761809943, 203.6521466954270068 ) ) ;
#107829=ORIENTED_EDGE ( 'NONE', *, *, #61921, .T. ) ;
#107830=LINE ( 'NONE', #89379, #5199 ) ;
#107838=PLANE ( 'NONE',  #3838 ) ;
#107845=CARTESIAN_POINT ( 'NONE',  ( 14.97085957818899971, 1514.147575501549909, 223.8949061397489970 ) ) ;
#107867=B_SPLINE_CURVE_WITH_KNOTS ( 'NONE', 3,
 ( #35018, #52402, #43436, #50194, #110627, #85976, #17637, #86525, #59689, #33352, #8704, #75924, #42321, #1427, #77587, #27181, #67547, #26045, #17078, #61364, #69197, #42882, #51273, #60808, #78123, #101649, #93801, #77039, #16532 ),
 .UNSPECIFIED., .F., .F.,
 ( 4, 2, 2, 1, 1, 2, 2, 2, 2, 2, 2, 2, 1, 2, 2, 4 ),
 ( 0.000000000000000000, 0.1250000000036102510, 0.1875000000054153904, 0.2187500000062866101, 0.2343750000067222339, 0.2421875000068499373, 0.2500000000069776407, 0.3750000000063050121, 0.4375000000059334204, 0.5000000000055617733, 0.6250000000043715032, 0.6875000000035829117, 0.7187500000030055958, 0.7343750000027402525, 0.7500000000024747981, 1.000000000000000000 ),
 .UNSPECIFIED. ) ;
#107883=CARTESIAN_POINT ( 'NONE',  ( -1.700706814495000163, 1516.923170579120097, 211.4225755968969906 ) ) ;
#107886=CARTESIAN_POINT ( 'NONE',  ( 1.715361092244999996, 1516.743010792419909, 212.5670474586069929 ) ) ;
#107893=CARTESIAN_POINT ( 'NONE',  ( 0.7386049046750020608, 1517.122674412569950, 202.5597518628069906 ) ) ;
#107902=ORIENTED_EDGE ( 'NONE', *, *, #90545, .F. ) ;
#107909=CARTESIAN_POINT ( 'NONE',  ( -6.548200625775000283, 1516.632821972880038, 210.2524534341069966 ) ) ;
#107914=CARTESIAN_POINT ( 'NONE',  ( 8.170896223665000235, 1511.354819475749991, 204.2943405042869927 ) ) ;
#107916=CARTESIAN_POINT ( 'NONE',  ( -3.269184946495000244, 1516.940296199220029, 206.8376465686969823 ) ) ;
#107923=CYLINDRICAL_SURFACE ( 'NONE', #92790, 1.999999999999997335 ) ;
#107930=CARTESIAN_POINT ( 'NONE',  ( 7.649034400464999273, 1514.243099272629934, 214.7715657207469917 ) ) ;
#107935=LINE ( 'NONE', #88931, #22657 ) ;
#107937=CARTESIAN_POINT ( 'NONE',  ( 0.7533001353030019942, 1516.714320817460020, 216.4479181143769893 ) ) ;
#107963=CARTESIAN_POINT ( 'NONE',  ( -5.106974084935000491, 1511.397837225850026, 200.5635451951269772 ) ) ;
#107968=VERTEX_POINT ( 'NONE', #8533 ) ;
#107991=CARTESIAN_POINT ( 'NONE',  ( -7.320051284198429542, 1508.610505975320166, 215.2032464672789729 ) ) ;
#107998=CARTESIAN_POINT ( 'NONE',  ( -8.631375286013071246, 1511.600151312669823, 215.0326715986050203 ) ) ;
#108003=CARTESIAN_POINT ( 'NONE',  ( 4.028611221114998919, 1516.744381837270112, 207.9874879615069858 ) ) ;
#108030=CARTESIAN_POINT ( 'NONE',  ( 3.487586701839819892, 1508.731366863229823, 204.5668911354170234 ) ) ;
#108039=CARTESIAN_POINT ( 'NONE',  ( 0.7365611785030020675, 1517.066898074209803, 204.4979538714769944 ) ) ;
#108042=CARTESIAN_POINT ( 'NONE',  ( 14.79494652412309819, 1512.129944624190102, 196.8603049394490085 ) ) ;
#108049=CARTESIAN_POINT ( 'NONE',  ( -12.92498210531170066, 1512.351864386150055, 193.9290602599010072 ) ) ;
#108073=FACE_OUTER_BOUND ( 'NONE', #84026, .T. ) ;
#108081=CARTESIAN_POINT ( 'NONE',  ( 11.02428137105887807, 1512.359593911811089, 224.9978793913905974 ) ) ;
#108087=B_SPLINE_CURVE_WITH_KNOTS ( 'NONE', 5,
 ( #63096, #29433, #9880, #10996, #45168, #104497 ),
 .UNSPECIFIED., .F., .F.,
 ( 6, 6 ),
 ( 4.250950522270000143, 7.082025451739999866 ),
 .UNSPECIFIED. ) ;
#108125=FILL_AREA_STYLE ('',( #56089 ) ) ;
#108128=EDGE_CURVE ( 'NONE', #71147, #84553, #18624, .T. ) ;
#108134=CARTESIAN_POINT ( 'NONE',  ( -4.598104748810852627, 1511.399590460244326, 200.7322199627068642 ) ) ;
#108142=CARTESIAN_POINT ( 'NONE',  ( -4.622842882315000068, 1516.901952101700090, 205.0913314195169903 ) ) ;
#108158=CARTESIAN_POINT ( 'NONE',  ( -0.7374509209069979310, 1516.978425811520083, 210.2554991112269818 ) ) ;
#108163=PRODUCT_DEFINITION_SHAPE ( 'NONE', 'NONE',  #102745 ) ;
#108183=CARTESIAN_POINT ( 'NONE',  ( 1.708747624254999931, 1517.213554313520035, 202.1696795498070003 ) ) ;
#108184=CARTESIAN_POINT ( 'NONE',  ( -5.788691363644999477, 1517.157901477309906, 207.9987443536870160 ) ) ;
#108197=CARTESIAN_POINT ( 'NONE',  ( -5.863482209052399696, 1511.603576927810082, 200.6690587505990209 ) ) ;
#108200=DIRECTION ( 'NONE',  ( -0.7384854939285241393, 0.000000000000000000, 0.6742693640208961003 ) ) ;
#108205=CARTESIAN_POINT ( 'NONE',  ( 0.7526715501680020237, 1516.710624944440042, 216.8354948044169817 ) ) ;
#108211=CARTESIAN_POINT ( 'NONE',  ( -2.284526496774999860, 1516.956048353049937, 212.5847947667770086 ) ) ;
#108215=ORIENTED_EDGE ( 'NONE', *, *, #75832, .T. ) ;
#108219=CARTESIAN_POINT ( 'NONE',  ( -4.329790274010359319, 1515.051704408389696, 205.2060425482763151 ) ) ;
#108229=CARTESIAN_POINT ( 'NONE',  ( -6.561686461364999445, 1517.069378699710114, 205.6695567495270041 ) ) ;
#108264=EDGE_CURVE ( 'NONE', #49508, #27633, #60958, .T. ) ;
#108267=ORIENTED_EDGE ( 'NONE', *, *, #72159, .T. ) ;
#108278=CARTESIAN_POINT ( 'NONE',  ( 7.715625202974999652, 1516.786099423779888, 202.5670817708370066 ) ) ;
#108281=CARTESIAN_POINT ( 'NONE',  ( 16.64927606573499830, 1512.799725290110018, 197.0740121610670030 ) ) ;
#108315=CARTESIAN_POINT ( 'NONE',  ( 7.330554133425000174, 1516.857992118400034, 216.4511490482170188 ) ) ;
#108317=EDGE_CURVE ( 'NONE', #74608, #94671, #3634, .T. ) ;
#108324=CARTESIAN_POINT ( 'NONE',  ( -0.7572979743539989261, 1516.829948096479939, 205.6721984920870057 ) ) ;
#108326=CARTESIAN_POINT ( 'NONE',  ( -6.562094107424999656, 1517.122674412569950, 208.3832410274270046 ) ) ;
#108339=CARTESIAN_POINT ( 'NONE',  ( -2.866857931135000204, 1516.951766529250108, 213.1652121904069759 ) ) ;
#108341=EDGE_CURVE ( 'NONE', #86690, #76843, #94958, .T. ) ;
#108345=CARTESIAN_POINT ( 'NONE',  ( -7.715586062468250184, 1516.784603496080081, 209.6398392507250321 ) ) ;
#108346=CARTESIAN_POINT ( 'NONE',  ( 3.269025135755000200, 1517.026534522949987, 210.2412850599169758 ) ) ;
#108362=CARTESIAN_POINT ( 'NONE',  ( -7.329303116114999739, 1516.857992118400034, 216.4524001036569985 ) ) ;
#108366=ORIENTED_EDGE ( 'NONE', *, *, #86, .T. ) ;
#108367=CARTESIAN_POINT ( 'NONE',  ( -2.873329398885000163, 1516.572193931679976, 201.7997408644770019 ) ) ;
#108368=CARTESIAN_POINT ( 'NONE',  ( -15.46640442256500059, 1511.810036768419877, 221.1669702143669838 ) ) ;
#108413=CARTESIAN_POINT ( 'NONE',  ( 13.72878283421173506, 1517.051704408389924, 191.9723449582409955 ) ) ;
#108443=CARTESIAN_POINT ( 'NONE',  ( -4.995726007844999650, 1516.651306816259876, 211.4173314712770093 ) ) ;
#108447=CARTESIAN_POINT ( 'NONE',  ( -7.710610441124999603, 1516.594591938570147, 212.5759658869370128 ) ) ;
#108454=CARTESIAN_POINT ( 'NONE',  ( 5.002593359325000044, 1516.960844870249957, 202.5626772953570196 ) ) ;
#108462=VERTEX_POINT ( 'NONE', #51859 ) ;
#108468=CARTESIAN_POINT ( 'NONE',  ( 6.563254890855000134, 1517.139039350860003, 211.6051684241269868 ) ) ;
#108473=CARTESIAN_POINT ( 'NONE',  ( 7.548380872364999661, 1510.399296111369949, 204.3167683741870064 ) ) ;
#108475=CARTESIAN_POINT ( 'NONE',  ( 2.476170596904999854, 1516.819260244609950, 207.4047612206870213 ) ) ;
#108476=ORIENTED_EDGE ( 'NONE', *, *, #18017, .F. ) ;
#108493=CARTESIAN_POINT ( 'NONE',  ( -2.484577695354999616, 1517.170512887980067, 216.4602579296269766 ) ) ;
#108520=CARTESIAN_POINT ( 'NONE',  ( -3.481979457305000025, 1511.353635254350138, 201.3868063830669826 ) ) ;
#108525=EDGE_LOOP ( 'NONE', ( #13494, #35302, #3862, #35447, #28704, #69092, #22847, #91914, #104607, #89592 ) ) ;
#108527=EDGE_CURVE ( 'NONE', #47285, #2864, #42902, .T. ) ;
#108563=CARTESIAN_POINT ( 'NONE',  ( -5.006259886824999228, 1516.939723362869927, 209.1347437590049765 ) ) ;
#108567=EDGE_CURVE ( 'NONE', #43145, #11042, #33666, .T. ) ;
#108593=CARTESIAN_POINT ( 'NONE',  ( 4.802243920988390258, 1508.551704408389924, 204.6921040114409891 ) ) ;
#108600=CARTESIAN_POINT ( 'NONE',  ( -4.333361549047180183, 1508.551704406479985, 204.4537186006569982 ) ) ;
#108602=CARTESIAN_POINT ( 'NONE',  ( -3.266349512195000138, 1516.797038924770050, 205.0935381919470046 ) ) ;
#108610=CARTESIAN_POINT ( 'NONE',  ( -13.64573741497510184, 1512.804203059160045, 193.8098271449230197 ) ) ;
#108622=CARTESIAN_POINT ( 'NONE',  ( -7.645478605405000572, 1514.134513140259969, 203.0666490157069859 ) ) ;
#108684=CARTESIAN_POINT ( 'NONE',  ( -7.717505791104999346, 1516.857914730730045, 216.8393517232070167 ) ) ;
#108691=CARTESIAN_POINT ( 'NONE',  ( -3.858625071233336978, 1511.506728505285992, 200.9714742573962951 ) ) ;
#108698=CARTESIAN_POINT ( 'NONE',  ( 6.935133380425000382, 1516.613881697390070, 205.8602099992770036 ) ) ;
#108713=CARTESIAN_POINT ( 'NONE',  ( -5.775625115495000017, 1516.745833913490060, 209.8771724060850090 ) ) ;
#108741=CARTESIAN_POINT ( 'NONE',  ( 6.941727252324999320, 1516.882217593000178, 201.7906628411569727 ) ) ;
#108742=CARTESIAN_POINT ( 'NONE',  ( -1.715109485185000171, 1516.963431999339946, 208.3866188148990091 ) ) ;
#108752=CARTESIAN_POINT ( 'NONE',  ( -6.013128445097610353, 1510.874996213040049, 201.6036617501539752 ) ) ;
#108760=CARTESIAN_POINT ( 'NONE',  ( 6.942344691835000248, 1516.810037859429940, 216.8380980232070101 ) ) ;
#108765=CARTESIAN_POINT ( 'NONE',  ( -1.703779643355000095, 1517.057265928030120, 213.1670284501570052 ) ) ;
#108768=CARTESIAN_POINT ( 'NONE',  ( 3.861651023821930373, 1508.610718263850003, 213.8016401658969983 ) ) ;
#108784=CARTESIAN_POINT ( 'NONE',  ( -5.786837717054999608, 1517.040132827679827, 205.8646253294070050 ) ) ;
#108785=VECTOR ( 'NONE', #106485, 999.9999999999998863 ) ;
#108807=CARTESIAN_POINT ( 'NONE',  ( -15.00581081485931279, 1514.742480524781740, 193.0300471132391351 ) ) ;
#108828=CARTESIAN_POINT ( 'NONE',  ( -7.330554171554999776, 1516.857992118400034, 201.7925428541169879 ) ) ;
#108831=CARTESIAN_POINT ( 'NONE',  ( 15.24995204913500046, 1513.868118914750085, 194.1593619713669909 ) ) ;
#108855=CARTESIAN_POINT ( 'NONE',  ( 8.640072888135000184, 1511.773927532309926, 202.9615657546970056 ) ) ;
#108865=CARTESIAN_POINT ( 'NONE',  ( -4.033653302454999867, 1517.028034847769959, 215.6825881955670070 ) ) ;
#108875=CARTESIAN_POINT ( 'NONE',  ( 1.119439089684999944, 1517.026534522949987, 205.8528207963470038 ) ) ;
#108877=CARTESIAN_POINT ( 'NONE',  ( 1.709766494024999917, 1516.959716008189844, 209.1091877442879934 ) ) ;
#108883=CARTESIAN_POINT ( 'NONE',  ( 5.513435558014999849, 1509.038615934239942, 216.6345961781970288 ) ) ;
#108889=CARTESIAN_POINT ( 'NONE',  ( 2.490245914424999985, 1516.691389976299888, 213.7302634767470124 ) ) ;
#108893=CARTESIAN_POINT ( 'NONE',  ( 7.444963622127359848, 1508.731180391300086, 214.6350537489069836 ) ) ;
#108895=CARTESIAN_POINT ( 'NONE',  ( 3.269984781304999810, 1516.999105586269934, 210.8242519552970009 ) ) ;
#108913=CARTESIAN_POINT ( 'NONE',  ( 6.554764161265000055, 1516.786099423779888, 216.8374711732070068 ) ) ;
#108918=CARTESIAN_POINT ( 'NONE',  ( -6.943602691585000208, 1516.858069504249897, 202.1807456543569685 ) ) ;
#108943=CARTESIAN_POINT ( 'NONE',  ( -4.668127369574689212, 1508.551704406479985, 213.4552074811490172 ) ) ;
#108949=AXIS2_PLACEMENT_3D ( 'NONE', #71636, #88933, #61556 ) ;
#108950=EDGE_CURVE ( 'NONE', #106739, #29094, #84207, .T. ) ;
#108962=VERTEX_POINT ( 'NONE', #75283 ) ;
#108972=CARTESIAN_POINT ( 'NONE',  ( 12.39098288733500119, 1517.051704408389924, 218.3803088333170024 ) ) ;
#108992=CARTESIAN_POINT ( 'NONE',  ( 5.513435558014999849, 1509.038615934239942, 216.6345961781970288 ) ) ;
#109001=CARTESIAN_POINT ( 'NONE',  ( 5.787476994515000861, 1517.070197312179971, 211.9915394291670054 ) ) ;
#109002=ADVANCED_FACE ( 'NONE', ( #11923 ), #95540, .F. ) ;
#109005=CARTESIAN_POINT ( 'NONE',  ( -1.702754409475000008, 1517.014196759610059, 212.5856132281170119 ) ) ;
#109008=AXIS2_PLACEMENT_3D ( 'NONE', #31488, #91413, #106557 ) ;
#109013=CARTESIAN_POINT ( 'NONE',  ( -4.037378294184999383, 1516.688761843659904, 202.5730239910470232 ) ) ;
#109017=CARTESIAN_POINT ( 'NONE',  ( -7.487063421429379417, 1517.051703294439903, 208.6815157772669806 ) ) ;
#109033=CARTESIAN_POINT ( 'NONE',  ( -2.863787893864999656, 1516.788317650260069, 210.8382387120070121 ) ) ;
#109039=CARTESIAN_POINT ( 'NONE',  ( -2.299983615734999987, 1516.861367446839949, 206.8392230197369770 ) ) ;
#109041=CARTESIAN_POINT ( 'NONE',  ( 7.709151570915000029, 1516.538881389200014, 206.5697199716970260 ) ) ;
#109059=CARTESIAN_POINT ( 'NONE',  ( 3.454748808194999743, 1516.609912606490070, 216.4448802441970088 ) ) ;
#109095=ORIENTED_EDGE ( 'NONE', *, *, #18017, .T. ) ;
#109134=CARTESIAN_POINT ( 'NONE',  ( 0.7468175155120010400, 1517.006509894990131, 209.1147170949500094 ) ) ;
#109138=B_SPLINE_SURFACE_WITH_KNOTS ( 'NONE', 5, 5, ( 
 ( #54684, #27247, #10443, #44614, #96667, #35089, #19938, #61428, #69271, #54134, #26680, #95551, #18824, #79868, #60879, #3179, #71505, #105624, #9345, #81489, #73684, #98854, #21025, #80960, #63639, #13725, #48480, #47362, #88810, #97753, #5351, #82046, #107256 ),
 ( #4262, #21578, #55786, #40055, #37860, #98302, #91000, #56871, #39511, #107811, #13173, #72046, #89902, #106163, #22670, #46831, #74236, #30551, #29440, #22117, #99392, #64740, #108367, #4790, #38936, #55228, #56315, #90448, #38395, #89358, #47911, #12653, #72571 ),
 ( #106698, #82618, #31098, #73116, #14290, #65280, #5909, #29990, #31648, #65830, #99947, #64181, #23242, #12094, #46288, #80416, #3730, #32210, #59629, #67489, #101593, #42265, #7002, #59086, #75870, #41711, #57441, #92112, #49578, #15388, #108918, #66937, #66391 ),
 ( #6459, #100510, #83709, #32755, #40607, #75336, #23789, #110020, #49031, #50131, #76414, #24878, #57978, #41161, #109477, #93206, #17018, #15930, #91566, #101045, #84799, #50667, #33296, #110568, #33853, #93740, #16476, #8097, #14842, #68044, #24345, #51217, #83166 ),
 ( #92656, #74778, #58528, #84260, #102154, #7556, #42820, #25433, #85348, #8645, #76980, #289, #34414, #68586, #102691, #9223, #10883, #10312, #11436, #51781, #9760, #44486, #36084, #18695, #45607, #27128, #60751, #1374, #103247, #70824, #45055, #78631, #43381 ),
 ( #79749, #18151, #35517, #27674, #70269, #1946, #2505, #78071, #52892, #52346, #104936, #79199, #36626, #104378, #28223, #61859, #87020, #26558, #95979, #94303, #34959, #19240, #3056, #37182, #71379, #831, #103828, #61314, #53450, #85919, #87595, #69143, #77530 ),
 ( #25986, #62411, #96538, #19812, #94874, #86467, #95432, #69709, #54018, #88148, #60186, #43924, #17581, #54563, #107130, #22538, #64055, #89232, #105490, #81919, #37728, #56180, #80835, #71932, #97637, #38267, #72452, #56740, #88697, #4143, #107687, #73553, #90318 ),
 ( #81363, #14164, #65147, #106582, #47785, #106044, #20358, #39378, #48349, #11978, #29869, #38816, #72992, #46705, #98175, #39931, #90875, #20906, #82488, #5225, #21445, #28781, #98727, #62982, #97093, #46159, #55655, #80290, #89778, #99260, #5790, #30421, #3605 ),
 ( #55107, #13047, #64608, #4677, #21988, #30971, #47236, #13596, #12527, #29321, #63521, #58944, #15787, #42137, #84125, #7424, #41590, #66267, #48907, #33169, #57314, #40474, #31516, #75745, #16891, #109889, #66809, #100910, #76287, #108229, #93612, #100384, #67359 ),
 ( #57852, #91441, #101456, #6862, #24745, #32077, #24208, #58394, #14717, #92520, #51096, #93074, #91980, #83034, #16348, #41023, #50546, #23669, #6325, #110437, #84671, #7970, #33715, #15255, #67909, #49989, #102017, #74100, #108784, #49446, #83570, #74649, #75201 ),
 ( #25300, #23110, #109352, #32633, #59501, #85221, #8513, #65698, #99815, #34278, #35383, #27535, #52752, #85781, #34827, #17446, #78496, #2371, #1245, #42686, #51643, #70133, #35947, #61180, #61718, #95840, #79066, #1811, #104245, #76844, #86885, #94735, #44919 ),
 ( #70683, #18558, #62271, #36486, #43788, #19107, #9080, #68459, #87452, #96400, #25856, #52206, #10179, #44354, #18013, #86333, #88018, #28083, #69014, #19676, #53311, #9619, #156, #10747, #102563, #60057, #94175, #77938, #43247, #69571, #104796, #53881, #77396 ),
 ( #698, #103119, #26420, #103691, #26991, #95297, #60612, #96957, #72853, #20764, #64468, #106987, #4543, #106446, #81228, #21849, #20223, #54963, #105910, #98030, #30275, #79612, #29729, #37589, #72314, #54424, #98583, #55507, #89090, #38677, #11840, #46011, #105350 ),
 ( #37033, #56046, #71228, #28640, #80142, #71791, #62844, #29189, #88557, #80698, #2916, #12377, #89635, #63915, #3461, #63380, #97496, #21302, #90173, #46564, #11302, #4008, #12922, #47102, #38133, #14980, #49175, #45470, #36289, #70481, #510, #44716, #52558 ),
 ( #62078, #27895, #35743, #60409, #9986, #17801, #45272, #69371, #96764, #18916, #94527, #10542, #11111, #53114, #20034, #104043, #27335, #52002, #96204, #95649, #54229, #26220, #95098, #87251, #78868, #61521, #88356, #1606, #35186, #86692, #77750, #79410, #19479 ),
 ( #36844, #105157, #2174, #102920, #104602, #44156, #69930, #78292, #43599, #2722, #53681, #28449, #71036, #62643, #87823, #11645, #45822, #1059, #34635, #68819, #86142, #9435, #103480, #26785, #18364, #60973, #82008, #41117, #32168, #108326, #92074, #74195, #65787 ),
 ( #6423, #40015, #74739, #31609, #23755, #47871, #6964, #5313, #99907, #39471, #23203, #37402, #90405, #108877, #58487, #101008, #24307, #56275, #48442, #75296, #32720, #40568, #64699, #66354, #66901, #73643, #90965, #83125, #91529, #57402, #57942, #22626, #14807 ),
 ( #109441, #15347, #48993, #49542, #92615, #107773, #100472, #14252, #83667, #15892, #71601, #79955, #99351, #3272, #31059, #105722, #30509, #98817, #22079, #13684, #65240, #56830, #82582, #5873, #39861, #81847, #4612, #38746, #108713, #72924, #22471, #107063, #99191 ),
 ( #57238, #21919, #74025, #90807, #56671, #72385, #30347, #64538, #98654, #12987, #5151, #47170, #48834, #30896, #49369, #48277, #74577, #108158, #81298, #98102, #65075, #13530, #91369, #14088, #39306, #21374, #31448, #55583, #65631, #100312, #82422, #56115, #106514 ),
 ( #99745, #5716, #14648, #82957, #32004, #23036, #6251, #29803, #40400, #47717, #66192, #63991, #23597, #57786, #91904, #15181, #83496, #73479, #6792, #90248, #89706, #107612, #60539, #24130, #50478, #85153, #8439, #93000, #84602, #86259, #26343, #67287, #94661 ),
 ( #25230, #51019, #33637, #17932, #42065, #75675, #16276, #7353, #85704, #76765, #40953, #42612, #7893, #43173, #75130, #34205, #68945, #16818, #52130, #625, #76215, #94102, #84054, #66738, #9000, #109279, #58321, #110360, #75, #68389, #67832, #101942, #32562 ),
 ( #100841, #51571, #59433, #92444, #102496, #15719, #49920, #41516, #93545, #109819, #25786, #34756, #103045, #59985, #33098, #17373, #101379, #24672, #77326, #58870, #19602, #96324, #98385, #61640, #2297, #35874, #55864, #30071, #106780, #62197, #89985, #53804, #87941 ),
 ( #95221, #79533, #103618, #86816, #77870, #11232, #64823, #45394, #36408, #70600, #13258, #43718, #30636, #1735, #2836, #36957, #71152, #19036, #52679, #10107, #47448, #44280, #104718, #78424, #28009, #1179, #18483, #64261, #98931, #22204, #56400, #70058, #87379 ),
 ( #104169, #61104, #53237, #27455, #21656, #78994, #9548, #81572, #4875, #39018, #95770, #35309, #73195, #10673, #107340, #69496, #44839, #26916, #15465, #39592, #92192, #7629, #49108, #74317, #90532, #67016, #22752, #41243, #65914, #56956, #82695, #23323, #7087 ),
 ( #100032, #91083, #5985, #57516, #91640, #41787, #73763, #14916, #92738, #58605, #75416, #109554, #83242, #107886, #6536, #31177, #24420, #48559, #75945, #109005, #65366, #100582, #101123, #32290, #110097, #40688, #74861, #99472, #32826, #66474, #33372, #5434, #108447 ),
 ( #83793, #47994, #13808, #82131, #23864, #14365, #58058, #50214, #67566, #49658, #40133, #16013, #101670, #31727, #84341, #24959, #69218, #35040, #35593, #370, #51861, #85425, #103902, #78147, #44008, #915, #27202, #103328, #26635, #60831, #51291, #33931, #18225 ),
 ( #77061, #94955, #59710, #18773, #9843, #85997, #69784, #9296, #43459, #42341, #77607, #2023, #93288, #25516, #93823, #1448, #102774, #52420, #17098, #68128, #61384, #86547, #95503, #52971, #8725, #87103, #10391, #44561, #59169, #42904, #34495, #68670, #110645 ),
 ( #8172, #78710, #76494, #102241, #26065, #60260, #94379, #17660, #36158, #70342, #50741, #104454, #16551, #84877, #70897, #19885, #2581, #63591, #98256, #97159, #27746, #36703, #87668, #29390, #55737, #20430, #11511, #61938, #4214, #105014, #89311, #3132, #28304 ),
 ( #97708, #20981, #96057, #72000, #79825, #29943, #19326, #55185, #89859, #3685, #47312, #21525, #28862, #80916, #62497, #53528, #72523, #81435, #10957, #37262, #106113, #12606, #71460, #105574, #73071, #13128, #54092, #4746, #38344, #63055, #45129, #46786, #79271 ),
 ( #54637, #96618, #88768, #38889, #88217, #106652, #45686, #64135, #12052, #46236, #80369, #37811, #6411, #83117, #83657, #48432, #99895, #22616, #41109, #15337, #92065, #48984, #75286, #40557, #74731, #108865, #99341, #81996, #66345, #90394, #73633, #64689, #32158 ),
 ( #57932, #23193, #6952, #57392, #91518, #13672, #14798, #50081, #30500, #107764, #31048, #49532, #40006, #100461, #65230, #5303, #109432, #23744, #32709, #66890, #56820, #100999, #24295, #58478, #107212, #90956, #14243, #82573, #47862, #5865, #39461, #92605, #56265 ),
 ( #74184, #108315, #31599, #65778, #15878, #98807, #84210, #7506, #41668, #22068, #67997, #68544, #60139, #59037, #94259, #18648, #109976, #42220, #110521, #94826, #8600, #85871, #33803, #50622, #78023, #9172, #43337, #60702, #25388, #77485, #17533, #51735, #75825 ),
 ( #785, #34915, #93159, #101543, #69660, #9712, #24832, #84755, #102109, #51173, #16430, #93694, #8052, #69100, #67444, #102643, #18102, #103202, #76372, #59581, #16974, #26507, #35470, #34370, #33253, #85302, #52297, #86422, #43879, #1330, #103783, #27084, #61269 ) ),
 .UNSPECIFIED., .F., .F., .F.,
 ( 6, 3, 3, 3, 3, 3, 3, 3, 3, 3, 6 ),
 ( 6, 3, 3, 3, 3, 3, 3, 3, 3, 3, 6 ),
 ( 0.000000000000000000, 1.936717162300000128, 3.873434324599999812, 4.841792905749999321, 5.810151486899999718, 7.746868649199999624, 9.683585811500000418, 10.65194439270000082, 11.62030297379999944, 13.55702013610000023, 15.49373729840000102 ),
 ( 0.000000000000000000, 1.936717162300000128, 3.873434324599999812, 4.841792905749999321, 5.810151486899999718, 7.746868649199999624, 9.683585811500000418, 10.65194439270000082, 11.62030297379999944, 13.55702013610000023, 15.49373729840000102 ),
 .UNSPECIFIED. ) ;
#109167=CARTESIAN_POINT ( 'NONE',  ( -4.987080977031280504, 1508.551704408389924, 205.1632012944579913 ) ) ;
#109169=CARTESIAN_POINT ( 'NONE',  ( 4.028630584655000568, 1516.812923327049930, 205.6617440802170051 ) ) ;
#109172=CARTESIAN_POINT ( 'NONE',  ( 15.29936282157690108, 1512.951873711579992, 195.2879060687520223 ) ) ;
#109179=CARTESIAN_POINT ( 'NONE',  ( -14.49132061573049945, 1513.569700116999911, 194.0178397853109971 ) ) ;
#109221=ADVANCED_FACE ( 'NONE', ( #71468 ), #12060, .F. ) ;
#109259=CARTESIAN_POINT ( 'NONE',  ( -5.130014241433883626, 1511.406470015445620, 200.5554185186313134 ) ) ;
#109264=CARTESIAN_POINT ( 'NONE',  ( 1.119439089684999944, 1517.026534522949987, 205.8528207963470038 ) ) ;
#109274=CARTESIAN_POINT ( 'NONE',  ( -16.75056594176211533, 1513.749562442875913, 222.7143392581427008 ) ) ;
#109279=CARTESIAN_POINT ( 'NONE',  ( -4.026777524084999449, 1516.718889242609976, 211.4189316860469887 ) ) ;
#109298=DIRECTION ( 'NONE',  ( -1.000000000000000000, 0.000000000000000000, 0.000000000000000000 ) ) ;
#109306=CARTESIAN_POINT ( 'NONE',  ( -4.035490750684999739, 1516.630499592039996, 201.4102952541169884 ) ) ;
#109307=CARTESIAN_POINT ( 'NONE',  ( -3.462835665494999660, 1517.038650117239968, 208.0021282158369900 ) ) ;
#109311=CARTESIAN_POINT ( 'NONE',  ( 4.607425546304328989, 1511.399183828327523, 217.5145368139657478 ) ) ;
#109327=CARTESIAN_POINT ( 'NONE',  ( -3.453544863754999472, 1517.106845464700200, 216.4586906126469898 ) ) ;
#109333=CARTESIAN_POINT ( 'NONE',  ( 5.008848199894999631, 1516.858456333729919, 214.1219297979669989 ) ) ;
#109337=CARTESIAN_POINT ( 'NONE',  ( 4.987078416403489811, 1508.551704408389924, 212.6094303565780024 ) ) ;
#109352=CARTESIAN_POINT ( 'NONE',  ( 6.934528529765000116, 1516.588006113850042, 206.2478870805069846 ) ) ;
#109360=CIRCLE ( 'NONE', #61106, 6.500000000000000000 ) ;
#109361=ADVANCED_FACE ( 'NONE', ( #73517 ), #57278, .F. ) ;
#109372=VECTOR ( 'NONE', #33193, 1000.000000000000114 ) ;
#109375=CARTESIAN_POINT ( 'NONE',  ( -12.99081176452876285, 1513.436191188001885, 192.3341863405429990 ) ) ;
#109388=CARTESIAN_POINT ( 'NONE',  ( -2.234923082067399758, 1512.341036938790012, 201.5226187867249905 ) ) ;
#109390=CARTESIAN_POINT ( 'NONE',  ( -7.459190136973458785, 1510.844697586386246, 215.3093670277948775 ) ) ;
#109394=CARTESIAN_POINT ( 'NONE',  ( -15.02579306586500074, 1513.907445464720013, 193.7166317783670024 ) ) ;
#109399=CARTESIAN_POINT ( 'NONE',  ( -0.01171164408179850049, 1516.939568781210028, 202.5649949355269825 ) ) ;
#109402=CARTESIAN_POINT ( 'NONE',  ( 15.99263752353499690, 1514.225267046429963, 194.0679338807670149 ) ) ;
#109432=CARTESIAN_POINT ( 'NONE',  ( 0.01126491619350150110, 1516.939530130779985, 216.0663127125970107 ) ) ;
#109433=CARTESIAN_POINT ( 'NONE',  ( -8.071183553683329848, 1511.586636681201526, 212.7277961325115143 ) ) ;
#109439=CARTESIAN_POINT ( 'NONE',  ( -5.011678876155000850, 1516.989560013210166, 205.8658785457569991 ) ) ;
#109441=CARTESIAN_POINT ( 'NONE',  ( 7.724874613184999461, 1517.139320148880188, 209.8621665372610039 ) ) ;
#109444=CARTESIAN_POINT ( 'NONE',  ( 6.560424596724999446, 1512.053281741910041, 217.7862930670369792 ) ) ;
#109453=CARTESIAN_POINT ( 'NONE',  ( 6.559798056295000457, 1516.987478262539980, 213.7368632980669929 ) ) ;
#109458=CARTESIAN_POINT ( 'NONE',  ( 0.01012488564660149991, 1516.989863902050047, 210.2497743036369968 ) ) ;
#109471=CARTESIAN_POINT ( 'NONE',  ( 11.12931921223499998, 1512.151624459629829, 224.9062103328670048 ) ) ;
#109472=CARTESIAN_POINT ( 'NONE',  ( -3.454172653555000139, 1517.122088787240045, 216.8462693643270143 ) ) ;
#109477=CARTESIAN_POINT ( 'NONE',  ( 1.124289655455000148, 1517.184063036290127, 202.5579304082170040 ) ) ;
#109551=CARTESIAN_POINT ( 'NONE',  ( 6.563254890855000134, 1517.139039350860003, 211.6051684241269868 ) ) ;
#109554=CARTESIAN_POINT ( 'NONE',  ( 2.492130623175000448, 1516.778761582560037, 212.5675310476169955 ) ) ;
#109562=CARTESIAN_POINT ( 'NONE',  ( -3.455378015385000001, 1516.627618683580067, 202.1863880069169852 ) ) ;
#109576=CARTESIAN_POINT ( 'NONE',  ( -4.608021707265000266, 1516.660388280709867, 210.8351633799069873 ) ) ;
#109581=CARTESIAN_POINT ( 'NONE',  ( -1.136814071995000175, 1516.854133554269993, 206.8377924607469822 ) ) ;
#109585=( BOUNDED_CURVE ( )  B_SPLINE_CURVE ( 3, ( #34211, #45398, #17939, #632 ),
 .UNSPECIFIED., .F., .T. ) 
 B_SPLINE_CURVE_WITH_KNOTS ( ( 4, 4 ),
 ( 5.097274796035865307, 5.883015582179621283 ),
 .UNSPECIFIED. ) 
 CURVE ( )  GEOMETRIC_REPRESENTATION_ITEM ( )  RATIONAL_B_SPLINE_CURVE ( ( 1.000000000000000000, 0.9492093072870055881, 0.9492093072870055881, 1.000000000000000000 ) ) 
 REPRESENTATION_ITEM ( '' )  );
#109597=CARTESIAN_POINT ( 'NONE',  ( 3.264778779384999829, 1516.727068157269969, 214.1190961241369735 ) ) ;
#109599=FACE_OUTER_BOUND ( 'NONE', #90548, .T. ) ;
#109600=CARTESIAN_POINT ( 'NONE',  ( 2.486474742745000022, 1516.560253536979872, 216.0557253731069807 ) ) ;
#109625=DIRECTION ( 'NONE',  ( -1.000000000000000000, 0.000000000000000000, 0.000000000000000000 ) ) ;
#109631=DIRECTION ( 'NONE',  ( 0.000000000000000000, -1.000000000000000000, 6.123233995736769734E-17 ) ) ;
#109668=CARTESIAN_POINT ( 'NONE',  ( -7.546131077396060149, 1510.764648358900104, 214.9767338929050027 ) ) ;
#109673=EDGE_CURVE ( 'NONE', #1894, #60389, #42797, .T. ) ;
#109674=CARTESIAN_POINT ( 'NONE',  ( 7.713648834184999359, 1516.710624944440042, 208.3691743819339877 ) ) ;
#109678=ADVANCED_FACE ( 'NONE', ( #22924 ), #5606, .T. ) ;
#109706=CARTESIAN_POINT ( 'NONE',  ( -3.822978263369920082, 1508.729442836390035, 204.5649349435400097 ) ) ;
#109708=CARTESIAN_POINT ( 'NONE',  ( 4.998515157294999511, 1516.787536375099990, 205.0819486540370065 ) ) ;
#109711=CARTESIAN_POINT ( 'NONE',  ( 15.26795440090729983, 1513.114148093550057, 195.0970705441609994 ) ) ;
#109728=ORIENTED_EDGE ( 'NONE', *, *, #78018, .T. ) ;
#109735=CARTESIAN_POINT ( 'NONE',  ( 10.25304830813499990, 1513.301704408390151, 203.8185450922669872 ) ) ;
#109753=LINE ( 'NONE', #33031, #34313 ) ;
#109796=CYLINDRICAL_SURFACE ( 'NONE', #21291, 0.4999999999999449329 ) ;
#109799=CARTESIAN_POINT ( 'NONE',  ( -2.613924617009112605, 1516.542698304417627, 201.4125944022433714 ) ) ;
#109805=CARTESIAN_POINT ( 'NONE',  ( -5.787477032644999575, 1517.070197312179971, 206.2521524731670013 ) ) ;
#109815=CARTESIAN_POINT ( 'NONE',  ( -16.50477756776011518, 1512.979858876863773, 220.9284238778866438 ) ) ;
#109819=CARTESIAN_POINT ( 'NONE',  ( 3.268859396054999866, 1516.922519270759949, 211.5998327024669834 ) ) ;
#109849=CARTESIAN_POINT ( 'NONE',  ( -6.942344729965000738, 1516.810037859429940, 201.4055938791270250 ) ) ;
#109850=CARTESIAN_POINT ( 'NONE',  ( -7.724874651314999952, 1517.139320148880188, 208.3815253650730028 ) ) ;
#109853=CARTESIAN_POINT ( 'NONE',  ( 4.936023922893961746, 1511.397677005970309, 217.6234439496228958 ) ) ;
#109868=CARTESIAN_POINT ( 'NONE',  ( -2.485205687335000135, 1517.181921232829836, 216.8478361320569832 ) ) ;
#109872=CARTESIAN_POINT ( 'NONE',  ( 6.947377783174999877, 1517.009964551830080, 213.7374907746170152 ) ) ;
#109889=CARTESIAN_POINT ( 'NONE',  ( -4.042417815834999928, 1516.904492006980036, 205.6736390534169914 ) ) ;
#109905=CYLINDRICAL_SURFACE ( 'NONE', #97976, 2.999999999999995115 ) ;
#109911=CARTESIAN_POINT ( 'NONE',  ( -13.20758818459541395, 1513.543667424516116, 192.3358642619628256 ) ) ;
#109940=CARTESIAN_POINT ( 'NONE',  ( 5.001338628314999646, 1516.911981270829983, 203.3378372969070256 ) ) ;
#109943=CARTESIAN_POINT ( 'NONE',  ( 15.65821248573499780, 1513.518111364920060, 194.4220667106669964 ) ) ;
#109954=VECTOR ( 'NONE', #46209, 1000.000000000000114 ) ;
#109976=CARTESIAN_POINT ( 'NONE',  ( 0.01073129396420149928, 1516.939491476980038, 216.4539099096770087 ) ) ;
#109977=CARTESIAN_POINT ( 'NONE',  ( -7.902635355081809365, 1511.989348023233788, 212.1516878991907333 ) ) ;
#109984=CARTESIAN_POINT ( 'NONE',  ( 1.702405985064999960, 1516.999105586269934, 205.8518611507970206 ) ) ;
#109989=CARTESIAN_POINT ( 'NONE',  ( 7.855403984495000103, 1514.254015528269974, 215.9093767484969817 ) ) ;
#109991=EDGE_LOOP ( 'NONE', ( #20157, #73103, #73211, #32533 ) ) ;
#109997=CARTESIAN_POINT ( 'NONE',  ( -2.285487619494999567, 1517.001127920769704, 213.1661676502270097 ) ) ;
#110000=CARTESIAN_POINT ( 'NONE',  ( -16.66966706706500290, 1516.995662938509895, 194.6788146269670108 ) ) ;
#110001=CARTESIAN_POINT ( 'NONE',  ( -3.251611363945000388, 1516.779243033999819, 211.4202154400570066 ) ) ;
#110006=ORIENTED_EDGE ( 'NONE', *, *, #40792, .T. ) ;
#110015=CARTESIAN_POINT ( 'NONE',  ( -5.779627092215000594, 1516.977993847330026, 216.8424961055369806 ) ) ;
#110020=CARTESIAN_POINT ( 'NONE',  ( 4.033653264325000265, 1517.028034847769959, 202.5611037067669997 ) ) ;
#110040=CARTESIAN_POINT ( 'NONE',  ( -3.803002609304670045, 1508.880967335730247, 213.6144902421019935 ) ) ;
#110052=CARTESIAN_POINT ( 'NONE',  ( 2.325731103684999912, 1511.751588929339960, 216.7056378762670192 ) ) ;
#110053=EDGE_LOOP ( 'NONE', ( #36279, #31286, #38096, #45556, #77654, #57388, #43380, #6280, #22783 ) ) ;
#110059=CARTESIAN_POINT ( 'NONE',  ( 6.149909982967501243, 1516.731221219415374, 204.8276256237976440 ) ) ;
#110073=ORIENTED_EDGE ( 'NONE', *, *, #65043, .T. ) ;
#110085=CARTESIAN_POINT ( 'NONE',  ( 0.000000000000000000, 0.000000000000000000, 0.000000000000000000 ) ) ;
#110097=CARTESIAN_POINT ( 'NONE',  ( -3.447264387095000160, 1516.858765657450249, 212.5828932618570093 ) ) ;
#110103=CARTESIAN_POINT ( 'NONE',  ( 7.714371502985000184, 1516.738222552470233, 203.3422428319769892 ) ) ;
#110119=CARTESIAN_POINT ( 'NONE',  ( 1.717084711415000076, 1516.819260244609950, 211.5980165671369946 ) ) ;
#110124=CARTESIAN_POINT ( 'NONE',  ( -7.337297350114999617, 1517.135701590510052, 208.3821536943570152 ) ) ;
#110129=ORIENTED_EDGE ( 'NONE', *, *, #38046, .F. ) ;
#110138=CARTESIAN_POINT ( 'NONE',  ( -2.480813923114999930, 1517.051603658920158, 214.1347848340070072 ) ) ;
#110141=CARTESIAN_POINT ( 'NONE',  ( -4.615017365965000451, 1516.987478262539980, 215.6816440265270103 ) ) ;
#110142=ORIENTED_EDGE ( 'NONE', *, *, #65451, .F. ) ;
#110170=DIRECTION ( 'NONE',  ( 0.000000000000000000, 1.000000000000000000, -6.123233995736769734E-17 ) ) ;
#110171=VECTOR ( 'NONE', #51302, 1000.000000000000114 ) ;
#110177=CARTESIAN_POINT ( 'NONE',  ( -14.28619595012664156, 1517.015067828383053, 225.9483486273336155 ) ) ;
#110217=CARTESIAN_POINT ( 'NONE',  ( -2.491655763544999846, 1516.977504706749869, 208.3867361609839861 ) ) ;
#110247=CARTESIAN_POINT ( 'NONE',  ( -4.369720495665090354, 1508.879003890470131, 205.0024468196820067 ) ) ;
#110249=CARTESIAN_POINT ( 'NONE',  ( -2.491188396525000126, 1516.733363207009916, 205.0947945262969938 ) ) ;
#110252=CARTESIAN_POINT ( 'NONE',  ( 15.30266648242040084, 1512.633419863009976, 195.7156704886770342 ) ) ;
#110280=PLANE ( 'NONE',  #106750 ) ;
#110292=DIRECTION ( 'NONE',  ( -1.603425251594204954E-18, 0.000000000000000000, 1.000000000000000000 ) ) ;
#110296=VECTOR ( 'NONE', #43952, 1000.000000000000114 ) ;
#110302=CARTESIAN_POINT ( 'NONE',  ( 0.01327404799950150129, 1516.939877939420057, 212.5773418040870126 ) ) ;
#110340=CARTESIAN_POINT ( 'NONE',  ( 2.714430905872757815, 1517.051704408389924, 201.2325484332300221 ) ) ;
#110346=CARTESIAN_POINT ( 'NONE',  ( 6.934528529765000116, 1516.588006113850042, 206.2478870805069846 ) ) ;
#110356=CARTESIAN_POINT ( 'NONE',  ( -16.77006247923849358, 1513.317537406934207, 221.8555522796357877 ) ) ;
#110360=CARTESIAN_POINT ( 'NONE',  ( -4.995726007844999650, 1516.651306816259876, 211.4173314712770093 ) ) ;
#110369=ORIENTED_EDGE ( 'NONE', *, *, #93993, .T. ) ;
#110390=CARTESIAN_POINT ( 'NONE',  ( 5.003220727074999985, 1516.983995446890049, 202.1750974131470286 ) ) ;
#110391=CARTESIAN_POINT ( 'NONE',  ( -4.037051035714999792, 1516.939819969850078, 209.1350663277499962 ) ) ;
#110395=CARTESIAN_POINT ( 'NONE',  ( 4.551262986272157640, 1511.401878033069579, 217.4960750013443374 ) ) ;
#110409=CARTESIAN_POINT ( 'NONE',  ( -5.371346839171279974, 1516.551188146539971, 218.7599618298110045 ) ) ;
#110414=CARTESIAN_POINT ( 'NONE',  ( -4.115863335914074383, 1509.032014613820593, 204.7576463065119299 ) ) ;
#110415=CARTESIAN_POINT ( 'NONE',  ( 0.4918342890736275841, 1516.791933468850175, 216.8376239430565136 ) ) ;
#110416=CARTESIAN_POINT ( 'NONE',  ( -6.937338783705000012, 1516.706638732659940, 213.7399656364970042 ) ) ;
#110424=EDGE_CURVE ( 'NONE', #7555, #21042, #64450, .T. ) ;
#110428=DIRECTION ( 'NONE',  ( -0.7384854939282339270, 4.128709092058508552E-17, 0.6742693640212139572 ) ) ;
#110437=CARTESIAN_POINT ( 'NONE',  ( -1.715704529104999931, 1516.757508073510053, 205.8704515699670026 ) ) ;
#110460=CARTESIAN_POINT ( 'NONE',  ( -14.86632106490745109, 1514.624316683434927, 192.9203402940289038 ) ) ;
#110477=CARTESIAN_POINT ( 'NONE',  ( 10.96015508933500016, 1512.830284628050094, 225.0317485278669949 ) ) ;
#110478=CARTESIAN_POINT ( 'NONE',  ( 14.44303130513500122, 1516.995662938509895, 192.4521789031669812 ) ) ;
#110485=CARTESIAN_POINT ( 'NONE',  ( 4.613762356885000138, 1516.939574742129935, 203.3372076122869885 ) ) ;
#110512=CARTESIAN_POINT ( 'NONE',  ( 7.645353494405000561, 1513.311928781869938, 201.7433401170069942 ) ) ;
#110521=CARTESIAN_POINT ( 'NONE',  ( -1.125509888415000104, 1517.203017563489766, 216.4609531728469847 ) ) ;
#110522=CARTESIAN_POINT ( 'NONE',  ( -7.948115392449770944, 1511.813433987433200, 212.3186854298990340 ) ) ;
#110527=CARTESIAN_POINT ( 'NONE',  ( -7.337793750624999944, 1517.145312756229941, 206.2496372219370073 ) ) ;
#110532=CARTESIAN_POINT ( 'NONE',  ( 7.466890166705000276, 1513.600111798359876, 215.7706967346870215 ) ) ;
#110541=AXIS2_PLACEMENT_3D ( 'NONE', #92977, #24643, #57761 ) ;
#110542=CARTESIAN_POINT ( 'NONE',  ( -7.714371541114999786, 1516.738222552470233, 214.9014490703569891 ) ) ;
#110547=CARTESIAN_POINT ( 'NONE',  ( 7.512750234783659664, 1509.038617475689989, 214.6350457605470012 ) ) ;
#110548=CARTESIAN_POINT ( 'NONE',  ( 5.013274961385000061, 1517.068517094990057, 211.4089302402969963 ) ) ;
#110558=CARTESIAN_POINT ( 'NONE',  ( -7.588802720235000798, 1511.942942747529969, 211.3806715220270007 ) ) ;
#110562=CARTESIAN_POINT ( 'NONE',  ( 1.128757561074999805, 1516.608208975040043, 216.8328129478670121 ) ) ;
#110568=CARTESIAN_POINT ( 'NONE',  ( -3.262264688434999726, 1516.633288330999903, 202.5742890007669814 ) ) ;
#110587=CARTESIAN_POINT ( 'NONE',  ( -4.491288185863250071, 1508.884219112060009, 212.6094329811639909 ) ) ;
#110602=EDGE_CURVE ( 'NONE', #51820, #43618, #91629, .T. ) ;
#110627=CARTESIAN_POINT ( 'NONE',  ( 7.548036962157971708, 1510.518062817387090, 203.4501585446919592 ) ) ;
#110638=VERTEX_POINT ( 'NONE', #40674 ) ;
#110642=ORIENTED_EDGE ( 'NONE', *, *, #72053, .T. ) ;
#110645=CARTESIAN_POINT ( 'NONE',  ( -7.712490991114999694, 1516.666407245520077, 213.7387074786470009 ) ) ;
#110650=CARTESIAN_POINT ( 'NONE',  ( 4.613762356885000138, 1516.939574742129935, 203.3372076122869885 ) ) ;
#110656=CARTESIAN_POINT ( 'NONE',  ( -10.96771875528765428, 1512.594959757391052, 193.2043797466445199 ) ) ;
#110663=CARTESIAN_POINT ( 'NONE',  ( -4.026777524084999449, 1516.718889242609976, 211.4189316860469887 ) ) ;
#110668=CARTESIAN_POINT ( 'NONE',  ( 8.652776089875690246, 1511.435001055579960, 203.7363227723449768 ) ) ;
#110669=CARTESIAN_POINT ( 'NONE',  ( -6.949703372784999722, 1517.130100026000036, 208.3827239650380250 ) ) ;
#110670=EDGE_LOOP ( 'NONE', ( #90597, #3350, #28724, #2870 ) ) ;
#110686=CARTESIAN_POINT ( 'NONE',  ( 2.295485501044999932, 1516.651306816259876, 214.1175719399469983 ) ) ;
#110690=CARTESIAN_POINT ( 'NONE',  ( -4.616272334694999202, 1517.030858226499959, 216.4568033268070053 ) ) ;
#110691=VERTEX_POINT ( 'NONE', #108992 ) ;
#110728=ADVANCED_FACE ( 'NONE', ( #33360, #51847 ), #17646, .F. ) ;
#110749=CARTESIAN_POINT ( 'NONE',  ( -7.404094510329910506, 1512.905891558379153, 200.7965695454380750 ) ) ;
#110773=CARTESIAN_POINT ( 'NONE',  ( 1.704170714124999986, 1516.927039499179955, 208.3639196453299860 ) ) ;
#110782=CARTESIAN_POINT ( 'NONE',  ( -15.25249362911780082, 1513.170547669029929, 223.2087981395630152 ) ) ;
#110802=CARTESIAN_POINT ( 'NONE',  ( -4.832613814269110186, 1508.551704408389924, 205.6342607178579840 ) ) ;
#110804=CARTESIAN_POINT ( 'NONE',  ( 4.609673241434999902, 1516.754149861460064, 205.8564388142570181 ) ) ;
ENDSEC;
END-ISO-10303-21;
